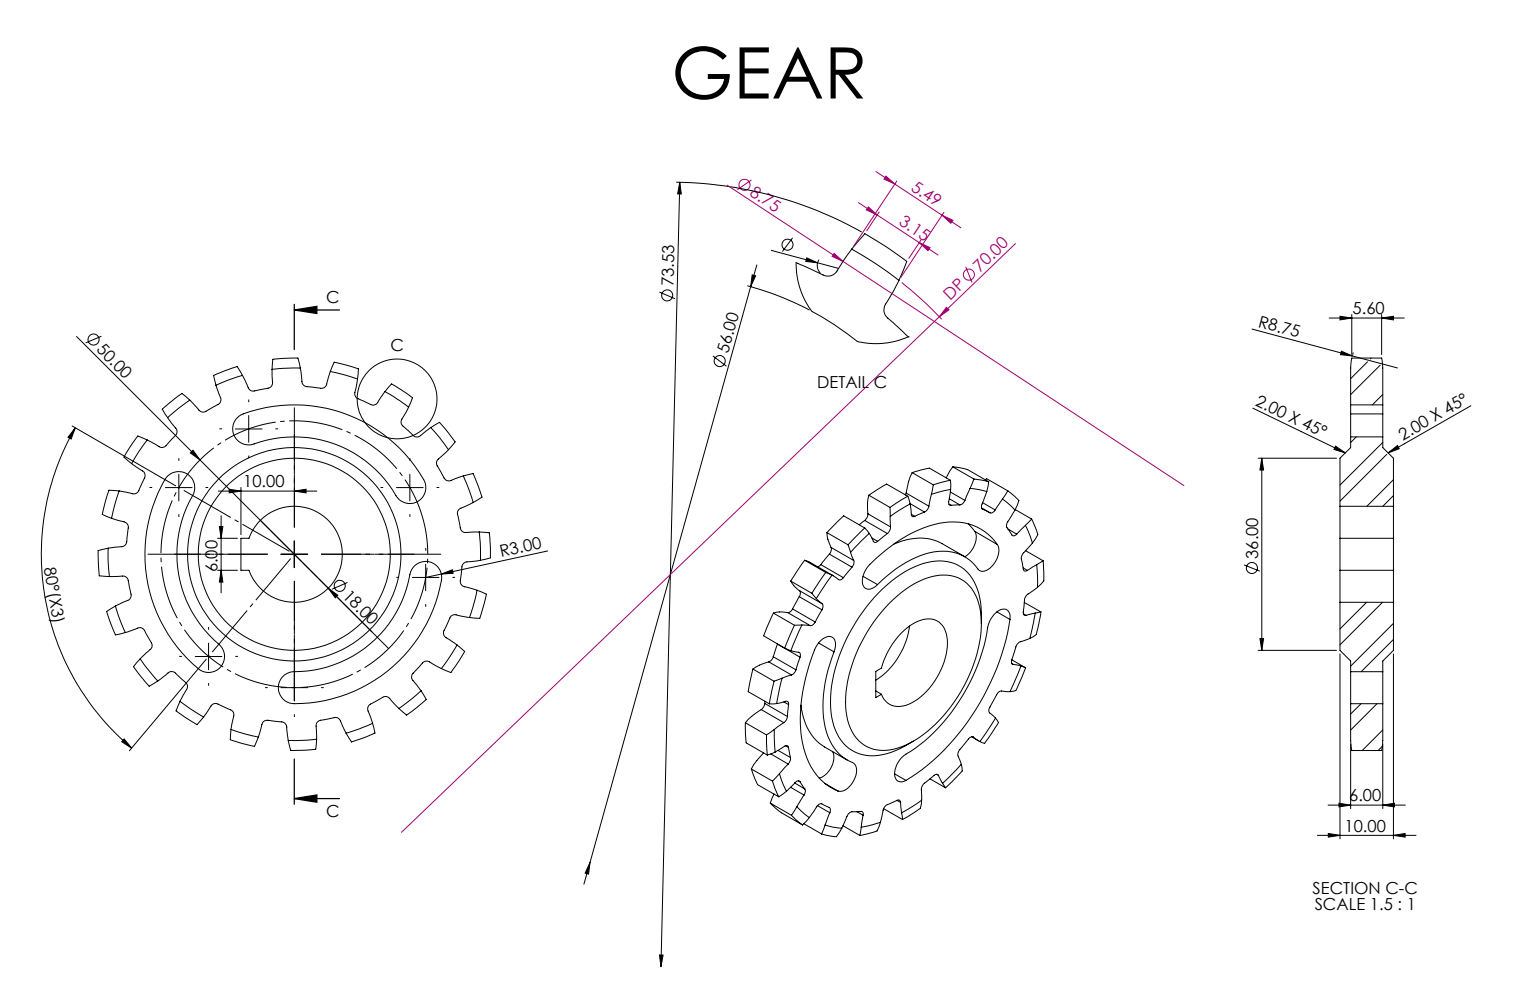
ISO-10303-21;
HEADER;
FILE_DESCRIPTION (('STEP AP214'),
    '1' );
FILE_NAME ('GEAR.step',
    '2026-10-24T00:51:42',
    ( '' ),
    ( '' ),
    'SwSTEP 2.0',
    'SolidWorks 2025',
    '' );
FILE_SCHEMA (( 'AUTOMOTIVE_DESIGN' ));
ENDSEC;

DATA;
#2=DIRECTION ( 'NONE',  ( -1.000000000000000000, 0.000000000000000000, 0.000000000000000000 ) ) ;
#3=EDGE_CURVE ( 'NONE', #16867, #19408, #6040, .T. ) ;
#4=CIRCLE ( 'NONE', #2943, 3.000000000000002665 ) ;
#5=ORIENTED_EDGE ( 'NONE', *, *, #17834, .T. ) ;
#10=CYLINDRICAL_SURFACE ( 'NONE', #2581, 1.000000000000000888 ) ;
#12=DIRECTION ( 'NONE',  ( -6.505213034913038160E-19, -3.903127820947822896E-18, -1.000000000000000000 ) ) ;
#23=ORIENTED_EDGE ( 'NONE', *, *, #6487, .T. ) ;
#24=DIRECTION ( 'NONE',  ( -6.505213034913038160E-19, -3.903127820947822896E-18, -1.000000000000000000 ) ) ;
#29=CARTESIAN_POINT ( 'NONE',  ( -36.39375341857508062, -7.980461308160102796, -6.999999999999985789 ) ) ;
#31=VERTEX_POINT ( 'NONE', #2518 ) ;
#35=ORIENTED_EDGE ( 'NONE', *, *, #15224, .F. ) ;
#41=DIRECTION ( 'NONE',  ( 6.505213034913038160E-19, 3.903127820947822896E-18, 1.000000000000000000 ) ) ;
#43=VERTEX_POINT ( 'NONE', #2740 ) ;
#45=ORIENTED_EDGE ( 'NONE', *, *, #21489, .F. ) ;
#48=DIRECTION ( 'NONE',  ( -1.000000000000000000, -1.208970125616063644E-17, 0.000000000000000000 ) ) ;
#49=ADVANCED_FACE ( 'NONE', ( #14857 ), #21880, .F. ) ;
#61=CARTESIAN_POINT ( 'NONE',  ( -24.43377932785584505, 26.64693883069154623, -2.933296326616394278 ) ) ;
#66=VERTEX_POINT ( 'NONE', #2856 ) ;
#68=CARTESIAN_POINT ( 'NONE',  ( -6.742883674876493316, -34.24928931925791176, -2.999999999999975131 ) ) ;
#69=EDGE_CURVE ( 'NONE', #16039, #14303, #1275, .T. ) ;
#72=DIRECTION ( 'NONE',  ( -1.000000000000000000, 0.000000000000000000, 0.000000000000000000 ) ) ;
#73=EDGE_CURVE ( 'NONE', #8231, #15027, #14429, .T. ) ;
#75=CARTESIAN_POINT ( 'NONE',  ( -21.65063509461097269, 12.49999999999990052, -5.000000000000004441 ) ) ;
#79=ADVANCED_FACE ( 'NONE', ( #15536 ), #15524, .T. ) ;
#80=ORIENTED_EDGE ( 'NONE', *, *, #1374, .F. ) ;
#81=ORIENTED_EDGE ( 'NONE', *, *, #16043, .F. ) ;
#85=CIRCLE ( 'NONE', #13966, 31.50000000000000711 ) ;
#94=CARTESIAN_POINT ( 'NONE',  ( 2.775557561562891351E-14, -2.775557561562891351E-14, 2.999999999999999112 ) ) ;
#100=CARTESIAN_POINT ( 'NONE',  ( -22.28024240313497728, -22.26748298433262008, 3.000000000000023537 ) ) ;
#101=CARTESIAN_POINT ( 'NONE',  ( 27.01645732367885699, 17.86915608785655252, -2.999999999999971578 ) ) ;
#102=AXIS2_PLACEMENT_3D ( 'NONE', #16431, #14697, #2342 ) ;
#103=EDGE_CURVE ( 'NONE', #20053, #16550, #22141, .T. ) ;
#104=VERTEX_POINT ( 'NONE', #2968 ) ;
#109=AXIS2_PLACEMENT_3D ( 'NONE', #8322, #11535, #18749 ) ;
#111=B_SPLINE_CURVE_WITH_KNOTS ( 'NONE', 3,
 ( #17365, #18873, #3301, #3063 ),
 .UNSPECIFIED., .F., .F.,
 ( 4, 4 ),
 ( 0.001893031756885769868, 0.003808480026564024790 ),
 .UNSPECIFIED. ) ;
#115=ORIENTED_EDGE ( 'NONE', *, *, #21368, .T. ) ;
#116=DIRECTION ( 'NONE',  ( 6.505213034913038160E-19, 3.903127820947822896E-18, 1.000000000000000000 ) ) ;
#119=DIRECTION ( 'NONE',  ( -6.505213034913038160E-19, -3.903127820947822896E-18, -1.000000000000000000 ) ) ;
#127=CARTESIAN_POINT ( 'NONE',  ( 4.177897941877304788, -34.13396246814587442, -2.999999999999999112 ) ) ;
#128=CARTESIAN_POINT ( 'NONE',  ( -31.11077005834418685, 4.936596639065066405, 2.999999999999995559 ) ) ;
#129=AXIS2_PLACEMENT_3D ( 'NONE', #9904, #8084, #22058 ) ;
#132=ORIENTED_EDGE ( 'NONE', *, *, #8958, .T. ) ;
#143=ORIENTED_EDGE ( 'NONE', *, *, #2467, .F. ) ;
#144=DIRECTION ( 'NONE',  ( 6.505213034913038160E-19, 3.903127820947822896E-18, 1.000000000000000000 ) ) ;
#148=ORIENTED_EDGE ( 'NONE', *, *, #5497, .F. ) ;
#161=ORIENTED_EDGE ( 'NONE', *, *, #622, .T. ) ;
#162=ORIENTED_EDGE ( 'NONE', *, *, #20424, .T. ) ;
#163=EDGE_CURVE ( 'NONE', #12184, #10164, #18107, .T. ) ;
#165=CARTESIAN_POINT ( 'NONE',  ( -32.75570538720762670, 15.02862401740784293, -2.999999999999995559 ) ) ;
#167=CARTESIAN_POINT ( 'NONE',  ( 3.330669073875469621E-13, -1.110223024625156540E-13, -2.999999999999971578 ) ) ;
#173=AXIS2_PLACEMENT_3D ( 'NONE', #16930, #17152, #13241 ) ;
#175=CARTESIAN_POINT ( 'NONE',  ( 2.220446049250313081E-13, 2.775557561562891351E-14, -2.800654218530485018 ) ) ;
#182=EDGE_CURVE ( 'NONE', #4097, #21371, #18465, .T. ) ;
#188=ORIENTED_EDGE ( 'NONE', *, *, #1082, .F. ) ;
#192=EDGE_LOOP ( 'NONE', ( #22045, #625, #16460, #5308 ) ) ;
#195=DIRECTION ( 'NONE',  ( 6.505213034913038160E-19, 3.903127820947822896E-18, 1.000000000000000000 ) ) ;
#203=AXIS2_PLACEMENT_3D ( 'NONE', #6824, #20803, #5115 ) ;
#204=ORIENTED_EDGE ( 'NONE', *, *, #20103, .T. ) ;
#206=CARTESIAN_POINT ( 'NONE',  ( -11.35354668330701422, -30.33632613426187774, 2.999999999999999112 ) ) ;
#209=CARTESIAN_POINT ( 'NONE',  ( -26.64365646977275048, -17.09029715894938661, -6.999999999999950262 ) ) ;
#211=CIRCLE ( 'NONE', #1322, 34.90673715956759082 ) ;
#214=DIRECTION ( 'NONE',  ( 6.505213034913038160E-19, 3.903127820947822896E-18, 1.000000000000000000 ) ) ;
#217=AXIS2_PLACEMENT_3D ( 'NONE', #4678, #12107, #11654 ) ;
#218=EDGE_CURVE ( 'NONE', #13519, #1842, #5991, .T. ) ;
#228=CARTESIAN_POINT ( 'NONE',  ( 11.93772187171674126, 33.46652738560661788, -3.000000000000018208 ) ) ;
#230=DIRECTION ( 'NONE',  ( 1.000000000000000000, 0.000000000000000000, 0.000000000000000000 ) ) ;
#236=FACE_OUTER_BOUND ( 'NONE', #19875, .T. ) ;
#237=ORIENTED_EDGE ( 'NONE', *, *, #15109, .F. ) ;
#238=DIRECTION ( 'NONE',  ( -1.000000000000000000, 0.000000000000000000, 0.000000000000000000 ) ) ;
#247=ORIENTED_EDGE ( 'NONE', *, *, #15444, .T. ) ;
#251=EDGE_CURVE ( 'NONE', #17561, #8959, #16232, .T. ) ;
#258=DIRECTION ( 'NONE',  ( -1.000000000000000000, -1.208970125616081209E-17, 0.000000000000000000 ) ) ;
#260=VERTEX_POINT ( 'NONE', #22683 ) ;
#263=DIRECTION ( 'NONE',  ( 1.000000000000000000, 0.000000000000000000, 0.000000000000000000 ) ) ;
#271=CARTESIAN_POINT ( 'NONE',  ( -12.00937115242646591, -34.74700806321101254, 2.800654218530512551 ) ) ;
#275=CARTESIAN_POINT ( 'NONE',  ( 17.79229176513301525, 31.47226199422865278, -2.933296326616372074 ) ) ;
#278=CARTESIAN_POINT ( 'NONE',  ( -25.58633464742629471, -23.74488952252781715, -2.999999999999975131 ) ) ;
#281=ORIENTED_EDGE ( 'NONE', *, *, #17376, .F. ) ;
#290=DIRECTION ( 'NONE',  ( 1.000000000000000000, 0.000000000000000000, 0.000000000000000000 ) ) ;
#294=CIRCLE ( 'NONE', #3228, 34.90673715956759082 ) ;
#295=VERTEX_POINT ( 'NONE', #13926 ) ;
#299=FACE_OUTER_BOUND ( 'NONE', #1043, .T. ) ;
#302=FACE_OUTER_BOUND ( 'NONE', #6391, .T. ) ;
#303=EDGE_CURVE ( 'NONE', #11367, #19446, #9654, .T. ) ;
#304=VECTOR ( 'NONE', #3939, 1000.000000000000000 ) ;
#309=AXIS2_PLACEMENT_3D ( 'NONE', #21426, #5731, #12703 ) ;
#312=VERTEX_POINT ( 'NONE', #7642 ) ;
#315=AXIS2_PLACEMENT_3D ( 'NONE', #10190, #17183, #1262 ) ;
#318=CARTESIAN_POINT ( 'NONE',  ( -26.50842683089743446, 24.41514043009193458, -2.999999999999975131 ) ) ;
#320=EDGE_CURVE ( 'NONE', #13797, #13818, #18394, .T. ) ;
#326=EDGE_LOOP ( 'NONE', ( #11952, #8295, #15497, #872 ) ) ;
#327=CARTESIAN_POINT ( 'NONE',  ( 5.551115123125782702E-14, -1.387778780781445676E-13, -5.749999999999949374 ) ) ;
#331=EDGE_CURVE ( 'NONE', #8378, #6859, #4945, .T. ) ;
#332=DIRECTION ( 'NONE',  ( 6.505213034913038160E-19, 3.903127820947822896E-18, 1.000000000000000000 ) ) ;
#333=ORIENTED_EDGE ( 'NONE', *, *, #2752, .T. ) ;
#335=DIRECTION ( 'NONE',  ( 6.505213034913038160E-19, 3.903127820947822896E-18, 1.000000000000000000 ) ) ;
#338=ORIENTED_EDGE ( 'NONE', *, *, #3032, .F. ) ;
#344=ADVANCED_FACE ( 'NONE', ( #7407, #531 ), #16341, .T. ) ;
#345=DIRECTION ( 'NONE',  ( 6.505213034913038160E-19, 3.903127820947822896E-18, 1.000000000000000000 ) ) ;
#346=ORIENTED_EDGE ( 'NONE', *, *, #17247, .F. ) ;
#352=DIRECTION ( 'NONE',  ( 1.000000000000000000, 0.000000000000000000, 0.000000000000000000 ) ) ;
#361=DIRECTION ( 'NONE',  ( -1.000000000000000000, -1.208970125616060717E-17, 0.000000000000000000 ) ) ;
#363=CIRCLE ( 'NONE', #12085, 1.000000000000000888 ) ;
#365=ORIENTED_EDGE ( 'NONE', *, *, #6652, .F. ) ;
#366=B_SPLINE_CURVE_WITH_KNOTS ( 'NONE', 3,
 ( #12902, #16119, #9147, #665 ),
 .UNSPECIFIED., .F., .F.,
 ( 4, 4 ),
 ( 0.001893031756885595529, 0.003808480026563915502 ),
 .UNSPECIFIED. ) ;
#372=AXIS2_PLACEMENT_3D ( 'NONE', #19827, #18095, #3326 ) ;
#375=ORIENTED_EDGE ( 'NONE', *, *, #11869, .T. ) ;
#376=DIRECTION ( 'NONE',  ( 1.000000000000000000, 0.000000000000000000, 0.000000000000000000 ) ) ;
#377=DIRECTION ( 'NONE',  ( 6.505213034913038160E-19, 3.903127820947822896E-18, 1.000000000000000000 ) ) ;
#378=ORIENTED_EDGE ( 'NONE', *, *, #15742, .T. ) ;
#381=CARTESIAN_POINT ( 'NONE',  ( 21.69517388068236841, 28.13960001536964128, -3.000000000000001776 ) ) ;
#382=DIRECTION ( 'NONE',  ( -6.505213034913038160E-19, -3.903127820947822896E-18, -1.000000000000000000 ) ) ;
#384=VERTEX_POINT ( 'NONE', #9359 ) ;
#396=ORIENTED_EDGE ( 'NONE', *, *, #11487, .T. ) ;
#399=ORIENTED_EDGE ( 'NONE', *, *, #73, .F. ) ;
#402=CARTESIAN_POINT ( 'NONE',  ( -35.79662727779878395, 4.171001175319294596, 3.000000000000006217 ) ) ;
#406=VECTOR ( 'NONE', #10198, 1000.000000000000000 ) ;
#410=LINE ( 'NONE', #7295, #19704 ) ;
#411=CARTESIAN_POINT ( 'NONE',  ( 2.775557561562891351E-14, 2.775557561562891351E-14, 5.750000000000001776 ) ) ;
#415=DIRECTION ( 'NONE',  ( 1.000000000000000000, 0.000000000000000000, 0.000000000000000000 ) ) ;
#417=B_SPLINE_CURVE_WITH_KNOTS ( 'NONE', 3,
 ( #9345, #17934, #21264, #14708 ),
 .UNSPECIFIED., .F., .F.,
 ( 4, 4 ),
 ( 9.545285770746368752E-07, 0.001900595205834774504 ),
 .UNSPECIFIED. ) ;
#427=LINE ( 'NONE', #14393, #10875 ) ;
#429=FACE_OUTER_BOUND ( 'NONE', #19761, .T. ) ;
#430=ADVANCED_FACE ( 'NONE', ( #15166 ), #13332, .T. ) ;
#443=EDGE_CURVE ( 'NONE', #2350, #18209, #20357, .T. ) ;
#444=ORIENTED_EDGE ( 'NONE', *, *, #19808, .F. ) ;
#445=CARTESIAN_POINT ( 'NONE',  ( -15.12081897056664914, 33.51030287062364721, -2.800654218530457484 ) ) ;
#446=ADVANCED_FACE ( 'NONE', ( #9810 ), #21783, .T. ) ;
#447=ORIENTED_EDGE ( 'NONE', *, *, #13329, .T. ) ;
#448=CARTESIAN_POINT ( 'NONE',  ( -4.170748987303213084, 34.65667543218822999, 3.000000000000002665 ) ) ;
#450=FACE_OUTER_BOUND ( 'NONE', #22695, .T. ) ;
#456=CARTESIAN_POINT ( 'NONE',  ( 2.775557561562891351E-14, -2.775557561562891351E-14, 2.999999999999999112 ) ) ;
#458=AXIS2_PLACEMENT_3D ( 'NONE', #18438, #22003, #1140 ) ;
#461=CARTESIAN_POINT ( 'NONE',  ( 7.463862311151453710, 35.99819890246943999, -2.800654218530457484 ) ) ;
#463=B_SPLINE_CURVE_WITH_KNOTS ( 'NONE', 3,
 ( #3611, #20792, #8757, #8523 ),
 .UNSPECIFIED., .F., .F.,
 ( 4, 4 ),
 ( 9.715086409175039034E-07, 0.001929643240672277446 ),
 .UNSPECIFIED. ) ;
#467=CARTESIAN_POINT ( 'NONE',  ( 31.21605069118074738, 8.646032897228984382, 2.999999999999995559 ) ) ;
#473=EDGE_LOOP ( 'NONE', ( #18170, #2329, #19189, #6844 ) ) ;
#481=CARTESIAN_POINT ( 'NONE',  ( 2.775557561562891351E-14, -2.775557561562891351E-14, 2.999999999999999112 ) ) ;
#483=CARTESIAN_POINT ( 'NONE',  ( -31.92986134326225667, 18.22261011550274645, 2.800654218530509443 ) ) ;
#489=ORIENTED_EDGE ( 'NONE', *, *, #9326, .F. ) ;
#492=DIRECTION ( 'NONE',  ( -1.000000000000000000, -1.052817288873011806E-14, 0.000000000000000000 ) ) ;
#502=AXIS2_PLACEMENT_3D ( 'NONE', #8254, #6205, #22245 ) ;
#505=ORIENTED_EDGE ( 'NONE', *, *, #18677, .F. ) ;
#509=ORIENTED_EDGE ( 'NONE', *, *, #13212, .T. ) ;
#519=EDGE_CURVE ( 'NONE', #5408, #3873, #7462, .T. ) ;
#520=EDGE_CURVE ( 'NONE', #4189, #4363, #18750, .T. ) ;
#525=DIRECTION ( 'NONE',  ( -1.000000000000000000, 0.000000000000000000, 0.000000000000000000 ) ) ;
#527=EDGE_CURVE ( 'NONE', #21131, #15970, #924, .T. ) ;
#531=FACE_OUTER_BOUND ( 'NONE', #18877, .T. ) ;
#541=AXIS2_PLACEMENT_3D ( 'NONE', #5026, #15537, #8566 ) ;
#556=PLANE ( 'NONE',  #2500 ) ;
#557=CIRCLE ( 'NONE', #3135, 31.50000000000000711 ) ;
#559=DIRECTION ( 'NONE',  ( 1.000000000000000000, 0.000000000000000000, 0.000000000000000000 ) ) ;
#561=EDGE_CURVE ( 'NONE', #19756, #19564, #12445, .T. ) ;
#571=CYLINDRICAL_SURFACE ( 'NONE', #12438, 36.76383501243555685 ) ;
#573=VERTEX_POINT ( 'NONE', #3286 ) ;
#581=DIRECTION ( 'NONE',  ( -6.505213034913038160E-19, -3.903127820947822896E-18, -1.000000000000000000 ) ) ;
#583=DIRECTION ( 'NONE',  ( 6.505213034913038160E-19, 3.903127820947822896E-18, 1.000000000000000000 ) ) ;
#584=DIRECTION ( 'NONE',  ( 1.000000000000000000, 0.000000000000000000, 0.000000000000000000 ) ) ;
#586=VERTEX_POINT ( 'NONE', #3393 ) ;
#587=DIRECTION ( 'NONE',  ( 1.000000000000000000, 0.000000000000000000, 0.000000000000000000 ) ) ;
#589=AXIS2_PLACEMENT_3D ( 'NONE', #14454, #144, #14110 ) ;
#591=CIRCLE ( 'NONE', #19618, 34.90673715956759082 ) ;
#600=CARTESIAN_POINT ( 'NONE',  ( 32.09841355225995585, -5.093313992686393732, -2.999999999999971578 ) ) ;
#601=DIRECTION ( 'NONE',  ( -6.505213034913038160E-19, -3.903127820947822896E-18, -1.000000000000000000 ) ) ;
#603=ORIENTED_EDGE ( 'NONE', *, *, #21489, .T. ) ;
#611=ORIENTED_EDGE ( 'NONE', *, *, #4266, .F. ) ;
#612=EDGE_CURVE ( 'NONE', #4064, #19773, #10257, .T. ) ;
#618=ORIENTED_EDGE ( 'NONE', *, *, #4093, .F. ) ;
#622=EDGE_CURVE ( 'NONE', #14783, #19446, #2359, .T. ) ;
#625=ORIENTED_EDGE ( 'NONE', *, *, #14576, .T. ) ;
#632=ORIENTED_EDGE ( 'NONE', *, *, #6395, .T. ) ;
#633=CARTESIAN_POINT ( 'NONE',  ( 21.00948735876884044, 24.79619811426203668, -6.999999999999950262 ) ) ;
#638=EDGE_LOOP ( 'NONE', ( #7057, #3498, #13428, #19774 ) ) ;
#648=AXIS2_PLACEMENT_3D ( 'NONE', #22157, #18941, #22389 ) ;
#649=DIRECTION ( 'NONE',  ( 1.000000000000000000, 0.000000000000000000, 0.000000000000000000 ) ) ;
#650=EDGE_CURVE ( 'NONE', #2517, #14456, #15130, .T. ) ;
#655=ADVANCED_FACE ( 'NONE', ( #1789 ), #15745, .T. ) ;
#657=EDGE_LOOP ( 'NONE', ( #17524, #9089, #7383, #7095 ) ) ;
#660=AXIS2_PLACEMENT_3D ( 'NONE', #764, #11299, #10833 ) ;
#662=FACE_OUTER_BOUND ( 'NONE', #3144, .T. ) ;
#665=CARTESIAN_POINT ( 'NONE',  ( -10.70799354677358295, 35.16985127952384715, -2.800654218530457484 ) ) ;
#667=VECTOR ( 'NONE', #15836, 1000.000000000000000 ) ;
#673=DIRECTION ( 'NONE',  ( -6.505213034913038160E-19, -3.903127820947822896E-18, -1.000000000000000000 ) ) ;
#683=AXIS2_PLACEMENT_3D ( 'NONE', #20759, #3350, #19155 ) ;
#684=ORIENTED_EDGE ( 'NONE', *, *, #8709, .F. ) ;
#686=LINE ( 'NONE', #5725, #14759 ) ;
#687=CIRCLE ( 'NONE', #13469, 19.11328065563150957 ) ;
#688=EDGE_CURVE ( 'NONE', #6587, #2221, #21014, .T. ) ;
#689=CARTESIAN_POINT ( 'NONE',  ( -4.153395668489446635, 35.29097153256767427, -3.000000000000005773 ) ) ;
#691=VERTEX_POINT ( 'NONE', #19537 ) ;
#700=CARTESIAN_POINT ( 'NONE',  ( 2.220446049250313081E-13, -8.326672684688674053E-14, 2.800654218530498785 ) ) ;
#706=AXIS2_PLACEMENT_3D ( 'NONE', #726, #7708, #376 ) ;
#710=ADVANCED_FACE ( 'NONE', ( #9559 ), #16194, .F. ) ;
#719=ORIENTED_EDGE ( 'NONE', *, *, #14828, .T. ) ;
#721=DIRECTION ( 'NONE',  ( -1.000000000000000000, -1.208970125616046080E-17, 6.505213034913038160E-19 ) ) ;
#726=CARTESIAN_POINT ( 'NONE',  ( -36.39375341857506641, -7.980461308160019307, 2.999999999999995559 ) ) ;
#728=VERTEX_POINT ( 'NONE', #12980 ) ;
#735=CARTESIAN_POINT ( 'NONE',  ( 3.330669073875469621E-13, -1.110223024625156540E-13, -2.999999999999971578 ) ) ;
#739=DIRECTION ( 'NONE',  ( 6.505213034913038160E-19, 3.903127820947822896E-18, 1.000000000000000000 ) ) ;
#741=ORIENTED_EDGE ( 'NONE', *, *, #20768, .T. ) ;
#743=DIRECTION ( 'NONE',  ( -1.000000000000000000, 0.000000000000000000, 0.000000000000000000 ) ) ;
#744=LINE ( 'NONE', #7724, #8894 ) ;
#746=AXIS2_PLACEMENT_3D ( 'NONE', #2751, #20166, #1139 ) ;
#749=ORIENTED_EDGE ( 'NONE', *, *, #19224, .T. ) ;
#750=ORIENTED_EDGE ( 'NONE', *, *, #2861, .F. ) ;
#754=ORIENTED_EDGE ( 'NONE', *, *, #3, .T. ) ;
#755=CARTESIAN_POINT ( 'NONE',  ( -30.57187188083515750, -7.711478842616581453, -7.000000000000006217 ) ) ;
#756=DIRECTION ( 'NONE',  ( -1.000000000000000000, -1.208970125616060717E-17, 0.000000000000000000 ) ) ;
#758=ORIENTED_EDGE ( 'NONE', *, *, #14920, .T. ) ;
#763=LINE ( 'NONE', #21503, #19035 ) ;
#764=CARTESIAN_POINT ( 'NONE',  ( 2.775557561562891351E-14, -2.775557561562891351E-14, 2.999999999999999112 ) ) ;
#766=DIRECTION ( 'NONE',  ( 6.505213034913038160E-19, 3.903127820947822896E-18, 1.000000000000000000 ) ) ;
#767=VERTEX_POINT ( 'NONE', #11155 ) ;
#768=VERTEX_POINT ( 'NONE', #14807 ) ;
#781=CARTESIAN_POINT ( 'NONE',  ( 3.330669073875469621E-13, -1.110223024625156540E-13, -2.999999999999971578 ) ) ;
#784=DIRECTION ( 'NONE',  ( 6.505213034913038160E-19, 3.903127820947822896E-18, 1.000000000000000000 ) ) ;
#794=EDGE_CURVE ( 'NONE', #10901, #12610, #2063, .T. ) ;
#795=ORIENTED_EDGE ( 'NONE', *, *, #10962, .F. ) ;
#801=CARTESIAN_POINT ( 'NONE',  ( -31.41239365194187272, 2.347663744114131035, -2.999999999999999112 ) ) ;
#803=DIRECTION ( 'NONE',  ( 1.000000000000000000, 0.000000000000000000, 0.000000000000000000 ) ) ;
#804=DIRECTION ( 'NONE',  ( -6.505213034913038160E-19, -3.903127820947822896E-18, -1.000000000000000000 ) ) ;
#808=CARTESIAN_POINT ( 'NONE',  ( -32.09841355225989901, 5.093313992686310243, -2.999999999999971578 ) ) ;
#811=DIRECTION ( 'NONE',  ( 6.505213034913038160E-19, 3.903127820947822896E-18, 1.000000000000000000 ) ) ;
#817=VERTEX_POINT ( 'NONE', #7327 ) ;
#820=CARTESIAN_POINT ( 'NONE',  ( 10.70799354677390269, -35.16985127952376899, -1.999999999999977573 ) ) ;
#822=AXIS2_PLACEMENT_3D ( 'NONE', #1588, #15211, #10392 ) ;
#824=DIRECTION ( 'NONE',  ( -1.000000000000000000, -1.208970125616062874E-17, 0.000000000000000000 ) ) ;
#827=ORIENTED_EDGE ( 'NONE', *, *, #19139, .F. ) ;
#829=FACE_OUTER_BOUND ( 'NONE', #20164, .T. ) ;
#833=DIRECTION ( 'NONE',  ( 6.505213034913038160E-19, 3.903127820947822896E-18, 1.000000000000000000 ) ) ;
#835=ORIENTED_EDGE ( 'NONE', *, *, #6395, .F. ) ;
#836=CARTESIAN_POINT ( 'NONE',  ( 36.75746821813308429, -0.6841746959067585010, 2.800654218530485018 ) ) ;
#838=EDGE_LOOP ( 'NONE', ( #3738, #12394, #3480, #9059 ) ) ;
#842=EDGE_LOOP ( 'NONE', ( #12632, #21482, #12314, #5111 ) ) ;
#845=DIRECTION ( 'NONE',  ( -1.000000000000000000, 0.000000000000000000, 0.000000000000000000 ) ) ;
#849=ORIENTED_EDGE ( 'NONE', *, *, #20424, .F. ) ;
#852=ORIENTED_EDGE ( 'NONE', *, *, #561, .T. ) ;
#854=DIRECTION ( 'NONE',  ( 6.505213034913038160E-19, 3.903127820947822896E-18, 1.000000000000000000 ) ) ;
#858=LINE ( 'NONE', #977, #13833 ) ;
#859=DIRECTION ( 'NONE',  ( -1.000000000000000000, 0.000000000000000000, 0.000000000000000000 ) ) ;
#863=DIRECTION ( 'NONE',  ( -6.505213034913038160E-19, -3.903127820947822896E-18, -1.000000000000000000 ) ) ;
#870=CARTESIAN_POINT ( 'NONE',  ( 8.646032897229400049, -31.21605069118077580, -6.999999999999950262 ) ) ;
#872=ORIENTED_EDGE ( 'NONE', *, *, #16600, .F. ) ;
#873=AXIS2_PLACEMENT_3D ( 'NONE', #3321, #3426, #13829 ) ;
#875=AXIS2_PLACEMENT_3D ( 'NONE', #12799, #6284, #13239 ) ;
#877=VERTEX_POINT ( 'NONE', #17322 ) ;
#885=DIRECTION ( 'NONE',  ( -1.000000000000000000, -1.208970125616063644E-17, 0.000000000000000000 ) ) ;
#890=CYLINDRICAL_SURFACE ( 'NONE', #9031, 1.000000000000000888 ) ;
#892=AXIS2_PLACEMENT_3D ( 'NONE', #18524, #18401, #17021 ) ;
#896=DIRECTION ( 'NONE',  ( 6.505213034913038160E-19, 3.903127820947822896E-18, 1.000000000000000000 ) ) ;
#898=ORIENTED_EDGE ( 'NONE', *, *, #4527, .T. ) ;
#899=CARTESIAN_POINT ( 'NONE',  ( 31.88709182564711142, -6.070730550691017413, 3.000000000000023537 ) ) ;
#901=CARTESIAN_POINT ( 'NONE',  ( 13.83143812983114707, -29.36548507648029016, -7.000000000000006217 ) ) ;
#905=CLOSED_SHELL ( 'NONE', ( #8563, #7076, #7929, #5678, #4465, #19150, #22576, #21458, #17712, #22222, #14782, #18419, #10391, #18239, #21785, #15928, #20178, #20226, #22233, #17927, #1863, #20395, #11837, #3599, #19443, #4692, #22628, #3299, #8649, #15514, #16721, #17259, #9019, #446, #1883, #17878, #8627, #15174, #20934, #10317, #17011, #430, #21730, #10433, #7354, #6426, #8274, #6528, #19882, #14280, #5310, #16856, #1353, #21124, #21999, #3977, #3481, #22065, #21190, #19028, #20680, #7463, #4335, #7078, #19523, #6625, #13775, #6600, #79, #8690, #20388, #3896, #2793, #13872, #15714, #5580, #19400, #10512, #8045, #12162, #18996, #15644, #12391, #11699, #344, #4559, #19376, #6148, #16346, #5545, #20631, #5202, #6959, #710, #4050, #13479, #14669, #14161, #1133, #2663, #18798, #4994, #14152, #14115, #16630, #13032, #3733, #10277, #7161, #2695, #3578, #1578, #655, #3354, #22650, #16686, #10847, #4861, #2677, #4727, #8678, #2175, #1764, #21366, #8230, #21822, #11023, #12771, #6554, #3602, #17130, #2598, #18208, #1841, #49, #6063, #16890, #12466, #17199, #15996, #21331, #8768, #2547, #8457, #22021, #6723, #20844, #21569, #17421, #5170, #16899, #4305, #11695, #22112, #22530, #9787, #17969, #8510, #5336, #13785, #10560, #17620, #13789, #1192, #21912, #3155, #19476, #2571, #13649, #2542, #11689, #2092, #18154, #9700, #18616, #5920, #14977, #20262, #5253, #5136, #6203, #12695, #20029, #16570, #21394, #16155, #16800, #21167, #16955, #6364, #9507, #16744, #8591, #19098, #1749, #6842, #21050, #6972, #17155, #19451, #8556 ) ) ;
#907=CARTESIAN_POINT ( 'NONE',  ( 34.74700806321121149, -12.00937115242670039, 2.800654218530512551 ) ) ;
#908=EDGE_CURVE ( 'NONE', #19435, #14442, #4561, .T. ) ;
#909=CARTESIAN_POINT ( 'NONE',  ( -4.025500340002513333, 36.54278193890309012, -2.800654218530457484 ) ) ;
#910=ORIENTED_EDGE ( 'NONE', *, *, #12200, .F. ) ;
#912=DIRECTION ( 'NONE',  ( 6.505213034913038160E-19, 3.903127820947822896E-18, 1.000000000000000000 ) ) ;
#920=CARTESIAN_POINT ( 'NONE',  ( 17.38064605515585725, 30.98879172160187068, 3.000000000000048850 ) ) ;
#921=EDGE_CURVE ( 'NONE', #10690, #11353, #1254, .T. ) ;
#924=CIRCLE ( 'NONE', #17694, 19.11328065563150957 ) ;
#928=VERTEX_POINT ( 'NONE', #1173 ) ;
#934=CIRCLE ( 'NONE', #6414, 36.76383501243555685 ) ;
#936=ORIENTED_EDGE ( 'NONE', *, *, #12946, .T. ) ;
#943=VERTEX_POINT ( 'NONE', #14908 ) ;
#945=CARTESIAN_POINT ( 'NONE',  ( 33.52953626616073279, 9.708269511265299911, -2.999999999999999112 ) ) ;
#953=ORIENTED_EDGE ( 'NONE', *, *, #3177, .F. ) ;
#955=AXIS2_PLACEMENT_3D ( 'NONE', #2451, #833, #9435 ) ;
#956=CARTESIAN_POINT ( 'NONE',  ( -21.05198877411806890, 30.13956425491229396, 2.800654218530481465 ) ) ;
#961=CARTESIAN_POINT ( 'NONE',  ( 22.15900668633799597, 29.33526866242094755, 2.800654218530481465 ) ) ;
#962=CARTESIAN_POINT ( 'NONE',  ( 2.775557561562891351E-14, 2.775557561562891351E-14, 5.750000000000001776 ) ) ;
#969=CIRCLE ( 'NONE', #14843, 1.000000000000000888 ) ;
#975=EDGE_CURVE ( 'NONE', #10281, #6403, #8168, .T. ) ;
#977=CARTESIAN_POINT ( 'NONE',  ( -33.51030287062356194, -15.12081897056691204, -2.000000000000005329 ) ) ;
#980=DIRECTION ( 'NONE',  ( -6.505213034913038160E-19, -3.903127820947822896E-18, -1.000000000000000000 ) ) ;
#986=CARTESIAN_POINT ( 'NONE',  ( -35.91964150878168027, -4.104665049622911788, -2.933296326616361416 ) ) ;
#995=FACE_OUTER_BOUND ( 'NONE', #22560, .T. ) ;
#1002=DIRECTION ( 'NONE',  ( 1.000000000000000000, 1.208970125616053475E-17, 0.000000000000000000 ) ) ;
#1010=DIRECTION ( 'NONE',  ( 1.000000000000000000, 1.208970125616053321E-17, 0.000000000000000000 ) ) ;
#1019=CARTESIAN_POINT ( 'NONE',  ( 37.07861450834818129, -3.656418565264468512, -6.999999999999999112 ) ) ;
#1020=EDGE_CURVE ( 'NONE', #18887, #21019, #14081, .T. ) ;
#1022=DIRECTION ( 'NONE',  ( 6.505213034913038160E-19, 3.903127820947822896E-18, 1.000000000000000000 ) ) ;
#1025=CIRCLE ( 'NONE', #15655, 31.50000000000001421 ) ;
#1028=VECTOR ( 'NONE', #21615, 1000.000000000000000 ) ;
#1029=DIRECTION ( 'NONE',  ( -1.000000000000000000, -1.208970125616060717E-17, 0.000000000000000000 ) ) ;
#1034=DIRECTION ( 'NONE',  ( -1.000000000000000000, -1.208970125616077665E-17, 0.000000000000000000 ) ) ;
#1041=B_SPLINE_CURVE_WITH_KNOTS ( 'NONE', 3,
 ( #15282, #19394, #22410, #15505 ),
 .UNSPECIFIED., .F., .F.,
 ( 4, 4 ),
 ( 0.001893031756885169004, 0.003808480026563660498 ),
 .UNSPECIFIED. ) ;
#1043=EDGE_LOOP ( 'NONE', ( #3805, #13880, #14516, #5311 ) ) ;
#1044=AXIS2_PLACEMENT_3D ( 'NONE', #4036, #2841, #6275 ) ;
#1046=DIRECTION ( 'NONE',  ( 6.505213034913038160E-19, 3.903127820947822896E-18, 1.000000000000000000 ) ) ;
#1047=AXIS2_PLACEMENT_3D ( 'NONE', #633, #15979, #290 ) ;
#1048=AXIS2_PLACEMENT_3D ( 'NONE', #20032, #4338, #1002 ) ;
#1050=ORIENTED_EDGE ( 'NONE', *, *, #320, .T. ) ;
#1051=EDGE_CURVE ( 'NONE', #1297, #18279, #13311, .T. ) ;
#1052=ORIENTED_EDGE ( 'NONE', *, *, #13195, .T. ) ;
#1060=CARTESIAN_POINT ( 'NONE',  ( -5.074925817841801745, 32.10132595304121850, -6.999999999999950262 ) ) ;
#1064=CIRCLE ( 'NONE', #7639, 36.76383501243555685 ) ;
#1066=EDGE_CURVE ( 'NONE', #22056, #12221, #10745, .T. ) ;
#1068=DIRECTION ( 'NONE',  ( 1.000000000000000000, 0.000000000000000000, 0.000000000000000000 ) ) ;
#1072=CARTESIAN_POINT ( 'NONE',  ( 29.36548507648026174, 13.83143812983086995, 3.000000000000023537 ) ) ;
#1073=ORIENTED_EDGE ( 'NONE', *, *, #4590, .T. ) ;
#1076=ORIENTED_EDGE ( 'NONE', *, *, #6843, .F. ) ;
#1080=EDGE_LOOP ( 'NONE', ( #4988, #8993, #12256, #12165, #18775, #10133 ) ) ;
#1081=DIRECTION ( 'NONE',  ( -1.000000000000000000, -1.208970125616081209E-17, 0.000000000000000000 ) ) ;
#1082=EDGE_CURVE ( 'NONE', #8936, #13925, #9174, .T. ) ;
#1086=ORIENTED_EDGE ( 'NONE', *, *, #5522, .F. ) ;
#1087=ORIENTED_EDGE ( 'NONE', *, *, #13548, .F. ) ;
#1088=VERTEX_POINT ( 'NONE', #16387 ) ;
#1089=VERTEX_POINT ( 'NONE', #12592 ) ;
#1093=DIRECTION ( 'NONE',  ( 6.505213034913038160E-19, 3.903127820947822896E-18, 1.000000000000000000 ) ) ;
#1103=EDGE_CURVE ( 'NONE', #4270, #21371, #16147, .T. ) ;
#1109=EDGE_LOOP ( 'NONE', ( #375, #3783, #3352, #21228, #19143, #12835 ) ) ;
#1110=CIRCLE ( 'NONE', #20504, 1.000000000000000888 ) ;
#1114=DIRECTION ( 'NONE',  ( 6.505213034913038160E-19, 3.903127820947822896E-18, 1.000000000000000000 ) ) ;
#1116=AXIS2_PLACEMENT_3D ( 'NONE', #1709, #13712, #16941 ) ;
#1118=DIRECTION ( 'NONE',  ( -1.000000000000000000, 0.000000000000000000, 0.000000000000000000 ) ) ;
#1128=DIRECTION ( 'NONE',  ( -6.505213034913038160E-19, -3.903127820947822896E-18, -1.000000000000000000 ) ) ;
#1129=CARTESIAN_POINT ( 'NONE',  ( 31.41239365194228839, -2.347663744114464102, -2.999999999999999112 ) ) ;
#1130=CARTESIAN_POINT ( 'NONE',  ( 34.64233806479157352, 10.34893680499398272, 2.932969818539056472 ) ) ;
#1133=ADVANCED_FACE ( 'NONE', ( #15921 ), #5617, .F. ) ;
#1139=DIRECTION ( 'NONE',  ( 1.000000000000000000, 0.000000000000000000, 0.000000000000000000 ) ) ;
#1140=DIRECTION ( 'NONE',  ( 1.000000000000000000, 0.000000000000000000, 0.000000000000000000 ) ) ;
#1141=CARTESIAN_POINT ( 'NONE',  ( 5.551115123125782702E-14, -1.387778780781445676E-13, -5.749999999999949374 ) ) ;
#1144=FACE_OUTER_BOUND ( 'NONE', #11608, .T. ) ;
#1152=CARTESIAN_POINT ( 'NONE',  ( 2.775557561562891351E-14, 2.775557561562891351E-14, 5.750000000000001776 ) ) ;
#1154=CIRCLE ( 'NONE', #13936, 19.11328065563152023 ) ;
#1156=ORIENTED_EDGE ( 'NONE', *, *, #12333, .T. ) ;
#1158=EDGE_LOOP ( 'NONE', ( #1280, #14441, #11642, #13027 ) ) ;
#1165=ORIENTED_EDGE ( 'NONE', *, *, #11487, .F. ) ;
#1169=CARTESIAN_POINT ( 'NONE',  ( -31.11359284679382498, -4.918774254216079278, -2.999999999999971578 ) ) ;
#1170=DIRECTION ( 'NONE',  ( -1.000000000000000000, 0.000000000000000000, 0.000000000000000000 ) ) ;
#1172=ORIENTED_EDGE ( 'NONE', *, *, #2942, .F. ) ;
#1173=CARTESIAN_POINT ( 'NONE',  ( -34.24928931925748543, 6.742883674876520850, -2.999999999999957367 ) ) ;
#1178=DIRECTION ( 'NONE',  ( -6.505213034913038160E-19, -3.903127820947822896E-18, -1.000000000000000000 ) ) ;
#1179=EDGE_CURVE ( 'NONE', #14813, #15106, #21665, .T. ) ;
#1183=EDGE_CURVE ( 'NONE', #15016, #19404, #7569, .T. ) ;
#1189=ORIENTED_EDGE ( 'NONE', *, *, #16482, .F. ) ;
#1192=ADVANCED_FACE ( 'NONE', ( #236 ), #10760, .T. ) ;
#1194=CYLINDRICAL_SURFACE ( 'NONE', #10169, 19.11328065563151668 ) ;
#1196=ORIENTED_EDGE ( 'NONE', *, *, #19405, .T. ) ;
#1199=ORIENTED_EDGE ( 'NONE', *, *, #1318, .F. ) ;
#1206=EDGE_CURVE ( 'NONE', #14456, #5141, #2188, .T. ) ;
#1213=LINE ( 'NONE', #6269, #13676 ) ;
#1219=FACE_OUTER_BOUND ( 'NONE', #18138, .T. ) ;
#1220=EDGE_LOOP ( 'NONE', ( #16663, #20723, #12377, #11901, #7553, #4761 ) ) ;
#1224=CARTESIAN_POINT ( 'NONE',  ( 19.59430950039317665, -28.88846368933348074, -2.999999999999999112 ) ) ;
#1229=ORIENTED_EDGE ( 'NONE', *, *, #6730, .F. ) ;
#1230=VECTOR ( 'NONE', #854, 1000.000000000000000 ) ;
#1236=ORIENTED_EDGE ( 'NONE', *, *, #4757, .T. ) ;
#1237=EDGE_CURVE ( 'NONE', #21534, #5255, #14095, .T. ) ;
#1238=ORIENTED_EDGE ( 'NONE', *, *, #7866, .T. ) ;
#1243=CARTESIAN_POINT ( 'NONE',  ( -14.93538271375417814, -34.13396246814587442, -6.999999999999950262 ) ) ;
#1244=TOROIDAL_SURFACE ( 'NONE', #873, 34.90673715956759082, 8.750000000000000000 ) ;
#1251=DIRECTION ( 'NONE',  ( -6.505213034913038160E-19, -3.903127820947822896E-18, -1.000000000000000000 ) ) ;
#1254=B_SPLINE_CURVE_WITH_KNOTS ( 'NONE', 3,
 ( #836, #7825, #22270, #16763 ),
 .UNSPECIFIED., .F., .F.,
 ( 4, 4 ),
 ( 9.715086431488502079E-07, 0.001929643240674611517 ),
 .UNSPECIFIED. ) ;
#1255=DIRECTION ( 'NONE',  ( 1.000000000000000000, 1.208970125616062874E-17, 0.000000000000000000 ) ) ;
#1256=CARTESIAN_POINT ( 'NONE',  ( -7.474202570535965151, 30.60042966911705165, 3.000000000000023537 ) ) ;
#1261=CARTESIAN_POINT ( 'NONE',  ( 2.220446049250313081E-13, -8.326672684688674053E-14, 2.800654218530498785 ) ) ;
#1262=DIRECTION ( 'NONE',  ( -1.000000000000000000, 0.000000000000000000, 0.000000000000000000 ) ) ;
#1263=VECTOR ( 'NONE', #7771, 1000.000000000000000 ) ;
#1266=B_SPLINE_CURVE_WITH_KNOTS ( 'NONE', 3,
 ( #10601, #3981, #8893, #7520 ),
 .UNSPECIFIED., .F., .F.,
 ( 4, 4 ),
 ( 0.001893031756885373267, 0.003808480026563830501 ),
 .UNSPECIFIED. ) ;
#1267=ORIENTED_EDGE ( 'NONE', *, *, #13329, .F. ) ;
#1271=CYLINDRICAL_SURFACE ( 'NONE', #19822, 1.000000000000000888 ) ;
#1275=CIRCLE ( 'NONE', #14789, 36.76383501243555685 ) ;
#1280=ORIENTED_EDGE ( 'NONE', *, *, #921, .F. ) ;
#1281=DIRECTION ( 'NONE',  ( -1.000000000000000000, 0.000000000000000000, 0.000000000000000000 ) ) ;
#1284=CARTESIAN_POINT ( 'NONE',  ( -28.45046755804880689, 15.62726112422596714, -2.999999999999999112 ) ) ;
#1288=ORIENTED_EDGE ( 'NONE', *, *, #21257, .T. ) ;
#1291=ORIENTED_EDGE ( 'NONE', *, *, #4150, .T. ) ;
#1293=DIRECTION ( 'NONE',  ( -1.000000000000000000, -1.788446540656407938E-15, 0.000000000000000000 ) ) ;
#1297=VERTEX_POINT ( 'NONE', #14988 ) ;
#1302=ORIENTED_EDGE ( 'NONE', *, *, #10885, .T. ) ;
#1303=DIRECTION ( 'NONE',  ( 1.000000000000000000, 0.000000000000000000, 0.000000000000000000 ) ) ;
#1304=DIRECTION ( 'NONE',  ( 6.505213034913038160E-19, 3.903127820947822896E-18, 1.000000000000000000 ) ) ;
#1306=ORIENTED_EDGE ( 'NONE', *, *, #1183, .F. ) ;
#1307=CARTESIAN_POINT ( 'NONE',  ( -29.75120097320039392, -20.55056392469606408, -2.932164912090505116 ) ) ;
#1309=ORIENTED_EDGE ( 'NONE', *, *, #20125, .F. ) ;
#1310=VECTOR ( 'NONE', #7238, 1000.000000000000000 ) ;
#1311=LINE ( 'NONE', #8305, #19049 ) ;
#1318=EDGE_CURVE ( 'NONE', #4146, #3268, #16945, .T. ) ;
#1319=LINE ( 'NONE', #19080, #8620 ) ;
#1322=AXIS2_PLACEMENT_3D ( 'NONE', #7206, #7552, #15901 ) ;
#1325=ORIENTED_EDGE ( 'NONE', *, *, #20988, .T. ) ;
#1328=ORIENTED_EDGE ( 'NONE', *, *, #519, .T. ) ;
#1332=CYLINDRICAL_SURFACE ( 'NONE', #21333, 22.00000000000000000 ) ;
#1336=CARTESIAN_POINT ( 'NONE',  ( 2.220446049250313081E-13, -2.498001805406602216E-13, -6.859353255829918616 ) ) ;
#1338=DIRECTION ( 'NONE',  ( 6.505213034913038160E-19, 3.903127820947822896E-18, 1.000000000000000000 ) ) ;
#1343=LINE ( 'NONE', #15307, #2031 ) ;
#1344=CIRCLE ( 'NONE', #21481, 0.9999999999999974465 ) ;
#1349=CARTESIAN_POINT ( 'NONE',  ( -1.423424233832348840, -32.35999952201584762, 3.000000000000002665 ) ) ;
#1353=ADVANCED_FACE ( 'NONE', ( #1144 ), #2535, .T. ) ;
#1354=ORIENTED_EDGE ( 'NONE', *, *, #11440, .T. ) ;
#1356=VECTOR ( 'NONE', #9848, 1000.000000000000000 ) ;
#1365=DIRECTION ( 'NONE',  ( 6.505213034913038160E-19, 3.903127820947822896E-18, 1.000000000000000000 ) ) ;
#1366=AXIS2_PLACEMENT_3D ( 'NONE', #3464, #14075, #10640 ) ;
#1368=VERTEX_POINT ( 'NONE', #9520 ) ;
#1370=AXIS2_PLACEMENT_3D ( 'NONE', #22005, #13158, #11571 ) ;
#1374=EDGE_CURVE ( 'NONE', #21043, #20280, #14319, .T. ) ;
#1378=DIRECTION ( 'NONE',  ( 6.505213034913038160E-19, 3.903127820947822896E-18, 1.000000000000000000 ) ) ;
#1379=CARTESIAN_POINT ( 'NONE',  ( 24.03323817228492132, -20.36304159388363644, 2.999999999999995559 ) ) ;
#1380=DIRECTION ( 'NONE',  ( -1.000000000000000000, -1.208970125616060717E-17, 0.000000000000000000 ) ) ;
#1387=ORIENTED_EDGE ( 'NONE', *, *, #1673, .T. ) ;
#1388=CARTESIAN_POINT ( 'NONE',  ( 14.67611967928938910, -31.67162468656004037, 2.999999999999999112 ) ) ;
#1391=CARTESIAN_POINT ( 'NONE',  ( -28.88846368933341324, -19.59430950039328678, 2.999999999999995559 ) ) ;
#1394=DIRECTION ( 'NONE',  ( 6.505213034913038160E-19, 3.903127820947822896E-18, 1.000000000000000000 ) ) ;
#1400=EDGE_CURVE ( 'NONE', #5811, #2517, #8137, .T. ) ;
#1402=LINE ( 'NONE', #8610, #11556 ) ;
#1405=AXIS2_PLACEMENT_3D ( 'NONE', #1465, #5570, #5468 ) ;
#1407=CARTESIAN_POINT ( 'NONE',  ( 21.05198877411829272, -30.13956425491240410, -2.800654218530457484 ) ) ;
#1408=DIRECTION ( 'NONE',  ( 1.000000000000000000, 0.000000000000000000, 0.000000000000000000 ) ) ;
#1410=ORIENTED_EDGE ( 'NONE', *, *, #4917, .F. ) ;
#1414=DIRECTION ( 'NONE',  ( 6.505213034913038160E-19, 3.903127820947822896E-18, 1.000000000000000000 ) ) ;
#1415=CARTESIAN_POINT ( 'NONE',  ( 0.8626474017861728294, 36.14481870267503894, 2.932969818539059137 ) ) ;
#1420=AXIS2_PLACEMENT_3D ( 'NONE', #20372, #8111, #1118 ) ;
#1434=VERTEX_POINT ( 'NONE', #8542 ) ;
#1435=LINE ( 'NONE', #12088, #8258 ) ;
#1437=CARTESIAN_POINT ( 'NONE',  ( 29.75120097320059642, 20.55056392469582249, -2.932164912090509556 ) ) ;
#1439=TOROIDAL_SURFACE ( 'NONE', #14213, 34.90673715956759082, 8.750000000000000000 ) ;
#1440=LINE ( 'NONE', #14853, #8918 ) ;
#1441=CIRCLE ( 'NONE', #7651, 19.11328065563151668 ) ;
#1442=CARTESIAN_POINT ( 'NONE',  ( 18.83615802559807051, -32.14641817400198676, -2.999999999999950706 ) ) ;
#1448=EDGE_CURVE ( 'NONE', #16878, #5871, #5205, .T. ) ;
#1451=LINE ( 'NONE', #20249, #16625 ) ;
#1453=TOROIDAL_SURFACE ( 'NONE', #18647, 34.90673715956759082, 8.750000000000000000 ) ;
#1461=DIRECTION ( 'NONE',  ( 6.505213034913038160E-19, 3.903127820947822896E-18, 1.000000000000000000 ) ) ;
#1462=ORIENTED_EDGE ( 'NONE', *, *, #22203, .T. ) ;
#1463=CARTESIAN_POINT ( 'NONE',  ( 29.14949368109903816, -11.93972437435561496, -6.999999999999999112 ) ) ;
#1465=CARTESIAN_POINT ( 'NONE',  ( 2.775557561562891351E-14, 2.775557561562891351E-14, 5.750000000000001776 ) ) ;
#1467=EDGE_CURVE ( 'NONE', #8376, #13932, #14012, .T. ) ;
#1472=EDGE_CURVE ( 'NONE', #1729, #5874, #13588, .T. ) ;
#1475=TOROIDAL_SURFACE ( 'NONE', #2955, 34.90673715956759082, 8.750000000000000000 ) ;
#1477=ORIENTED_EDGE ( 'NONE', *, *, #17589, .F. ) ;
#1483=CARTESIAN_POINT ( 'NONE',  ( -31.09841355225970005, 5.093313992686310243, 2.999999999999995559 ) ) ;
#1487=CARTESIAN_POINT ( 'NONE',  ( -28.95348479018568355, 14.76298474240497782, -2.999999999999999112 ) ) ;
#1489=LINE ( 'NONE', #13265, #7925 ) ;
#1491=EDGE_LOOP ( 'NONE', ( #5886, #13429, #17032, #22013, #13605, #1325 ) ) ;
#1493=EDGE_CURVE ( 'NONE', #19154, #7411, #3753, .T. ) ;
#1496=CARTESIAN_POINT ( 'NONE',  ( -36.54278193890292670, -4.025500340002762911, -1.999999999999977573 ) ) ;
#1498=SHAPE_DEFINITION_REPRESENTATION ( #16442, #18960 ) ;
#1499=EDGE_CURVE ( 'NONE', #11018, #12118, #6669, .T. ) ;
#1507=DIRECTION ( 'NONE',  ( -1.000000000000000000, -1.208970125616081209E-17, 0.000000000000000000 ) ) ;
#1508=VERTEX_POINT ( 'NONE', #1900 ) ;
#1510=CARTESIAN_POINT ( 'NONE',  ( -31.41173278719225337, -17.66631876130930578, -2.999999999999981792 ) ) ;
#1512=CARTESIAN_POINT ( 'NONE',  ( 4.104166344909097042, -35.92356703407504881, 2.932460736555814407 ) ) ;
#1513=DIRECTION ( 'NONE',  ( -1.000000000000000000, -1.208970125616083212E-17, 0.000000000000000000 ) ) ;
#1518=EDGE_CURVE ( 'NONE', #8421, #11018, #19211, .T. ) ;
#1521=DIRECTION ( 'NONE',  ( 1.000000000000000000, 0.000000000000000000, 0.000000000000000000 ) ) ;
#1529=ORIENTED_EDGE ( 'NONE', *, *, #2995, .T. ) ;
#1531=ORIENTED_EDGE ( 'NONE', *, *, #14736, .T. ) ;
#1533=ORIENTED_EDGE ( 'NONE', *, *, #11163, .F. ) ;
#1534=DIRECTION ( 'NONE',  ( -6.505213034913038160E-19, -3.903127820947822896E-18, -1.000000000000000000 ) ) ;
#1536=VECTOR ( 'NONE', #1251, 1000.000000000000000 ) ;
#1540=FACE_OUTER_BOUND ( 'NONE', #15792, .T. ) ;
#1547=FACE_OUTER_BOUND ( 'NONE', #14907, .T. ) ;
#1551=CARTESIAN_POINT ( 'NONE',  ( 10.01331137436180008, -34.09180625983483992, -2.999999999999996891 ) ) ;
#1553=EDGE_CURVE ( 'NONE', #2190, #14890, #85, .T. ) ;
#1554=ORIENTED_EDGE ( 'NONE', *, *, #11138, .F. ) ;
#1555=VERTEX_POINT ( 'NONE', #3516 ) ;
#1557=CARTESIAN_POINT ( 'NONE',  ( 2.220446049250313081E-13, -8.326672684688674053E-14, 2.800654218530498785 ) ) ;
#1562=AXIS2_PLACEMENT_3D ( 'NONE', #2038, #14391, #17621 ) ;
#1569=CIRCLE ( 'NONE', #12525, 19.11328065563151668 ) ;
#1573=ORIENTED_EDGE ( 'NONE', *, *, #1493, .T. ) ;
#1577=ORIENTED_EDGE ( 'NONE', *, *, #20768, .F. ) ;
#1578=ADVANCED_FACE ( 'NONE', ( #21038 ), #21605, .F. ) ;
#1584=CARTESIAN_POINT ( 'NONE',  ( 32.09841355226000559, -5.093313992686670844, 2.999999999999995559 ) ) ;
#1588=CARTESIAN_POINT ( 'NONE',  ( 22.97438720605751783, -22.98755168577440600, -2.999999999999995559 ) ) ;
#1591=CARTESIAN_POINT ( 'NONE',  ( 18.22261011550299514, 31.92986134326217140, -2.800654218530460593 ) ) ;
#1602=ORIENTED_EDGE ( 'NONE', *, *, #8075, .T. ) ;
#1603=CARTESIAN_POINT ( 'NONE',  ( 2.220446049250313081E-13, 2.775557561562891351E-14, -2.800654218530485018 ) ) ;
#1612=AXIS2_PLACEMENT_3D ( 'NONE', #18108, #14771, #16730 ) ;
#1614=CARTESIAN_POINT ( 'NONE',  ( 4.170748987303491084, -34.65667543218836499, -2.999999999999988898 ) ) ;
#1615=CYLINDRICAL_SURFACE ( 'NONE', #8464, 8.999999999999998224 ) ;
#1619=LINE ( 'NONE', #3234, #6176 ) ;
#1625=DIRECTION ( 'NONE',  ( 6.505213034913038160E-19, 3.903127820947822896E-18, 1.000000000000000000 ) ) ;
#1643=ORIENTED_EDGE ( 'NONE', *, *, #4636, .T. ) ;
#1644=EDGE_CURVE ( 'NONE', #6092, #9113, #22053, .T. ) ;
#1648=CARTESIAN_POINT ( 'NONE',  ( 0.000000000000000000, 0.000000000000000000, 0.000000000000000000 ) ) ;
#1652=DIRECTION ( 'NONE',  ( -1.000000000000000000, -1.208970125616044077E-17, 0.000000000000000000 ) ) ;
#1656=CARTESIAN_POINT ( 'NONE',  ( 11.93972437435558653, 29.14949368109881433, 2.999999999999995559 ) ) ;
#1657=CARTESIAN_POINT ( 'NONE',  ( 1.110223024625156540E-13, -5.551115123125782702E-14, -6.999999999999950262 ) ) ;
#1659=ORIENTED_EDGE ( 'NONE', *, *, #20988, .F. ) ;
#1673=EDGE_CURVE ( 'NONE', #16039, #2202, #2606, .T. ) ;
#1678=CYLINDRICAL_SURFACE ( 'NONE', #14726, 0.9999999999999974465 ) ;
#1679=CIRCLE ( 'NONE', #19987, 2.999999999999999112 ) ;
#1681=CARTESIAN_POINT ( 'NONE',  ( 21.66577056626872633, -3.820259908672546167, -2.999999999999971578 ) ) ;
#1686=CARTESIAN_POINT ( 'NONE',  ( -34.09574698892485856, -10.01544929272315088, 3.000000000000056399 ) ) ;
#1688=CARTESIAN_POINT ( 'NONE',  ( 1.110223024625156540E-13, -5.551115123125782702E-14, -6.999999999999950262 ) ) ;
#1697=DIRECTION ( 'NONE',  ( 1.000000000000000000, 0.000000000000000000, 0.000000000000000000 ) ) ;
#1703=ORIENTED_EDGE ( 'NONE', *, *, #17438, .T. ) ;
#1708=EDGE_CURVE ( 'NONE', #19434, #18082, #21683, .T. ) ;
#1709=CARTESIAN_POINT ( 'NONE',  ( 1.110223024625156540E-13, -5.551115123125782702E-14, -6.999999999999950262 ) ) ;
#1714=EDGE_CURVE ( 'NONE', #12526, #19349, #10771, .T. ) ;
#1715=AXIS2_PLACEMENT_3D ( 'NONE', #7984, #21973, #12889 ) ;
#1720=CARTESIAN_POINT ( 'NONE',  ( -36.54278193890294091, -4.025500340002652777, 2.800654218530481465 ) ) ;
#1721=ORIENTED_EDGE ( 'NONE', *, *, #14368, .F. ) ;
#1725=EDGE_CURVE ( 'NONE', #2966, #11042, #17270, .T. ) ;
#1729=VERTEX_POINT ( 'NONE', #18275 ) ;
#1734=CARTESIAN_POINT ( 'NONE',  ( 4.936596639065371050, 31.11077005834392395, -2.999999999999975131 ) ) ;
#1737=VERTEX_POINT ( 'NONE', #20454 ) ;
#1738=FACE_OUTER_BOUND ( 'NONE', #22008, .T. ) ;
#1742=CIRCLE ( 'NONE', #2089, 3.000000000000002665 ) ;
#1748=CARTESIAN_POINT ( 'NONE',  ( 20.00000000000004974, -2.506448799221099482E-14, 2.999999999999995559 ) ) ;
#1749=ADVANCED_FACE ( 'NONE', ( #4646 ), #4530, .F. ) ;
#1754=AXIS2_PLACEMENT_3D ( 'NONE', #3712, #21577, #721 ) ;
#1759=AXIS2_PLACEMENT_3D ( 'NONE', #7535, #9704, #14727 ) ;
#1760=ORIENTED_EDGE ( 'NONE', *, *, #4883, .T. ) ;
#1762=ORIENTED_EDGE ( 'NONE', *, *, #19139, .T. ) ;
#1764=ADVANCED_FACE ( 'NONE', ( #11512 ), #16551, .T. ) ;
#1766=EDGE_CURVE ( 'NONE', #1817, #14184, #21715, .T. ) ;
#1769=CARTESIAN_POINT ( 'NONE',  ( 2.220446049250313081E-13, -2.498001805406602216E-13, -6.859353255829918616 ) ) ;
#1779=DIRECTION ( 'NONE',  ( 1.000000000000000000, 1.208970125616053321E-17, 0.000000000000000000 ) ) ;
#1783=EDGE_CURVE ( 'NONE', #10281, #4282, #12160, .T. ) ;
#1784=DIRECTION ( 'NONE',  ( -1.000000000000000000, -5.354846555474805578E-15, 0.000000000000000000 ) ) ;
#1789=FACE_OUTER_BOUND ( 'NONE', #2176, .T. ) ;
#1793=AXIS2_PLACEMENT_3D ( 'NONE', #5535, #12510, #17457 ) ;
#1795=VERTEX_POINT ( 'NONE', #4419 ) ;
#1798=DIRECTION ( 'NONE',  ( 6.505213034913038160E-19, 3.903127820947822896E-18, 1.000000000000000000 ) ) ;
#1800=DIRECTION ( 'NONE',  ( -1.000000000000000000, -1.208970125616046080E-17, 6.505213034913038160E-19 ) ) ;
#1805=ORIENTED_EDGE ( 'NONE', *, *, #12333, .F. ) ;
#1809=CARTESIAN_POINT ( 'NONE',  ( 27.01645732367857633, 17.86915608785674792, 3.000000000000023537 ) ) ;
#1812=DIRECTION ( 'NONE',  ( 1.000000000000000000, 0.000000000000000000, 0.000000000000000000 ) ) ;
#1817=VERTEX_POINT ( 'NONE', #12074 ) ;
#1819=CIRCLE ( 'NONE', #19020, 19.11328065563150957 ) ;
#1822=CARTESIAN_POINT ( 'NONE',  ( 2.775557561562891351E-14, -2.775557561562891351E-14, 2.999999999999995559 ) ) ;
#1823=VERTEX_POINT ( 'NONE', #15269 ) ;
#1826=CARTESIAN_POINT ( 'NONE',  ( 28.45046755804883531, -15.62726112422599378, -2.999999999999971578 ) ) ;
#1827=DIRECTION ( 'NONE',  ( 6.505213034913038160E-19, 3.903127820947822896E-18, 1.000000000000000000 ) ) ;
#1829=CYLINDRICAL_SURFACE ( 'NONE', #7148, 0.9999999999999974465 ) ;
#1830=CIRCLE ( 'NONE', #4408, 19.11328065563152379 ) ;
#1832=DIRECTION ( 'NONE',  ( -1.000000000000000000, -1.208970125616044077E-17, 0.000000000000000000 ) ) ;
#1835=CARTESIAN_POINT ( 'NONE',  ( 34.88850421923977763, -1.128083539116253586, 3.000000000000023537 ) ) ;
#1837=CARTESIAN_POINT ( 'NONE',  ( 36.54278193890314697, 4.025500340002402311, -2.800654218530457484 ) ) ;
#1841=ADVANCED_FACE ( 'NONE', ( #10229 ), #21011, .T. ) ;
#1842=VERTEX_POINT ( 'NONE', #17221 ) ;
#1846=CARTESIAN_POINT ( 'NONE',  ( 2.775557561562891351E-14, 2.775557561562891351E-14, 5.750000000000001776 ) ) ;
#1854=FACE_OUTER_BOUND ( 'NONE', #17768, .T. ) ;
#1857=ORIENTED_EDGE ( 'NONE', *, *, #4842, .T. ) ;
#1863=ADVANCED_FACE ( 'NONE', ( #6926 ), #16193, .T. ) ;
#1866=EDGE_CURVE ( 'NONE', #18033, #8806, #17562, .T. ) ;
#1871=CARTESIAN_POINT ( 'NONE',  ( -8.646032897229122938, 31.21605069118058040, -6.999999999999950262 ) ) ;
#1875=VERTEX_POINT ( 'NONE', #3145 ) ;
#1878=ORIENTED_EDGE ( 'NONE', *, *, #9036, .T. ) ;
#1880=CIRCLE ( 'NONE', #5533, 1.000000000000001776 ) ;
#1883=ADVANCED_FACE ( 'NONE', ( #3605 ), #9242, .T. ) ;
#1885=ORIENTED_EDGE ( 'NONE', *, *, #3594, .F. ) ;
#1886=CARTESIAN_POINT ( 'NONE',  ( 35.43002037646326841, -7.196011215416819873, -2.933296326616337435 ) ) ;
#1900=CARTESIAN_POINT ( 'NONE',  ( -31.67162468655987340, -14.67611967928944594, -2.999999999999971578 ) ) ;
#1905=EDGE_CURVE ( 'NONE', #3795, #8449, #2994, .T. ) ;
#1907=DIRECTION ( 'NONE',  ( 1.000000000000000000, 1.208970125616067650E-17, 0.000000000000000000 ) ) ;
#1908=DIRECTION ( 'NONE',  ( -1.000000000000000000, -1.208970125616060717E-17, 0.000000000000000000 ) ) ;
#1912=AXIS2_PLACEMENT_3D ( 'NONE', #1557, #15854, #22421 ) ;
#1914=DIRECTION ( 'NONE',  ( 1.000000000000000000, 0.000000000000000000, 0.000000000000000000 ) ) ;
#1915=CARTESIAN_POINT ( 'NONE',  ( -30.98879172160200213, 17.38064605515573291, 3.000000000000043077 ) ) ;
#1916=CARTESIAN_POINT ( 'NONE',  ( -24.10117729468380077, 26.10603996529630777, 3.000000000000042188 ) ) ;
#1917=EDGE_CURVE ( 'NONE', #4478, #16652, #11956, .T. ) ;
#1919=ORIENTED_EDGE ( 'NONE', *, *, #19990, .F. ) ;
#1923=AXIS2_PLACEMENT_3D ( 'NONE', #18496, #11280, #15037 ) ;
#1926=CARTESIAN_POINT ( 'NONE',  ( 28.07080038625117524, 14.29266125237876928, 2.999999999999995559 ) ) ;
#1931=VERTEX_POINT ( 'NONE', #22513 ) ;
#1938=LINE ( 'NONE', #13847, #10442 ) ;
#1942=EDGE_LOOP ( 'NONE', ( #18055, #2733, #2323, #16683 ) ) ;
#1944=ORIENTED_EDGE ( 'NONE', *, *, #1708, .F. ) ;
#1947=TOROIDAL_SURFACE ( 'NONE', #3788, 34.90673715956759082, 8.750000000000000000 ) ;
#1957=EDGE_CURVE ( 'NONE', #12666, #15098, #19511, .T. ) ;
#1958=CARTESIAN_POINT ( 'NONE',  ( 2.775557561562891351E-14, 2.775557561562891351E-14, 5.750000000000001776 ) ) ;
#1959=DIRECTION ( 'NONE',  ( 1.000000000000000000, 0.000000000000000000, 0.000000000000000000 ) ) ;
#1968=CARTESIAN_POINT ( 'NONE',  ( 3.330669073875469621E-13, -1.110223024625156540E-13, -2.999999999999971578 ) ) ;
#1971=AXIS2_PLACEMENT_3D ( 'NONE', #21641, #673, #21759 ) ;
#1972=AXIS2_PLACEMENT_3D ( 'NONE', #8588, #18795, #6882 ) ;
#1974=EDGE_LOOP ( 'NONE', ( #17985, #19237, #10620, #7582 ) ) ;
#1976=SHAPE_REPRESENTATION_RELATIONSHIP ( 'NONE' , 'NONE' ,  #18960, #19467 ) ;
#1978=FACE_OUTER_BOUND ( 'NONE', #2696, .T. ) ;
#1983=DIRECTION ( 'NONE',  ( -6.505213034913038160E-19, -3.903127820947822896E-18, -1.000000000000000000 ) ) ;
#1993=ORIENTED_EDGE ( 'NONE', *, *, #14587, .T. ) ;
#1997=CIRCLE ( 'NONE', #4923, 3.000000000000002665 ) ;
#1999=CARTESIAN_POINT ( 'NONE',  ( -11.98978967046166666, -34.10919265018085866, 2.932969818539081786 ) ) ;
#2003=EDGE_LOOP ( 'NONE', ( #10767, #8699, #15633, #17642 ) ) ;
#2005=EDGE_CURVE ( 'NONE', #4617, #5340, #5421, .T. ) ;
#2007=EDGE_LOOP ( 'NONE', ( #10156, #21285, #13146, #10033 ) ) ;
#2009=CARTESIAN_POINT ( 'NONE',  ( -24.10368028608786162, 26.10969099697611995, -3.000000000000011546 ) ) ;
#2013=CIRCLE ( 'NONE', #5327, 19.11328065563151668 ) ;
#2014=EDGE_CURVE ( 'NONE', #15016, #3715, #20184, .T. ) ;
#2017=CYLINDRICAL_SURFACE ( 'NONE', #10457, 19.11328065563152379 ) ;
#2021=VECTOR ( 'NONE', #8797, 1000.000000000000000 ) ;
#2022=CARTESIAN_POINT ( 'NONE',  ( -23.65408649739100966, -22.22891329980539155, -2.999999999999995559 ) ) ;
#2023=DIRECTION ( 'NONE',  ( -1.000000000000000000, -1.208970125616063644E-17, 0.000000000000000000 ) ) ;
#2028=EDGE_CURVE ( 'NONE', #17302, #16867, #2252, .T. ) ;
#2031=VECTOR ( 'NONE', #22330, 1000.000000000000000 ) ;
#2032=FACE_OUTER_BOUND ( 'NONE', #17813, .T. ) ;
#2034=EDGE_CURVE ( 'NONE', #14303, #14783, #12839, .T. ) ;
#2038=CARTESIAN_POINT ( 'NONE',  ( -28.95348479018558407, 14.76298474240494940, 3.000000000000023537 ) ) ;
#2039=CARTESIAN_POINT ( 'NONE',  ( 3.330669073875469621E-13, -1.110223024625156540E-13, -2.999999999999971578 ) ) ;
#2043=AXIS2_PLACEMENT_3D ( 'NONE', #16183, #14231, #1784 ) ;
#2046=DIRECTION ( 'NONE',  ( 6.505213034913038160E-19, 3.903127820947822896E-18, 1.000000000000000000 ) ) ;
#2051=ORIENTED_EDGE ( 'NONE', *, *, #6256, .T. ) ;
#2052=LINE ( 'NONE', #19474, #7529 ) ;
#2054=TOROIDAL_SURFACE ( 'NONE', #5721, 34.90673715956759082, 8.750000000000000000 ) ;
#2055=VECTOR ( 'NONE', #12216, 1000.000000000000000 ) ;
#2059=ORIENTED_EDGE ( 'NONE', *, *, #6843, .T. ) ;
#2063=B_SPLINE_CURVE_WITH_KNOTS ( 'NONE', 3,
 ( #16023, #3899, #12464, #2173 ),
 .UNSPECIFIED., .F., .F.,
 ( 4, 4 ),
 ( 9.715086407478086874E-07, 0.001929643240672472169 ),
 .UNSPECIFIED. ) ;
#2065=ORIENTED_EDGE ( 'NONE', *, *, #19552, .T. ) ;
#2068=ORIENTED_EDGE ( 'NONE', *, *, #6955, .T. ) ;
#2075=CARTESIAN_POINT ( 'NONE',  ( 30.07487443287998374, -12.31876324338282380, -7.000000000000006217 ) ) ;
#2078=AXIS2_PLACEMENT_3D ( 'NONE', #2075, #9069, #5619 ) ;
#2079=VERTEX_POINT ( 'NONE', #21454 ) ;
#2082=DIRECTION ( 'NONE',  ( -1.000000000000000000, 9.802091999852181989E-15, 0.000000000000000000 ) ) ;
#2083=LINE ( 'NONE', #2429, #18051 ) ;
#2086=ORIENTED_EDGE ( 'NONE', *, *, #4485, .F. ) ;
#2087=CIRCLE ( 'NONE', #17827, 31.50000000000000711 ) ;
#2088=ORIENTED_EDGE ( 'NONE', *, *, #16733, .T. ) ;
#2089=AXIS2_PLACEMENT_3D ( 'NONE', #13590, #15322, #16836 ) ;
#2092=ADVANCED_FACE ( 'NONE', ( #1978 ), #8960, .F. ) ;
#2093=CARTESIAN_POINT ( 'NONE',  ( -29.33203831401591444, -20.06142356895425038, 3.000000000000049738 ) ) ;
#2096=DIRECTION ( 'NONE',  ( -6.505213034913038160E-19, -3.903127820947822896E-18, -1.000000000000000000 ) ) ;
#2099=CARTESIAN_POINT ( 'NONE',  ( -29.33526866242094755, 22.15900668633769044, -2.800654218530477912 ) ) ;
#2101=CARTESIAN_POINT ( 'NONE',  ( 31.11359284679418735, 4.918774254215718678, -6.999999999999999112 ) ) ;
#2104=ORIENTED_EDGE ( 'NONE', *, *, #1673, .F. ) ;
#2109=DIRECTION ( 'NONE',  ( 6.505213034913038160E-19, 3.903127820947822896E-18, 1.000000000000000000 ) ) ;
#2110=ORIENTED_EDGE ( 'NONE', *, *, #14828, .F. ) ;
#2111=DIRECTION ( 'NONE',  ( 1.000000000000000000, 0.000000000000000000, 0.000000000000000000 ) ) ;
#2127=DIRECTION ( 'NONE',  ( 1.000000000000000000, 0.000000000000000000, 0.000000000000000000 ) ) ;
#2133=DIRECTION ( 'NONE',  ( 1.000000000000000000, 0.000000000000000000, 0.000000000000000000 ) ) ;
#2136=CARTESIAN_POINT ( 'NONE',  ( 19.05255888325771352, 10.99999999999989875, 2.999999999999995559 ) ) ;
#2140=EDGE_CURVE ( 'NONE', #19773, #877, #2555, .T. ) ;
#2143=CIRCLE ( 'NONE', #12004, 31.50000000000000711 ) ;
#2145=CARTESIAN_POINT ( 'NONE',  ( 14.93538271375446946, 34.13396246814556889, 3.000000000000023537 ) ) ;
#2146=B_SPLINE_CURVE_WITH_KNOTS ( 'NONE', 3,
 ( #945, #20198, #18703, #14900 ),
 .UNSPECIFIED., .F., .F.,
 ( 4, 4 ),
 ( 0.001893031756885906478, 0.003808480026564050377 ),
 .UNSPECIFIED. ) ;
#2154=CYLINDRICAL_SURFACE ( 'NONE', #13661, 31.50000000000000711 ) ;
#2155=AXIS2_PLACEMENT_3D ( 'NONE', #4219, #14847, #12678 ) ;
#2162=CARTESIAN_POINT ( 'NONE',  ( 5.551115123125782702E-14, -1.387778780781445676E-13, -5.749999999999949374 ) ) ;
#2163=EDGE_CURVE ( 'NONE', #17952, #22537, #11802, .T. ) ;
#2164=ORIENTED_EDGE ( 'NONE', *, *, #16598, .T. ) ;
#2166=DIRECTION ( 'NONE',  ( 6.505213034913038160E-19, 3.903127820947822896E-18, 1.000000000000000000 ) ) ;
#2168=VERTEX_POINT ( 'NONE', #13514 ) ;
#2170=DIRECTION ( 'NONE',  ( 6.505213034913038160E-19, 3.903127820947822896E-18, 1.000000000000000000 ) ) ;
#2173=CARTESIAN_POINT ( 'NONE',  ( -19.59430950039299546, 28.88846368933323205, 2.999999999999995559 ) ) ;
#2175=ADVANCED_FACE ( 'NONE', ( #8716 ), #1271, .F. ) ;
#2176=EDGE_LOOP ( 'NONE', ( #8644, #3320, #15371, #20064, #8776, #7471 ) ) ;
#2177=CARTESIAN_POINT ( 'NONE',  ( -4.153516728483839238, 35.28654656445758064, 3.000000000000046629 ) ) ;
#2181=ORIENTED_EDGE ( 'NONE', *, *, #8709, .T. ) ;
#2182=FACE_OUTER_BOUND ( 'NONE', #17675, .T. ) ;
#2185=CARTESIAN_POINT ( 'NONE',  ( 29.33526866242106124, -22.15900668633785742, 2.800654218530492123 ) ) ;
#2187=DIRECTION ( 'NONE',  ( -1.000000000000000000, -9.076011110974242363E-16, 0.000000000000000000 ) ) ;
#2188=LINE ( 'NONE', #12713, #13951 ) ;
#2190=VERTEX_POINT ( 'NONE', #16963 ) ;
#2192=FACE_OUTER_BOUND ( 'NONE', #12078, .T. ) ;
#2194=ORIENTED_EDGE ( 'NONE', *, *, #14920, .F. ) ;
#2200=EDGE_CURVE ( 'NONE', #20280, #8421, #7747, .T. ) ;
#2202=VERTEX_POINT ( 'NONE', #1614 ) ;
#2207=CYLINDRICAL_SURFACE ( 'NONE', #18576, 1.000000000000000888 ) ;
#2213=DIRECTION ( 'NONE',  ( -6.505213034913038160E-19, -3.903127820947822896E-18, -1.000000000000000000 ) ) ;
#2215=ORIENTED_EDGE ( 'NONE', *, *, #3324, .T. ) ;
#2221=VERTEX_POINT ( 'NONE', #3002 ) ;
#2222=CARTESIAN_POINT ( 'NONE',  ( -4.171001175319544174, -35.79662727779886211, -2.999999999999995559 ) ) ;
#2226=CARTESIAN_POINT ( 'NONE',  ( -11.85401191286875111, -32.83234229683740324, 3.000000000000023537 ) ) ;
#2228=CARTESIAN_POINT ( 'NONE',  ( 26.10969099697632956, 24.10368028608786517, -3.000000000000007105 ) ) ;
#2239=EDGE_CURVE ( 'NONE', #5417, #22152, #1154, .T. ) ;
#2241=CARTESIAN_POINT ( 'NONE',  ( -13.83143812983110621, 29.36548507648009831, -2.999999999999995559 ) ) ;
#2244=CARTESIAN_POINT ( 'NONE',  ( -28.96193690644918561, -14.74639653023249153, -2.999999999999988898 ) ) ;
#2246=CARTESIAN_POINT ( 'NONE',  ( 28.45046755804905914, -15.62726112422602220, -7.000000000000006217 ) ) ;
#2252=CIRCLE ( 'NONE', #19087, 28.00000000000001066 ) ;
#2253=AXIS2_PLACEMENT_3D ( 'NONE', #8380, #11803, #11922 ) ;
#2254=CARTESIAN_POINT ( 'NONE',  ( -18.83615802559791774, 32.14641817400182333, 2.999999999999995559 ) ) ;
#2256=ORIENTED_EDGE ( 'NONE', *, *, #13298, .F. ) ;
#2263=DIRECTION ( 'NONE',  ( 1.000000000000000000, 1.208970125616053321E-17, 0.000000000000000000 ) ) ;
#2266=EDGE_CURVE ( 'NONE', #8449, #4746, #10218, .T. ) ;
#2270=CARTESIAN_POINT ( 'NONE',  ( 1.110223024625156540E-13, -5.551115123125782702E-14, -6.999999999999950262 ) ) ;
#2273=LINE ( 'NONE', #16242, #18852 ) ;
#2275=ORIENTED_EDGE ( 'NONE', *, *, #13053, .T. ) ;
#2276=CARTESIAN_POINT ( 'NONE',  ( -19.99999999999979394, -2.775557561562891351E-14, -2.999999999999971578 ) ) ;
#2277=VERTEX_POINT ( 'NONE', #11920 ) ;
#2278=DIRECTION ( 'NONE',  ( 6.505213034913038160E-19, 3.903127820947822896E-18, 1.000000000000000000 ) ) ;
#2282=ORIENTED_EDGE ( 'NONE', *, *, #17720, .F. ) ;
#2283=CARTESIAN_POINT ( 'NONE',  ( -30.13956425491233659, -21.05198877411806890, -2.000000000000001776 ) ) ;
#2286=CARTESIAN_POINT ( 'NONE',  ( -4.025500340002485800, 36.54278193890309012, 2.800654218530485018 ) ) ;
#2288=CYLINDRICAL_SURFACE ( 'NONE', #7270, 0.9999999999999974465 ) ;
#2289=ORIENTED_EDGE ( 'NONE', *, *, #14020, .T. ) ;
#2291=CARTESIAN_POINT ( 'NONE',  ( -27.19760187735847978, -24.73600648735121865, -1.999999999999977573 ) ) ;
#2292=VERTEX_POINT ( 'NONE', #15574 ) ;
#2293=CARTESIAN_POINT ( 'NONE',  ( -17.99999999999980460, -8.348434146949763185E-14, 4.999999999999993783 ) ) ;
#2294=EDGE_CURVE ( 'NONE', #2966, #18701, #22597, .T. ) ;
#2298=CARTESIAN_POINT ( 'NONE',  ( 35.99819890246955367, -7.463862311151231665, -2.000000000000001776 ) ) ;
#2300=LINE ( 'NONE', #12827, #21107 ) ;
#2308=VERTEX_POINT ( 'NONE', #5284 ) ;
#2315=ORIENTED_EDGE ( 'NONE', *, *, #18484, .T. ) ;
#2318=DIRECTION ( 'NONE',  ( -6.505213034913038160E-19, -3.903127820947822896E-18, -1.000000000000000000 ) ) ;
#2321=CARTESIAN_POINT ( 'NONE',  ( -18.83615802559775076, 32.14641817400176649, -2.999999999999971578 ) ) ;
#2322=CARTESIAN_POINT ( 'NONE',  ( -30.48934413892756368, 16.99647590252650886, -2.999999999999995559 ) ) ;
#2323=ORIENTED_EDGE ( 'NONE', *, *, #21288, .T. ) ;
#2326=DIRECTION ( 'NONE',  ( -1.000000000000000000, -1.208970125616077665E-17, 0.000000000000000000 ) ) ;
#2327=CARTESIAN_POINT ( 'NONE',  ( -33.51030287062352642, -15.12081897056683033, 2.800654218530502337 ) ) ;
#2328=CARTESIAN_POINT ( 'NONE',  ( -21.65063509461097269, 12.49999999999990052, -5.000000000000004441 ) ) ;
#2329=ORIENTED_EDGE ( 'NONE', *, *, #1957, .T. ) ;
#2330=CIRCLE ( 'NONE', #15851, 19.11328065563152023 ) ;
#2335=EDGE_CURVE ( 'NONE', #1842, #1434, #12463, .T. ) ;
#2342=DIRECTION ( 'NONE',  ( 1.000000000000000000, 0.000000000000000000, 0.000000000000000000 ) ) ;
#2343=VECTOR ( 'NONE', #13022, 1000.000000000000000 ) ;
#2344=VECTOR ( 'NONE', #3447, 1000.000000000000000 ) ;
#2345=DIRECTION ( 'NONE',  ( -6.505213034913038160E-19, -3.903127820947822896E-18, -1.000000000000000000 ) ) ;
#2349=ORIENTED_EDGE ( 'NONE', *, *, #14496, .T. ) ;
#2350=VERTEX_POINT ( 'NONE', #7215 ) ;
#2354=DIRECTION ( 'NONE',  ( -6.505213034913038160E-19, -3.903127820947822896E-18, -1.000000000000000000 ) ) ;
#2356=DIRECTION ( 'NONE',  ( 6.505213034913038160E-19, 3.903127820947822896E-18, 1.000000000000000000 ) ) ;
#2358=AXIS2_PLACEMENT_3D ( 'NONE', #94, #10399, #19249 ) ;
#2359=B_SPLINE_CURVE_WITH_KNOTS ( 'NONE', 3,
 ( #20809, #5120, #6828, #13792 ),
 .UNSPECIFIED., .F., .F.,
 ( 4, 4 ),
 ( 9.715086431275246711E-07, 0.001929643240674561860 ),
 .UNSPECIFIED. ) ;
#2370=DIRECTION ( 'NONE',  ( 1.000000000000000000, 1.208970125616062874E-17, 0.000000000000000000 ) ) ;
#2373=ORIENTED_EDGE ( 'NONE', *, *, #16600, .T. ) ;
#2387=DIRECTION ( 'NONE',  ( 6.505213034913038160E-19, 3.903127820947822896E-18, 1.000000000000000000 ) ) ;
#2388=VERTEX_POINT ( 'NONE', #10481 ) ;
#2389=CARTESIAN_POINT ( 'NONE',  ( 37.07861450834834471, -3.656418565264496490, -2.999999999999971578 ) ) ;
#2394=ORIENTED_EDGE ( 'NONE', *, *, #1237, .T. ) ;
#2395=DIRECTION ( 'NONE',  ( -6.505213034913038160E-19, -3.903127820947822896E-18, -1.000000000000000000 ) ) ;
#2401=ORIENTED_EDGE ( 'NONE', *, *, #2034, .T. ) ;
#2407=VERTEX_POINT ( 'NONE', #12428 ) ;
#2416=AXIS2_PLACEMENT_3D ( 'NONE', #1603, #15788, #10406 ) ;
#2420=CARTESIAN_POINT ( 'NONE',  ( 3.608224830031758756E-13, -2.775557561562891351E-14, -4.999999999999997335 ) ) ;
#2429=CARTESIAN_POINT ( 'NONE',  ( -9.999999999999758415, -3.000000000000169198, -4.999999999999984013 ) ) ;
#2430=CIRCLE ( 'NONE', #4262, 1.000000000000000888 ) ;
#2432=AXIS2_PLACEMENT_3D ( 'NONE', #10888, #7346, #15812 ) ;
#2434=EDGE_LOOP ( 'NONE', ( #8528, #1302, #8110, #3876 ) ) ;
#2435=AXIS2_PLACEMENT_3D ( 'NONE', #3194, #11770, #3075 ) ;
#2440=DIRECTION ( 'NONE',  ( 6.505213034913038160E-19, 3.903127820947822896E-18, 1.000000000000000000 ) ) ;
#2441=DIRECTION ( 'NONE',  ( 1.000000000000000000, 0.000000000000000000, 0.000000000000000000 ) ) ;
#2443=FACE_OUTER_BOUND ( 'NONE', #20008, .T. ) ;
#2446=ORIENTED_EDGE ( 'NONE', *, *, #3743, .F. ) ;
#2447=LINE ( 'NONE', #19860, #304 ) ;
#2448=CARTESIAN_POINT ( 'NONE',  ( 28.95348479018572263, -14.76298474240511638, -6.999999999999999112 ) ) ;
#2450=CARTESIAN_POINT ( 'NONE',  ( 21.05198877411804048, -30.13956425491232238, 2.800654218530485018 ) ) ;
#2451=CARTESIAN_POINT ( 'NONE',  ( 1.110223024625156540E-13, -5.551115123125782702E-14, -6.999999999999950262 ) ) ;
#2452=DIRECTION ( 'NONE',  ( -6.505213034913038160E-19, -3.903127820947822896E-18, -1.000000000000000000 ) ) ;
#2453=EDGE_LOOP ( 'NONE', ( #11507, #15045, #19659, #10420 ) ) ;
#2454=LINE ( 'NONE', #11259, #17473 ) ;
#2459=CARTESIAN_POINT ( 'NONE',  ( -17.09029715894932977, 27.64365646977273627, -6.999999999999999112 ) ) ;
#2463=CARTESIAN_POINT ( 'NONE',  ( 18.22261011550299514, 31.92986134326217140, -2.800654218530460593 ) ) ;
#2467=EDGE_CURVE ( 'NONE', #2631, #2388, #19331, .T. ) ;
#2489=AXIS2_PLACEMENT_3D ( 'NONE', #175, #18139, #1908 ) ;
#2492=VECTOR ( 'NONE', #4133, 1000.000000000000000 ) ;
#2494=AXIS2_PLACEMENT_3D ( 'NONE', #6744, #17162, #8461 ) ;
#2498=EDGE_CURVE ( 'NONE', #312, #5560, #12650, .T. ) ;
#2499=CYLINDRICAL_SURFACE ( 'NONE', #3959, 31.50000000000001421 ) ;
#2500=AXIS2_PLACEMENT_3D ( 'NONE', #5716, #14639, #10983 ) ;
#2501=EDGE_CURVE ( 'NONE', #15970, #12342, #4312, .T. ) ;
#2509=CIRCLE ( 'NONE', #8007, 31.50000000000000711 ) ;
#2510=ORIENTED_EDGE ( 'NONE', *, *, #3448, .F. ) ;
#2515=DIRECTION ( 'NONE',  ( 1.000000000000000000, 0.000000000000000000, 0.000000000000000000 ) ) ;
#2517=VERTEX_POINT ( 'NONE', #21610 ) ;
#2518=CARTESIAN_POINT ( 'NONE',  ( 4.025500340002624355, -36.54278193890314697, 2.800654218530485018 ) ) ;
#2519=CARTESIAN_POINT ( 'NONE',  ( -17.66631876130915657, 31.41173278719225337, -6.999999999999950262 ) ) ;
#2521=AXIS2_PLACEMENT_3D ( 'NONE', #13809, #20827, #22206 ) ;
#2522=VECTOR ( 'NONE', #1394, 1000.000000000000000 ) ;
#2526=TOROIDAL_SURFACE ( 'NONE', #309, 34.90673715956759082, 8.750000000000000000 ) ;
#2531=CARTESIAN_POINT ( 'NONE',  ( 2.220446049250313081E-13, 2.775557561562891351E-14, -2.800654218530485018 ) ) ;
#2534=DIRECTION ( 'NONE',  ( -1.000000000000000000, -1.208970125616077665E-17, 0.000000000000000000 ) ) ;
#2535=CYLINDRICAL_SURFACE ( 'NONE', #2656, 36.76383501243555685 ) ;
#2536=AXIS2_PLACEMENT_3D ( 'NONE', #10267, #6850, #10490 ) ;
#2540=AXIS2_PLACEMENT_3D ( 'NONE', #3716, #1983, #258 ) ;
#2542=ADVANCED_FACE ( 'NONE', ( #14365 ), #14252, .F. ) ;
#2543=ORIENTED_EDGE ( 'NONE', *, *, #8775, .F. ) ;
#2547=ADVANCED_FACE ( 'NONE', ( #8998 ), #10944, .T. ) ;
#2551=VECTOR ( 'NONE', #2850, 1000.000000000000000 ) ;
#2554=ORIENTED_EDGE ( 'NONE', *, *, #9741, .F. ) ;
#2555=LINE ( 'NONE', #820, #5193 ) ;
#2558=CARTESIAN_POINT ( 'NONE',  ( 24.79619811426236708, -21.00948735876897899, 3.000000000000016431 ) ) ;
#2559=DIRECTION ( 'NONE',  ( -1.000000000000000000, 0.000000000000000000, 0.000000000000000000 ) ) ;
#2560=VERTEX_POINT ( 'NONE', #5909 ) ;
#2563=VERTEX_POINT ( 'NONE', #2241 ) ;
#2568=LINE ( 'NONE', #18257, #2055 ) ;
#2569=CARTESIAN_POINT ( 'NONE',  ( 22.15900668633785742, 29.33526866242092268, -1.999999999999991340 ) ) ;
#2570=VERTEX_POINT ( 'NONE', #21719 ) ;
#2571=ADVANCED_FACE ( 'NONE', ( #12989 ), #9225, .T. ) ;
#2574=ORIENTED_EDGE ( 'NONE', *, *, #9619, .T. ) ;
#2576=CARTESIAN_POINT ( 'NONE',  ( 21.69710536060296135, 28.14364593009908688, 3.000000000000044853 ) ) ;
#2580=VERTEX_POINT ( 'NONE', #9347 ) ;
#2581=AXIS2_PLACEMENT_3D ( 'NONE', #3232, #5500, #15908 ) ;
#2583=ORIENTED_EDGE ( 'NONE', *, *, #2335, .F. ) ;
#2584=ORIENTED_EDGE ( 'NONE', *, *, #9100, .F. ) ;
#2589=ORIENTED_EDGE ( 'NONE', *, *, #4315, .F. ) ;
#2593=VERTEX_POINT ( 'NONE', #19782 ) ;
#2598=ADVANCED_FACE ( 'NONE', ( #16330 ), #20004, .F. ) ;
#2600=AXIS2_PLACEMENT_3D ( 'NONE', #4769, #11738, #9684 ) ;
#2601=CARTESIAN_POINT ( 'NONE',  ( -8.999999999999841904, -5.551115123125782702E-14, 5.000000000000022204 ) ) ;
#2602=LINE ( 'NONE', #870, #15961 ) ;
#2605=ORIENTED_EDGE ( 'NONE', *, *, #14981, .F. ) ;
#2606=B_SPLINE_CURVE_WITH_KNOTS ( 'NONE', 3,
 ( #12871, #19880, #5454, #8994 ),
 .UNSPECIFIED., .F., .F.,
 ( 4, 4 ),
 ( 9.545285769294494988E-07, 0.001900595205834635293 ),
 .UNSPECIFIED. ) ;
#2608=ORIENTED_EDGE ( 'NONE', *, *, #10655, .F. ) ;
#2611=VECTOR ( 'NONE', #4531, 1000.000000000000000 ) ;
#2612=EDGE_CURVE ( 'NONE', #10824, #5940, #858, .T. ) ;
#2613=B_SPLINE_CURVE_WITH_KNOTS ( 'NONE', 3,
 ( #12709, #19730, #11001, #9286 ),
 .UNSPECIFIED., .F., .F.,
 ( 4, 4 ),
 ( 9.715086411615364248E-07, 0.001929643240672571482 ),
 .UNSPECIFIED. ) ;
#2614=CARTESIAN_POINT ( 'NONE',  ( 17.09029715894957846, -27.64365646977279312, -2.999999999999992450 ) ) ;
#2615=CARTESIAN_POINT ( 'NONE',  ( -8.646032897229122938, 31.21605069118058040, -2.999999999999957367 ) ) ;
#2616=B_SPLINE_CURVE_WITH_KNOTS ( 'NONE', 3,
 ( #15225, #20300, #7800, #16510 ),
 .UNSPECIFIED., .F., .F.,
 ( 4, 4 ),
 ( 9.715086408138421055E-07, 0.001929643240672349221 ),
 .UNSPECIFIED. ) ;
#2621=EDGE_CURVE ( 'NONE', #11042, #7992, #9766, .T. ) ;
#2622=DIRECTION ( 'NONE',  ( -6.505213034913038160E-19, -3.903127820947822896E-18, -1.000000000000000000 ) ) ;
#2627=DIRECTION ( 'NONE',  ( 6.505213034913038160E-19, 3.903127820947822896E-18, 1.000000000000000000 ) ) ;
#2628=LINE ( 'NONE', #7428, #17740 ) ;
#2631=VERTEX_POINT ( 'NONE', #6136 ) ;
#2632=FACE_BOUND ( 'NONE', #15399, .T. ) ;
#2634=DIRECTION ( 'NONE',  ( -1.000000000000000000, 1.070969311094961116E-14, 0.000000000000000000 ) ) ;
#2639=DIRECTION ( 'NONE',  ( 1.000000000000000000, 0.000000000000000000, 0.000000000000000000 ) ) ;
#2641=ORIENTED_EDGE ( 'NONE', *, *, #12470, .F. ) ;
#2644=CARTESIAN_POINT ( 'NONE',  ( -9.708269511265104512, 33.52953626616034200, -2.999999999999978240 ) ) ;
#2645=DIRECTION ( 'NONE',  ( -1.000000000000000000, 0.000000000000000000, 0.000000000000000000 ) ) ;
#2647=DIRECTION ( 'NONE',  ( -6.505213034913038160E-19, -3.903127820947822896E-18, -1.000000000000000000 ) ) ;
#2650=CARTESIAN_POINT ( 'NONE',  ( 6.742883674876798850, 34.24928931925757780, -2.999999999999971578 ) ) ;
#2656=AXIS2_PLACEMENT_3D ( 'NONE', #13260, #18445, #2759 ) ;
#2663=ADVANCED_FACE ( 'NONE', ( #20119 ), #6588, .F. ) ;
#2664=ORIENTED_EDGE ( 'NONE', *, *, #14038, .T. ) ;
#2666=DIRECTION ( 'NONE',  ( 6.505213034913038160E-19, 3.903127820947822896E-18, 1.000000000000000000 ) ) ;
#2669=DIRECTION ( 'NONE',  ( 4.718764931986839378E-35, -3.903127820947822896E-18, -1.000000000000000000 ) ) ;
#2675=AXIS2_PLACEMENT_3D ( 'NONE', #5443, #19768, #19533 ) ;
#2677=ADVANCED_FACE ( 'NONE', ( #13104 ), #1194, .T. ) ;
#2687=CARTESIAN_POINT ( 'NONE',  ( 24.62019382530528233, -4.341204441673129466, 3.000000000000023537 ) ) ;
#2689=VECTOR ( 'NONE', #2724, 1000.000000000000000 ) ;
#2691=CIRCLE ( 'NONE', #502, 0.9999999999999974465 ) ;
#2692=VERTEX_POINT ( 'NONE', #15043 ) ;
#2694=VERTEX_POINT ( 'NONE', #13550 ) ;
#2695=ADVANCED_FACE ( 'NONE', ( #13208 ), #4422, .F. ) ;
#2696=EDGE_LOOP ( 'NONE', ( #10369, #9322, #10556, #3613 ) ) ;
#2697=CARTESIAN_POINT ( 'NONE',  ( 30.13956425491251423, 21.05198877411795877, -1.999999999999953149 ) ) ;
#2700=ORIENTED_EDGE ( 'NONE', *, *, #9245, .T. ) ;
#2701=CARTESIAN_POINT ( 'NONE',  ( -30.13956425491234725, -21.05198877411829272, -2.800654218530471251 ) ) ;
#2705=EDGE_CURVE ( 'NONE', #12156, #5124, #17853, .T. ) ;
#2707=ORIENTED_EDGE ( 'NONE', *, *, #21736, .F. ) ;
#2708=CARTESIAN_POINT ( 'NONE',  ( -13.74639653023205277, 28.96193690644924246, -7.000000000000006217 ) ) ;
#2714=AXIS2_PLACEMENT_3D ( 'NONE', #1442, #8428, #15056 ) ;
#2715=CARTESIAN_POINT ( 'NONE',  ( 14.30873905802343415, 28.06260833510304664, -6.999999999999950262 ) ) ;
#2716=EDGE_CURVE ( 'NONE', #20782, #12370, #2143, .T. ) ;
#2717=CARTESIAN_POINT ( 'NONE',  ( 3.330669073875469621E-13, -1.110223024625156540E-13, -2.999999999999971578 ) ) ;
#2718=VERTEX_POINT ( 'NONE', #16895 ) ;
#2719=EDGE_LOOP ( 'NONE', ( #4492, #6449, #8085, #81 ) ) ;
#2722=VERTEX_POINT ( 'NONE', #9569 ) ;
#2724=DIRECTION ( 'NONE',  ( -6.505213034913038160E-19, -3.903127820947822896E-18, -1.000000000000000000 ) ) ;
#2730=FACE_OUTER_BOUND ( 'NONE', #8226, .T. ) ;
#2733=ORIENTED_EDGE ( 'NONE', *, *, #21057, .T. ) ;
#2735=DIRECTION ( 'NONE',  ( 1.000000000000000000, 0.000000000000000000, 0.000000000000000000 ) ) ;
#2740=CARTESIAN_POINT ( 'NONE',  ( 34.65667543218833657, 4.170748987303380062, 2.999999999999999112 ) ) ;
#2741=EDGE_CURVE ( 'NONE', #10740, #2718, #7858, .T. ) ;
#2751=CARTESIAN_POINT ( 'NONE',  ( 27.84804035626045504, -24.75236754129161909, -7.000000000000006217 ) ) ;
#2752=EDGE_CURVE ( 'NONE', #9113, #8849, #1025, .T. ) ;
#2753=CARTESIAN_POINT ( 'NONE',  ( 2.775557561562891351E-14, 2.775557561562891351E-14, 5.750000000000001776 ) ) ;
#2755=CIRCLE ( 'NONE', #14437, 19.11328065563152379 ) ;
#2758=CIRCLE ( 'NONE', #14439, 36.76383501243555685 ) ;
#2759=DIRECTION ( 'NONE',  ( -1.000000000000000000, -1.208970125616044077E-17, 0.000000000000000000 ) ) ;
#2760=ORIENTED_EDGE ( 'NONE', *, *, #20514, .T. ) ;
#2761=CARTESIAN_POINT ( 'NONE',  ( -21.65063509461084834, 12.49999999999967848, -2.999999999999988898 ) ) ;
#2762=DIRECTION ( 'NONE',  ( 6.505213034913038160E-19, 3.903127820947822896E-18, 1.000000000000000000 ) ) ;
#2764=CARTESIAN_POINT ( 'NONE',  ( 3.608224830031758756E-13, -25.00000000000021672, -2.999999999999999112 ) ) ;
#2766=CIRCLE ( 'NONE', #21789, 19.11328065563152379 ) ;
#2769=CARTESIAN_POINT ( 'NONE',  ( -21.94460005644892675, -28.73837443790567647, -2.932164912090524655 ) ) ;
#2772=VERTEX_POINT ( 'NONE', #6931 ) ;
#2776=VECTOR ( 'NONE', #1461, 1000.000000000000000 ) ;
#2778=DIRECTION ( 'NONE',  ( -6.505213034913038160E-19, -3.903127820947822896E-18, -1.000000000000000000 ) ) ;
#2781=CARTESIAN_POINT ( 'NONE',  ( 2.775557561562891351E-14, 2.775557561562891351E-14, 5.750000000000001776 ) ) ;
#2784=CARTESIAN_POINT ( 'NONE',  ( 2.220446049250313081E-13, -2.498001805406602216E-13, -6.859353255829918616 ) ) ;
#2785=VERTEX_POINT ( 'NONE', #20907 ) ;
#2787=CARTESIAN_POINT ( 'NONE',  ( -32.89708536800386440, -15.00428685838208587, 2.932460736555834835 ) ) ;
#2791=DIRECTION ( 'NONE',  ( 6.505213034913038160E-19, 3.903127820947822896E-18, 1.000000000000000000 ) ) ;
#2793=ADVANCED_FACE ( 'NONE', ( #8416 ), #15289, .T. ) ;
#2799=ORIENTED_EDGE ( 'NONE', *, *, #14942, .F. ) ;
#2801=DIRECTION ( 'NONE',  ( -6.505213034913038160E-19, -3.903127820947822896E-18, -1.000000000000000000 ) ) ;
#2806=ORIENTED_EDGE ( 'NONE', *, *, #7077, .F. ) ;
#2809=AXIS2_PLACEMENT_3D ( 'NONE', #2915, #5082, #18823 ) ;
#2811=CARTESIAN_POINT ( 'NONE',  ( 24.41514043009218682, 26.50842683089740959, -6.999999999999999112 ) ) ;
#2813=CARTESIAN_POINT ( 'NONE',  ( -29.33526866242079478, 22.15900668633771886, 2.800654218530485018 ) ) ;
#2820=CARTESIAN_POINT ( 'NONE',  ( 2.775557561562891351E-14, -2.775557561562891351E-14, 2.999999999999999112 ) ) ;
#2823=CARTESIAN_POINT ( 'NONE',  ( -34.65667543218827262, -4.170748987303407596, -2.999999999999971578 ) ) ;
#2824=AXIS2_PLACEMENT_3D ( 'NONE', #2761, #6303, #9743 ) ;
#2834=B_SPLINE_CURVE_WITH_KNOTS ( 'NONE', 3,
 ( #909, #4362, #689, #7673 ),
 .UNSPECIFIED., .F., .F.,
 ( 4, 4 ),
 ( 9.545285769850769053E-07, 0.001900595205834759759 ),
 .UNSPECIFIED. ) ;
#2835=AXIS2_PLACEMENT_3D ( 'NONE', #12849, #13071, #3011 ) ;
#2838=DIRECTION ( 'NONE',  ( -6.505213034913038160E-19, -3.903127820947822896E-18, -1.000000000000000000 ) ) ;
#2841=DIRECTION ( 'NONE',  ( 6.505213034913038160E-19, 3.903127820947822896E-18, 1.000000000000000000 ) ) ;
#2843=CARTESIAN_POINT ( 'NONE',  ( -27.64365646977254443, -17.09029715894946833, 3.000000000000012879 ) ) ;
#2848=TOROIDAL_SURFACE ( 'NONE', #1754, 34.90673715956759082, 8.750000000000000000 ) ;
#2850=DIRECTION ( 'NONE',  ( 6.505213034913038160E-19, 3.903127820947822896E-18, 1.000000000000000000 ) ) ;
#2855=AXIS2_PLACEMENT_3D ( 'NONE', #4502, #20089, #13181 ) ;
#2856=CARTESIAN_POINT ( 'NONE',  ( 31.11077005834453502, -4.936596639065232495, 2.999999999999995559 ) ) ;
#2859=CARTESIAN_POINT ( 'NONE',  ( 27.56232195404084706, -21.41958700883264655, -2.999999999999954259 ) ) ;
#2861=EDGE_CURVE ( 'NONE', #14184, #1555, #463, .T. ) ;
#2865=ORIENTED_EDGE ( 'NONE', *, *, #3, .F. ) ;
#2877=CARTESIAN_POINT ( 'NONE',  ( 1.110223024625156540E-13, -5.551115123125782702E-14, -6.999999999999950262 ) ) ;
#2882=VERTEX_POINT ( 'NONE', #1656 ) ;
#2884=VECTOR ( 'NONE', #11383, 1000.000000000000000 ) ;
#2886=CARTESIAN_POINT ( 'NONE',  ( 34.65667543218853552, 4.170748987303296573, -2.999999999999975131 ) ) ;
#2889=EDGE_CURVE ( 'NONE', #5874, #11652, #16575, .T. ) ;
#2894=ORIENTED_EDGE ( 'NONE', *, *, #15318, .T. ) ;
#2897=PLANE ( 'NONE',  #16863 ) ;
#2912=CARTESIAN_POINT ( 'NONE',  ( -15.12081897056648216, 33.51030287062351221, -1.999999999999977573 ) ) ;
#2914=ORIENTED_EDGE ( 'NONE', *, *, #20129, .F. ) ;
#2915=CARTESIAN_POINT ( 'NONE',  ( -7.094908322883064500, 35.33352588067081967, 3.000000000000023537 ) ) ;
#2919=CARTESIAN_POINT ( 'NONE',  ( -4.171001175319322130, -35.79662727779903264, 3.000000000000023537 ) ) ;
#2920=CARTESIAN_POINT ( 'NONE',  ( 2.775557561562891351E-13, 3.000000000000002665, -5.000000000000004441 ) ) ;
#2925=ORIENTED_EDGE ( 'NONE', *, *, #20473, .F. ) ;
#2927=EDGE_CURVE ( 'NONE', #2593, #18617, #2447, .T. ) ;
#2928=ORIENTED_EDGE ( 'NONE', *, *, #5415, .T. ) ;
#2932=DIRECTION ( 'NONE',  ( 6.505213034913038160E-19, 3.903127820947822896E-18, 1.000000000000000000 ) ) ;
#2936=LINE ( 'NONE', #22150, #15177 ) ;
#2940=CARTESIAN_POINT ( 'NONE',  ( -34.88850421923980605, 1.128083539116031542, 2.999999999999995559 ) ) ;
#2942=EDGE_CURVE ( 'NONE', #11842, #14574, #9813, .T. ) ;
#2943=AXIS2_PLACEMENT_3D ( 'NONE', #8132, #16377, #4128 ) ;
#2944=CARTESIAN_POINT ( 'NONE',  ( 2.775557561562891351E-14, 2.775557561562891351E-14, 5.750000000000001776 ) ) ;
#2948=EDGE_CURVE ( 'NONE', #4189, #2718, #12723, .T. ) ;
#2949=VERTEX_POINT ( 'NONE', #18132 ) ;
#2951=DIRECTION ( 'NONE',  ( 1.000000000000000000, 1.208970125616067650E-17, 0.000000000000000000 ) ) ;
#2954=EDGE_CURVE ( 'NONE', #17558, #7013, #4701, .T. ) ;
#2955=AXIS2_PLACEMENT_3D ( 'NONE', #8908, #19572, #19462 ) ;
#2960=CARTESIAN_POINT ( 'NONE',  ( 36.54278193890331039, 4.025500340002458266, 2.800654218530485018 ) ) ;
#2962=EDGE_CURVE ( 'NONE', #7988, #14674, #7621, .T. ) ;
#2963=ORIENTED_EDGE ( 'NONE', *, *, #3662, .T. ) ;
#2964=CARTESIAN_POINT ( 'NONE',  ( 28.07080038625092655, 14.29266125237893448, -2.999999999999999112 ) ) ;
#2966=VERTEX_POINT ( 'NONE', #483 ) ;
#2968=CARTESIAN_POINT ( 'NONE',  ( -34.65667543218827262, -4.170748987303407596, -2.999999999999971578 ) ) ;
#2971=CIRCLE ( 'NONE', #15753, 36.76383501243555685 ) ;
#2973=CIRCLE ( 'NONE', #7343, 1.000000000000000888 ) ;
#2986=ORIENTED_EDGE ( 'NONE', *, *, #20605, .F. ) ;
#2988=DIRECTION ( 'NONE',  ( -1.000000000000000000, -1.208970125616014957E-17, 0.000000000000000000 ) ) ;
#2992=CARTESIAN_POINT ( 'NONE',  ( -28.96193690644939522, -14.74639653023249153, 2.999999999999995559 ) ) ;
#2993=CARTESIAN_POINT ( 'NONE',  ( -22.15900668633755188, -29.33526866242114295, -2.800654218530433059 ) ) ;
#2994=CIRCLE ( 'NONE', #8481, 19.11328065563151668 ) ;
#2995=EDGE_CURVE ( 'NONE', #12838, #21713, #1441, .T. ) ;
#3000=EDGE_CURVE ( 'NONE', #13430, #14951, #3285, .T. ) ;
#3002=CARTESIAN_POINT ( 'NONE',  ( 14.29266125237896290, -28.07080038625095497, 3.000000000000002665 ) ) ;
#3005=CARTESIAN_POINT ( 'NONE',  ( -10.01544929272295192, 34.09574698892465250, 3.000000000000057732 ) ) ;
#3011=DIRECTION ( 'NONE',  ( -1.000000000000000000, -1.208970125616077665E-17, 0.000000000000000000 ) ) ;
#3012=FACE_OUTER_BOUND ( 'NONE', #8975, .T. ) ;
#3016=ORIENTED_EDGE ( 'NONE', *, *, #22148, .T. ) ;
#3022=CARTESIAN_POINT ( 'NONE',  ( 30.48934413892778750, -16.99647590252659057, 3.000000000000027089 ) ) ;
#3029=ORIENTED_EDGE ( 'NONE', *, *, #2200, .T. ) ;
#3032=EDGE_CURVE ( 'NONE', #22365, #18209, #4740, .T. ) ;
#3051=ORIENTED_EDGE ( 'NONE', *, *, #3059, .F. ) ;
#3056=CARTESIAN_POINT ( 'NONE',  ( -7.711478842616553919, 31.57187188083510065, 3.000000000000023537 ) ) ;
#3059=EDGE_CURVE ( 'NONE', #10976, #4064, #5463, .T. ) ;
#3061=DIRECTION ( 'NONE',  ( 6.505213034913038160E-19, 3.903127820947822896E-18, 1.000000000000000000 ) ) ;
#3063=CARTESIAN_POINT ( 'NONE',  ( -35.16985127952374057, -10.70799354677395776, -2.800654218530457484 ) ) ;
#3066=AXIS2_PLACEMENT_3D ( 'NONE', #2254, #18053, #415 ) ;
#3070=ORIENTED_EDGE ( 'NONE', *, *, #3966, .F. ) ;
#3071=CARTESIAN_POINT ( 'NONE',  ( 34.13396246814584600, -14.93538271375421900, -2.999999999999971578 ) ) ;
#3075=DIRECTION ( 'NONE',  ( 1.000000000000000000, 0.000000000000000000, 0.000000000000000000 ) ) ;
#3078=ORIENTED_EDGE ( 'NONE', *, *, #21368, .F. ) ;
#3084=DIRECTION ( 'NONE',  ( -6.505213034913038160E-19, -3.903127820947822896E-18, -1.000000000000000000 ) ) ;
#3086=FACE_OUTER_BOUND ( 'NONE', #6443, .T. ) ;
#3089=CIRCLE ( 'NONE', #18441, 0.9999999999999995559 ) ;
#3099=DIRECTION ( 'NONE',  ( -1.000000000000000000, 0.000000000000000000, 0.000000000000000000 ) ) ;
#3100=CARTESIAN_POINT ( 'NONE',  ( -17.86915608785656673, 27.01645732367835606, -6.999999999999992006 ) ) ;
#3105=EDGE_CURVE ( 'NONE', #22237, #10740, #7294, .T. ) ;
#3108=ORIENTED_EDGE ( 'NONE', *, *, #11411, .F. ) ;
#3110=CARTESIAN_POINT ( 'NONE',  ( 34.88850421923997658, -1.128083539116281342, -2.999999999999971578 ) ) ;
#3113=CARTESIAN_POINT ( 'NONE',  ( 20.00000000000041211, -2.750597533486379899E-14, -2.999999999999971578 ) ) ;
#3116=CARTESIAN_POINT ( 'NONE',  ( -32.20238537491798780, -4.080045426412992171, 2.999999999999995559 ) ) ;
#3118=LINE ( 'NONE', #13625, #20025 ) ;
#3119=DIRECTION ( 'NONE',  ( 1.000000000000000000, 0.000000000000000000, 0.000000000000000000 ) ) ;
#3120=AXIS2_PLACEMENT_3D ( 'NONE', #7065, #14032, #14149 ) ;
#3123=ORIENTED_EDGE ( 'NONE', *, *, #6032, .F. ) ;
#3126=ORIENTED_EDGE ( 'NONE', *, *, #6887, .T. ) ;
#3127=CARTESIAN_POINT ( 'NONE',  ( 14.74639653023263008, -28.96193690644938101, -2.999999999999971578 ) ) ;
#3133=AXIS2_PLACEMENT_3D ( 'NONE', #1968, #13974, #10551 ) ;
#3135=AXIS2_PLACEMENT_3D ( 'NONE', #4136, #2647, #9289 ) ;
#3137=AXIS2_PLACEMENT_3D ( 'NONE', #6785, #13748, #11817 ) ;
#3141=EDGE_LOOP ( 'NONE', ( #611, #18493, #8514, #2194 ) ) ;
#3144=EDGE_LOOP ( 'NONE', ( #333, #17242, #15002, #10659 ) ) ;
#3145=CARTESIAN_POINT ( 'NONE',  ( -8.485281374238290653, -3.000000000000308198, -4.999999999999997335 ) ) ;
#3153=AXIS2_PLACEMENT_3D ( 'NONE', #8765, #7038, #48 ) ;
#3155=ADVANCED_FACE ( 'NONE', ( #9765 ), #13404, .T. ) ;
#3156=EDGE_LOOP ( 'NONE', ( #15749, #1531, #16740, #19176 ) ) ;
#3172=ORIENTED_EDGE ( 'NONE', *, *, #17176, .F. ) ;
#3175=DIRECTION ( 'NONE',  ( 6.505213034913038160E-19, 3.903127820947822896E-18, 1.000000000000000000 ) ) ;
#3177=EDGE_CURVE ( 'NONE', #9803, #10281, #19587, .T. ) ;
#3179=FACE_OUTER_BOUND ( 'NONE', #192, .T. ) ;
#3182=FACE_OUTER_BOUND ( 'NONE', #18847, .T. ) ;
#3184=CARTESIAN_POINT ( 'NONE',  ( 5.074925817841996256, -32.10132595304126824, -2.999999999999995559 ) ) ;
#3191=FACE_OUTER_BOUND ( 'NONE', #838, .T. ) ;
#3194=CARTESIAN_POINT ( 'NONE',  ( 5.093313992686365310, 32.09841355225992743, -6.999999999999999112 ) ) ;
#3197=EDGE_CURVE ( 'NONE', #22134, #768, #14573, .T. ) ;
#3199=AXIS2_PLACEMENT_3D ( 'NONE', #2389, #7885, #20037 ) ;
#3201=DIRECTION ( 'NONE',  ( 6.505213034913038160E-19, 3.903127820947822896E-18, 1.000000000000000000 ) ) ;
#3203=DIRECTION ( 'NONE',  ( 1.000000000000000000, 0.000000000000000000, 0.000000000000000000 ) ) ;
#3211=AXIS2_PLACEMENT_3D ( 'NONE', #2448, #19517, #21237 ) ;
#3222=CARTESIAN_POINT ( 'NONE',  ( 23.74488952252792728, -25.58633464742643326, 2.999999999999999112 ) ) ;
#3223=DIRECTION ( 'NONE',  ( -6.505213034913038160E-19, -3.903127820947822896E-18, -1.000000000000000000 ) ) ;
#3226=ORIENTED_EDGE ( 'NONE', *, *, #14377, .F. ) ;
#3228=AXIS2_PLACEMENT_3D ( 'NONE', #167, #15857, #7165 ) ;
#3231=CARTESIAN_POINT ( 'NONE',  ( 2.220446049250313081E-13, -2.498001805406602216E-13, -6.859353255829918616 ) ) ;
#3232=CARTESIAN_POINT ( 'NONE',  ( 32.10132595304135350, 5.074925817841719144, -7.000000000000006217 ) ) ;
#3234=CARTESIAN_POINT ( 'NONE',  ( -32.35999952201571972, 1.423424233832654151, -7.000000000000006217 ) ) ;
#3235=ORIENTED_EDGE ( 'NONE', *, *, #6400, .T. ) ;
#3236=DIRECTION ( 'NONE',  ( -1.000000000000000000, -1.208970125616077665E-17, 0.000000000000000000 ) ) ;
#3237=CARTESIAN_POINT ( 'NONE',  ( -27.19760187735852242, -24.73600648735135721, 2.800654218530492123 ) ) ;
#3241=DIRECTION ( 'NONE',  ( 1.000000000000000000, 0.000000000000000000, 0.000000000000000000 ) ) ;
#3245=CARTESIAN_POINT ( 'NONE',  ( -36.75746821813305587, 0.6841746959065087008, -1.999999999999977573 ) ) ;
#3246=AXIS2_PLACEMENT_3D ( 'NONE', #3071, #10042, #18882 ) ;
#3247=ORIENTED_EDGE ( 'NONE', *, *, #19252, .F. ) ;
#3249=LINE ( 'NONE', #17207, #18456 ) ;
#3250=ORIENTED_EDGE ( 'NONE', *, *, #5660, .T. ) ;
#3251=CARTESIAN_POINT ( 'NONE',  ( 31.47514467962671247, -17.79500259159635078, 2.932460736555848602 ) ) ;
#3255=CARTESIAN_POINT ( 'NONE',  ( -31.57187188083505802, -7.711478842616608986, -2.999999999999971578 ) ) ;
#3256=AXIS2_PLACEMENT_3D ( 'NONE', #9401, #16378, #14650 ) ;
#3263=DIRECTION ( 'NONE',  ( -6.505213034913038160E-19, -3.903127820947822896E-18, -1.000000000000000000 ) ) ;
#3268=VERTEX_POINT ( 'NONE', #6900 ) ;
#3271=ORIENTED_EDGE ( 'NONE', *, *, #14496, .F. ) ;
#3276=CARTESIAN_POINT ( 'NONE',  ( -32.20238537491819386, -4.080045426413020593, -2.999999999999975131 ) ) ;
#3277=EDGE_LOOP ( 'NONE', ( #1288, #13989, #378, #15264, #15144, #18553 ) ) ;
#3278=DIRECTION ( 'NONE',  ( -1.000000000000000000, 0.000000000000000000, 0.000000000000000000 ) ) ;
#3285=CIRCLE ( 'NONE', #2540, 34.90673715956759082 ) ;
#3286=CARTESIAN_POINT ( 'NONE',  ( -20.17230487860815913, -25.34312177887351680, -2.999999999999995559 ) ) ;
#3288=ORIENTED_EDGE ( 'NONE', *, *, #19075, .F. ) ;
#3290=ORIENTED_EDGE ( 'NONE', *, *, #2954, .F. ) ;
#3293=DIRECTION ( 'NONE',  ( -1.000000000000000000, -1.208970125616063644E-17, 0.000000000000000000 ) ) ;
#3299=ADVANCED_FACE ( 'NONE', ( #22261 ), #20829, .T. ) ;
#3301=CARTESIAN_POINT ( 'NONE',  ( -34.64554704988852052, -10.35112103033883812, -2.932164912090537534 ) ) ;
#3304=DIRECTION ( 'NONE',  ( 1.000000000000000000, 0.000000000000000000, 0.000000000000000000 ) ) ;
#3306=AXIS2_PLACEMENT_3D ( 'NONE', #14186, #21200, #12471 ) ;
#3312=FACE_OUTER_BOUND ( 'NONE', #20333, .T. ) ;
#3315=CARTESIAN_POINT ( 'NONE',  ( -31.92986134326225667, 18.22261011550274645, 2.800654218530509443 ) ) ;
#3319=EDGE_CURVE ( 'NONE', #14813, #6131, #1064, .T. ) ;
#3320=ORIENTED_EDGE ( 'NONE', *, *, #9372, .T. ) ;
#3321=CARTESIAN_POINT ( 'NONE',  ( 5.551115123125782702E-14, -1.387778780781445676E-13, -5.749999999999949374 ) ) ;
#3322=TOROIDAL_SURFACE ( 'NONE', #16104, 34.90673715956759082, 8.750000000000000000 ) ;
#3323=CARTESIAN_POINT ( 'NONE',  ( 2.775557561562891351E-14, -2.775557561562891351E-14, 2.999999999999999112 ) ) ;
#3324=EDGE_CURVE ( 'NONE', #19833, #16523, #17891, .T. ) ;
#3326=DIRECTION ( 'NONE',  ( 1.000000000000000000, 0.000000000000000000, 0.000000000000000000 ) ) ;
#3337=CARTESIAN_POINT ( 'NONE',  ( -35.28654656445755933, -4.153516728484126119, 3.000000000000047962 ) ) ;
#3341=CARTESIAN_POINT ( 'NONE',  ( 16.56444186175090749, -26.79308242454919764, -2.999999999999999112 ) ) ;
#3344=ORIENTED_EDGE ( 'NONE', *, *, #4142, .F. ) ;
#3345=DIRECTION ( 'NONE',  ( 6.505213034913038160E-19, 3.903127820947822896E-18, 1.000000000000000000 ) ) ;
#3349=ORIENTED_EDGE ( 'NONE', *, *, #2294, .T. ) ;
#3350=DIRECTION ( 'NONE',  ( 6.505213034913038160E-19, 3.903127820947822896E-18, 1.000000000000000000 ) ) ;
#3352=ORIENTED_EDGE ( 'NONE', *, *, #18266, .T. ) ;
#3354=ADVANCED_FACE ( 'NONE', ( #1738 ), #13520, .T. ) ;
#3359=EDGE_LOOP ( 'NONE', ( #5325, #9602, #14619, #14769 ) ) ;
#3371=VERTEX_POINT ( 'NONE', #13961 ) ;
#3376=EDGE_CURVE ( 'NONE', #3870, #9197, #12264, .T. ) ;
#3377=VECTOR ( 'NONE', #581, 1000.000000000000000 ) ;
#3379=VERTEX_POINT ( 'NONE', #22376 ) ;
#3389=B_SPLINE_CURVE_WITH_KNOTS ( 'NONE', 3,
 ( #11603, #16418, #21695, #6448 ),
 .UNSPECIFIED., .F., .F.,
 ( 4, 4 ),
 ( 0.001893031756885525489, 0.003808480026563626671 ),
 .UNSPECIFIED. ) ;
#3391=DIRECTION ( 'NONE',  ( 6.505213034913038160E-19, 3.903127820947822896E-18, 1.000000000000000000 ) ) ;
#3393=CARTESIAN_POINT ( 'NONE',  ( 22.22891329980544839, -23.65408649739131164, 3.000000000000023537 ) ) ;
#3394=EDGE_CURVE ( 'NONE', #10477, #4282, #13621, .T. ) ;
#3417=DIRECTION ( 'NONE',  ( -6.505213034913038160E-19, -3.903127820947822896E-18, -1.000000000000000000 ) ) ;
#3421=AXIS2_PLACEMENT_3D ( 'NONE', #7622, #19663, #2127 ) ;
#3422=ORIENTED_EDGE ( 'NONE', *, *, #2861, .T. ) ;
#3424=AXIS2_PLACEMENT_3D ( 'NONE', #2687, #8176, #22160 ) ;
#3426=DIRECTION ( 'NONE',  ( -6.505213034913038160E-19, -3.903127820947822896E-18, -1.000000000000000000 ) ) ;
#3427=DIRECTION ( 'NONE',  ( -1.000000000000000000, 0.000000000000000000, 0.000000000000000000 ) ) ;
#3428=ORIENTED_EDGE ( 'NONE', *, *, #1467, .T. ) ;
#3434=CARTESIAN_POINT ( 'NONE',  ( -33.52953626616041305, -9.708269511265326557, -2.999999999999971578 ) ) ;
#3438=DIRECTION ( 'NONE',  ( 1.000000000000000000, 0.000000000000000000, 0.000000000000000000 ) ) ;
#3440=CARTESIAN_POINT ( 'NONE',  ( -27.01645732367838448, -17.86915608785691489, 2.999999999999995559 ) ) ;
#3445=ORIENTED_EDGE ( 'NONE', *, *, #21208, .F. ) ;
#3447=DIRECTION ( 'NONE',  ( 6.505213034913038160E-19, 3.903127820947822896E-18, 1.000000000000000000 ) ) ;
#3448=EDGE_CURVE ( 'NONE', #12800, #13841, #11298, .T. ) ;
#3449=EDGE_CURVE ( 'NONE', #17215, #17302, #14201, .T. ) ;
#3451=ORIENTED_EDGE ( 'NONE', *, *, #8194, .F. ) ;
#3453=EDGE_CURVE ( 'NONE', #19820, #11397, #21540, .T. ) ;
#3458=DIRECTION ( 'NONE',  ( -6.505213034913038160E-19, -3.903127820947822896E-18, -1.000000000000000000 ) ) ;
#3464=CARTESIAN_POINT ( 'NONE',  ( 22.98755168577423902, 22.97438720605746099, -2.999999999999971578 ) ) ;
#3469=CARTESIAN_POINT ( 'NONE',  ( 4.171001175319766219, 35.79662727779869869, -2.999999999999992450 ) ) ;
#3470=DIRECTION ( 'NONE',  ( 6.505213034913038160E-19, 3.903127820947822896E-18, 1.000000000000000000 ) ) ;
#3472=FACE_OUTER_BOUND ( 'NONE', #13417, .T. ) ;
#3476=DIRECTION ( 'NONE',  ( 6.505213034913038160E-19, 3.903127820947822896E-18, 1.000000000000000000 ) ) ;
#3477=FACE_OUTER_BOUND ( 'NONE', #6339, .T. ) ;
#3478=DIRECTION ( 'NONE',  ( -1.000000000000000000, 0.000000000000000000, 0.000000000000000000 ) ) ;
#3479=B_SPLINE_CURVE_WITH_KNOTS ( 'NONE', 3,
 ( #8703, #8475, #22242, #12140 ),
 .UNSPECIFIED., .F., .F.,
 ( 4, 4 ),
 ( 9.545285770338856966E-07, 0.001900595205834574144 ),
 .UNSPECIFIED. ) ;
#3480=ORIENTED_EDGE ( 'NONE', *, *, #19931, .F. ) ;
#3481=ADVANCED_FACE ( 'NONE', ( #2182 ), #12706, .T. ) ;
#3493=ORIENTED_EDGE ( 'NONE', *, *, #14239, .T. ) ;
#3498=ORIENTED_EDGE ( 'NONE', *, *, #5104, .F. ) ;
#3502=CIRCLE ( 'NONE', #16280, 31.50000000000000711 ) ;
#3505=AXIS2_PLACEMENT_3D ( 'NONE', #19466, #7315, #8913 ) ;
#3506=CARTESIAN_POINT ( 'NONE',  ( 0.6841746959068417677, 36.75746821813288534, -1.999999999999977573 ) ) ;
#3510=EDGE_LOOP ( 'NONE', ( #719, #13213, #13948, #8055 ) ) ;
#3512=ORIENTED_EDGE ( 'NONE', *, *, #1374, .T. ) ;
#3514=VECTOR ( 'NONE', #14344, 1000.000000000000000 ) ;
#3516=CARTESIAN_POINT ( 'NONE',  ( 28.88846368933348074, 19.59430950039314823, 2.999999999999995559 ) ) ;
#3533=DIRECTION ( 'NONE',  ( -1.000000000000000000, 0.000000000000000000, 0.000000000000000000 ) ) ;
#3537=EDGE_CURVE ( 'NONE', #7411, #10689, #12893, .T. ) ;
#3538=CARTESIAN_POINT ( 'NONE',  ( -27.84804035626028806, 24.75236754129139882, 2.999999999999995559 ) ) ;
#3543=ORIENTED_EDGE ( 'NONE', *, *, #22437, .F. ) ;
#3549=DIRECTION ( 'NONE',  ( -6.505213034913038160E-19, -3.903127820947822896E-18, -1.000000000000000000 ) ) ;
#3557=DIRECTION ( 'NONE',  ( -6.505213034913038160E-19, -3.903127820947822896E-18, -1.000000000000000000 ) ) ;
#3566=ORIENTED_EDGE ( 'NONE', *, *, #15790, .F. ) ;
#3569=CIRCLE ( 'NONE', #16363, 19.11328065563152379 ) ;
#3576=CARTESIAN_POINT ( 'NONE',  ( -26.10603996529605553, -24.10117729468409209, 3.000000000000057732 ) ) ;
#3578=ADVANCED_FACE ( 'NONE', ( #7679 ), #21660, .T. ) ;
#3580=AXIS2_PLACEMENT_3D ( 'NONE', #16373, #5950, #19932 ) ;
#3582=CARTESIAN_POINT ( 'NONE',  ( 24.62019382530525391, -4.341204441673101933, -2.999999999999999112 ) ) ;
#3587=DIRECTION ( 'NONE',  ( -6.505213034913038160E-19, -3.903127820947822896E-18, -1.000000000000000000 ) ) ;
#3591=CIRCLE ( 'NONE', #9793, 19.11328065563152379 ) ;
#3593=FACE_OUTER_BOUND ( 'NONE', #1491, .T. ) ;
#3594=EDGE_CURVE ( 'NONE', #2221, #3795, #10326, .T. ) ;
#3597=AXIS2_PLACEMENT_3D ( 'NONE', #1510, #21098, #5291 ) ;
#3599=ADVANCED_FACE ( 'NONE', ( #4366 ), #13245, .T. ) ;
#3602=ADVANCED_FACE ( 'NONE', ( #16841 ), #20167, .F. ) ;
#3604=VERTEX_POINT ( 'NONE', #13376 ) ;
#3605=FACE_OUTER_BOUND ( 'NONE', #3141, .T. ) ;
#3607=CARTESIAN_POINT ( 'NONE',  ( 27.62019382530527878, -4.341204441673157888, 3.000000000000023537 ) ) ;
#3608=CARTESIAN_POINT ( 'NONE',  ( 7.474202570536298218, -30.60042966911724704, 2.999999999999995559 ) ) ;
#3609=VECTOR ( 'NONE', #18766, 1000.000000000000000 ) ;
#3611=CARTESIAN_POINT ( 'NONE',  ( 30.13956425491254265, 21.05198877411773495, 2.800654218530485018 ) ) ;
#3613=ORIENTED_EDGE ( 'NONE', *, *, #19693, .T. ) ;
#3627=CIRCLE ( 'NONE', #7999, 1.000000000000000888 ) ;
#3628=AXIS2_PLACEMENT_3D ( 'NONE', #20536, #22486, #17081 ) ;
#3629=ORIENTED_EDGE ( 'NONE', *, *, #13058, .F. ) ;
#3630=AXIS2_PLACEMENT_3D ( 'NONE', #10820, #12875, #6021 ) ;
#3636=DIRECTION ( 'NONE',  ( 1.000000000000000000, 1.208970125616063490E-17, 0.000000000000000000 ) ) ;
#3638=CARTESIAN_POINT ( 'NONE',  ( -9.999999999999980460, -3.000000000000002665, 4.999999999999997335 ) ) ;
#3639=FACE_OUTER_BOUND ( 'NONE', #22407, .T. ) ;
#3643=CARTESIAN_POINT ( 'NONE',  ( 2.775557561562891351E-14, -2.775557561562891351E-14, 2.999999999999995559 ) ) ;
#3647=CARTESIAN_POINT ( 'NONE',  ( 35.99819890246980236, -7.463862311151397755, -2.800654218530467698 ) ) ;
#3649=EDGE_CURVE ( 'NONE', #22210, #15922, #4122, .T. ) ;
#3660=DIRECTION ( 'NONE',  ( -1.000000000000000000, -1.208970125616046080E-17, 6.505213034913038160E-19 ) ) ;
#3662=EDGE_CURVE ( 'NONE', #2563, #10262, #11070, .T. ) ;
#3665=CARTESIAN_POINT ( 'NONE',  ( 35.16985127952396084, 10.70799354677376414, 2.800654218530485018 ) ) ;
#3672=( LENGTH_UNIT ( ) NAMED_UNIT ( * ) SI_UNIT ( .MILLI., .METRE. ) );
#3679=VERTEX_POINT ( 'NONE', #18675 ) ;
#3680=EDGE_CURVE ( 'NONE', #3268, #11125, #9240, .T. ) ;
#3682=ORIENTED_EDGE ( 'NONE', *, *, #15109, .T. ) ;
#3685=FACE_OUTER_BOUND ( 'NONE', #22154, .T. ) ;
#3687=CARTESIAN_POINT ( 'NONE',  ( -14.74639653023226948, 28.96193690644935259, 2.999999999999995559 ) ) ;
#3689=DIRECTION ( 'NONE',  ( 6.505213034913038160E-19, 3.903127820947822896E-18, 1.000000000000000000 ) ) ;
#3690=DIRECTION ( 'NONE',  ( -1.000000000000000000, -5.863186540146433761E-14, 0.000000000000000000 ) ) ;
#3693=CARTESIAN_POINT ( 'NONE',  ( -24.24871130596435620, 13.99999999999990052, 2.999999999999995559 ) ) ;
#3695=TOROIDAL_SURFACE ( 'NONE', #7328, 34.90673715956759082, 8.750000000000000000 ) ;
#3703=DIRECTION ( 'NONE',  ( 6.505213034913038160E-19, 3.903127820947822896E-18, 1.000000000000000000 ) ) ;
#3707=AXIS2_PLACEMENT_3D ( 'NONE', #7589, #19856, #6215 ) ;
#3709=ORIENTED_EDGE ( 'NONE', *, *, #14294, .F. ) ;
#3710=ORIENTED_EDGE ( 'NONE', *, *, #20129, .T. ) ;
#3712=CARTESIAN_POINT ( 'NONE',  ( 5.551115123125782702E-14, -1.387778780781445676E-13, -5.749999999999949374 ) ) ;
#3715=VERTEX_POINT ( 'NONE', #18327 ) ;
#3716=CARTESIAN_POINT ( 'NONE',  ( 3.330669073875469621E-13, -1.110223024625156540E-13, -2.999999999999971578 ) ) ;
#3719=CARTESIAN_POINT ( 'NONE',  ( -31.11359284679371484, -4.918774254216190300, -7.000000000000006217 ) ) ;
#3721=DIRECTION ( 'NONE',  ( -6.505213034913038160E-19, -3.903127820947822896E-18, -1.000000000000000000 ) ) ;
#3722=VERTEX_POINT ( 'NONE', #2644 ) ;
#3725=FACE_OUTER_BOUND ( 'NONE', #8858, .T. ) ;
#3727=CARTESIAN_POINT ( 'NONE',  ( 15.00354810072215095, -32.89319786336249507, -2.933296326616342764 ) ) ;
#3733=ADVANCED_FACE ( 'NONE', ( #3086 ), #20959, .F. ) ;
#3736=VECTOR ( 'NONE', #15493, 1000.000000000000000 ) ;
#3738=ORIENTED_EDGE ( 'NONE', *, *, #21735, .F. ) ;
#3743=EDGE_CURVE ( 'NONE', #14737, #4123, #16934, .T. ) ;
#3746=ORIENTED_EDGE ( 'NONE', *, *, #11418, .T. ) ;
#3748=CARTESIAN_POINT ( 'NONE',  ( 32.28023859650885186, 14.85562396683469544, -2.999999999999997780 ) ) ;
#3753=CIRCLE ( 'NONE', #16546, 34.90673715956759082 ) ;
#3755=DIRECTION ( 'NONE',  ( -6.505213034913038160E-19, -3.903127820947822896E-18, -1.000000000000000000 ) ) ;
#3757=EDGE_LOOP ( 'NONE', ( #17591, #3051, #11838, #12422 ) ) ;
#3766=DIRECTION ( 'NONE',  ( -6.505213034913038160E-19, -3.903127820947822896E-18, -1.000000000000000000 ) ) ;
#3768=FACE_OUTER_BOUND ( 'NONE', #9363, .T. ) ;
#3776=AXIS2_PLACEMENT_3D ( 'NONE', #15912, #7336, #230 ) ;
#3777=ORIENTED_EDGE ( 'NONE', *, *, #7700, .F. ) ;
#3779=DIRECTION ( 'NONE',  ( -1.000000000000000000, -7.986889777657331544E-15, 0.000000000000000000 ) ) ;
#3783=ORIENTED_EDGE ( 'NONE', *, *, #22592, .T. ) ;
#3785=EDGE_LOOP ( 'NONE', ( #20669, #19567, #10195, #9967 ) ) ;
#3787=DIRECTION ( 'NONE',  ( -6.505213034913038160E-19, -3.903127820947822896E-18, -1.000000000000000000 ) ) ;
#3788=AXIS2_PLACEMENT_3D ( 'NONE', #4224, #7886, #20151 ) ;
#3792=DIRECTION ( 'NONE',  ( -1.000000000000000000, -1.208970125616044077E-17, 0.000000000000000000 ) ) ;
#3795=VERTEX_POINT ( 'NONE', #20853 ) ;
#3796=DIRECTION ( 'NONE',  ( 6.505213034913038160E-19, 3.903127820947822896E-18, 1.000000000000000000 ) ) ;
#3805=ORIENTED_EDGE ( 'NONE', *, *, #7613, .F. ) ;
#3806=CARTESIAN_POINT ( 'NONE',  ( 2.220446049250313081E-13, 2.775557561562891351E-14, -2.800654218530485018 ) ) ;
#3807=CARTESIAN_POINT ( 'NONE',  ( 34.24928931925771991, -6.742883674876576805, -2.999999999999971578 ) ) ;
#3814=ORIENTED_EDGE ( 'NONE', *, *, #14239, .F. ) ;
#3816=ORIENTED_EDGE ( 'NONE', *, *, #21685, .T. ) ;
#3819=CARTESIAN_POINT ( 'NONE',  ( -30.13956425491219449, -21.05198877411826430, 2.800654218530505890 ) ) ;
#3830=VERTEX_POINT ( 'NONE', #11894 ) ;
#3843=ORIENTED_EDGE ( 'NONE', *, *, #8108, .F. ) ;
#3848=DIRECTION ( 'NONE',  ( 1.000000000000000000, 0.000000000000000000, 0.000000000000000000 ) ) ;
#3852=CARTESIAN_POINT ( 'NONE',  ( -32.09841355225981374, 5.093313992686310243, -7.000000000000006217 ) ) ;
#3857=DIRECTION ( 'NONE',  ( -1.000000000000000000, 0.000000000000000000, 0.000000000000000000 ) ) ;
#3861=CARTESIAN_POINT ( 'NONE',  ( 2.220446049250313081E-13, 2.775557561562891351E-14, -2.800654218530485018 ) ) ;
#3865=DIRECTION ( 'NONE',  ( 6.505213034913038160E-19, 3.903127820947822896E-18, 1.000000000000000000 ) ) ;
#3866=DIRECTION ( 'NONE',  ( -6.505213034913038160E-19, -3.903127820947822896E-18, -1.000000000000000000 ) ) ;
#3869=CIRCLE ( 'NONE', #8977, 34.90673715956759082 ) ;
#3870=VERTEX_POINT ( 'NONE', #17513 ) ;
#3873=VERTEX_POINT ( 'NONE', #1826 ) ;
#3874=EDGE_CURVE ( 'NONE', #10976, #13471, #18753, .T. ) ;
#3876=ORIENTED_EDGE ( 'NONE', *, *, #15734, .F. ) ;
#3879=EDGE_CURVE ( 'NONE', #15473, #8378, #15446, .T. ) ;
#3886=VECTOR ( 'NONE', #22409, 1000.000000000000000 ) ;
#3887=FACE_OUTER_BOUND ( 'NONE', #18134, .T. ) ;
#3888=AXIS2_PLACEMENT_3D ( 'NONE', #9576, #4321, #7743 ) ;
#3895=EDGE_LOOP ( 'NONE', ( #5883, #8008, #16558, #2914 ) ) ;
#3896=ADVANCED_FACE ( 'NONE', ( #5370 ), #7177, .T. ) ;
#3899=CARTESIAN_POINT ( 'NONE',  ( -20.54749497201914465, 29.74882400976386521, 2.932969818539061801 ) ) ;
#3914=CARTESIAN_POINT ( 'NONE',  ( 2.775557561562891351E-14, -2.775557561562891351E-14, 2.999999999999999112 ) ) ;
#3917=EDGE_LOOP ( 'NONE', ( #5908, #632, #4245, #5770 ) ) ;
#3918=CARTESIAN_POINT ( 'NONE',  ( -6.070730550690822902, -31.88709182564697286, -2.999999999999971578 ) ) ;
#3924=LINE ( 'NONE', #21329, #1310 ) ;
#3925=CARTESIAN_POINT ( 'NONE',  ( 18.83615802559796037, -32.14641817400193702, 2.999999999999995559 ) ) ;
#3929=B_SPLINE_CURVE_WITH_KNOTS ( 'NONE', 3,
 ( #19236, #9022, #10503, #17508 ),
 .UNSPECIFIED., .F., .F.,
 ( 4, 4 ),
 ( 9.545285768588289738E-07, 0.001900595205834635509 ),
 .UNSPECIFIED. ) ;
#3933=ORIENTED_EDGE ( 'NONE', *, *, #14294, .T. ) ;
#3939=DIRECTION ( 'NONE',  ( 6.505213034913038160E-19, 3.903127820947822896E-18, 1.000000000000000000 ) ) ;
#3940=DIRECTION ( 'NONE',  ( 1.000000000000000000, 0.000000000000000000, 0.000000000000000000 ) ) ;
#3947=CARTESIAN_POINT ( 'NONE',  ( -18.22261011550271803, -31.92986134326270076, 2.800654218530509443 ) ) ;
#3950=CARTESIAN_POINT ( 'NONE',  ( 34.24928931925771991, -6.742883674876576805, -2.999999999999971578 ) ) ;
#3952=CARTESIAN_POINT ( 'NONE',  ( 14.67611967928950101, -31.67162468656004037, -2.999999999999995559 ) ) ;
#3953=VERTEX_POINT ( 'NONE', #8910 ) ;
#3954=CARTESIAN_POINT ( 'NONE',  ( 32.35999952201606789, -1.423424233832765173, 2.999999999999999112 ) ) ;
#3956=CIRCLE ( 'NONE', #5048, 34.90673715956759082 ) ;
#3958=CARTESIAN_POINT ( 'NONE',  ( -1.423424233832348840, -32.35999952201618157, -6.999999999999992006 ) ) ;
#3959=AXIS2_PLACEMENT_3D ( 'NONE', #16692, #16228, #11072 ) ;
#3966=EDGE_CURVE ( 'NONE', #11046, #17302, #21180, .T. ) ;
#3970=VECTOR ( 'NONE', #19241, 1000.000000000000000 ) ;
#3974=DIRECTION ( 'NONE',  ( 6.505213034913038160E-19, 3.903127820947822896E-18, 1.000000000000000000 ) ) ;
#3977=ADVANCED_FACE ( 'NONE', ( #3768 ), #16007, .T. ) ;
#3978=ORIENTED_EDGE ( 'NONE', *, *, #19823, .T. ) ;
#3979=CARTESIAN_POINT ( 'NONE',  ( 24.41514043009201984, 26.50842683089762986, -2.999999999999947153 ) ) ;
#3981=CARTESIAN_POINT ( 'NONE',  ( -33.46652738560673868, 11.93772187171645172, -3.000000000000015099 ) ) ;
#3983=DIRECTION ( 'NONE',  ( 6.505213034913038160E-19, 3.903127820947822896E-18, 1.000000000000000000 ) ) ;
#3988=CARTESIAN_POINT ( 'NONE',  ( 28.88846368933370456, 19.59430950039303809, -2.999999999999975131 ) ) ;
#3997=CARTESIAN_POINT ( 'NONE',  ( -28.95348479018550236, 14.76298474240492276, -6.999999999999950262 ) ) ;
#4007=DIRECTION ( 'NONE',  ( 1.000000000000000000, 0.000000000000000000, 0.000000000000000000 ) ) ;
#4015=ORIENTED_EDGE ( 'NONE', *, *, #12837, .F. ) ;
#4018=CYLINDRICAL_SURFACE ( 'NONE', #14043, 2.999999999999999112 ) ;
#4019=FACE_OUTER_BOUND ( 'NONE', #22566, .T. ) ;
#4022=EDGE_CURVE ( 'NONE', #2292, #11397, #17795, .T. ) ;
#4030=VECTOR ( 'NONE', #11661, 1000.000000000000000 ) ;
#4036=CARTESIAN_POINT ( 'NONE',  ( 3.330669073875469621E-13, -1.110223024625156540E-13, -2.999999999999971578 ) ) ;
#4037=DIRECTION ( 'NONE',  ( 1.000000000000000000, 1.208970125616063028E-17, 0.000000000000000000 ) ) ;
#4041=LINE ( 'NONE', #9625, #22591 ) ;
#4045=AXIS2_PLACEMENT_3D ( 'NONE', #4585, #14758, #20282 ) ;
#4050=ADVANCED_FACE ( 'NONE', ( #11541 ), #20031, .F. ) ;
#4052=DIRECTION ( 'NONE',  ( 6.505213034913038160E-19, 3.903127820947822896E-18, 1.000000000000000000 ) ) ;
#4060=CARTESIAN_POINT ( 'NONE',  ( -34.74700806321090596, 12.00937115242645170, 2.800654218530481465 ) ) ;
#4062=DIRECTION ( 'NONE',  ( 6.505213034913038160E-19, 3.903127820947822896E-18, 1.000000000000000000 ) ) ;
#4064=VERTEX_POINT ( 'NONE', #18874 ) ;
#4069=DIRECTION ( 'NONE',  ( 1.000000000000000000, 0.000000000000000000, 0.000000000000000000 ) ) ;
#4070=CARTESIAN_POINT ( 'NONE',  ( 14.85562396683509689, -32.28023859650878080, -2.999999999999985789 ) ) ;
#4071=ORIENTED_EDGE ( 'NONE', *, *, #688, .F. ) ;
#4073=DIRECTION ( 'NONE',  ( -1.000000000000000000, -1.208970125616063644E-17, 0.000000000000000000 ) ) ;
#4093=EDGE_CURVE ( 'NONE', #12118, #17505, #9376, .T. ) ;
#4096=DIRECTION ( 'NONE',  ( -1.000000000000000000, -1.788446540656407938E-15, 0.000000000000000000 ) ) ;
#4097=VERTEX_POINT ( 'NONE', #6384 ) ;
#4109=CARTESIAN_POINT ( 'NONE',  ( -25.58633464742622721, -23.74488952252778873, 3.000000000000002665 ) ) ;
#4110=CARTESIAN_POINT ( 'NONE',  ( -35.33352588067073441, -7.094908322883425100, -7.000000000000006217 ) ) ;
#4118=CARTESIAN_POINT ( 'NONE',  ( 27.19760187735889545, 24.73600648735091312, 2.800654218530485018 ) ) ;
#4120=FACE_OUTER_BOUND ( 'NONE', #3156, .T. ) ;
#4122=CIRCLE ( 'NONE', #5234, 28.00000000000000355 ) ;
#4123=VERTEX_POINT ( 'NONE', #19336 ) ;
#4128=DIRECTION ( 'NONE',  ( 1.000000000000000000, 0.000000000000000000, 0.000000000000000000 ) ) ;
#4133=DIRECTION ( 'NONE',  ( -6.505213034913038160E-19, -3.903127820947822896E-18, -1.000000000000000000 ) ) ;
#4135=DIRECTION ( 'NONE',  ( -6.505213034913038160E-19, -3.903127820947822896E-18, -1.000000000000000000 ) ) ;
#4136=CARTESIAN_POINT ( 'NONE',  ( 2.775557561562891351E-14, -2.775557561562891351E-14, 2.999999999999999112 ) ) ;
#4139=CARTESIAN_POINT ( 'NONE',  ( -20.00948735876882623, -24.79619811426206510, -6.999999999999950262 ) ) ;
#4142=EDGE_CURVE ( 'NONE', #4270, #11307, #15950, .T. ) ;
#4144=CIRCLE ( 'NONE', #16935, 31.50000000000000711 ) ;
#4146=VERTEX_POINT ( 'NONE', #14257 ) ;
#4150=EDGE_CURVE ( 'NONE', #5303, #817, #2568, .T. ) ;
#4151=VERTEX_POINT ( 'NONE', #19448 ) ;
#4154=ORIENTED_EDGE ( 'NONE', *, *, #10758, .F. ) ;
#4162=ORIENTED_EDGE ( 'NONE', *, *, #2005, .F. ) ;
#4165=ORIENTED_EDGE ( 'NONE', *, *, #2705, .F. ) ;
#4166=CARTESIAN_POINT ( 'NONE',  ( 2.220446049250313081E-13, -8.326672684688674053E-14, 2.800654218530498785 ) ) ;
#4168=DIRECTION ( 'NONE',  ( 1.000000000000000000, 0.000000000000000000, 0.000000000000000000 ) ) ;
#4169=ORIENTED_EDGE ( 'NONE', *, *, #21574, .F. ) ;
#4171=ORIENTED_EDGE ( 'NONE', *, *, #2028, .F. ) ;
#4174=CYLINDRICAL_SURFACE ( 'NONE', #20983, 1.000000000000000888 ) ;
#4175=ORIENTED_EDGE ( 'NONE', *, *, #13148, .F. ) ;
#4181=CIRCLE ( 'NONE', #6007, 36.76383501243555685 ) ;
#4185=EDGE_LOOP ( 'NONE', ( #15540, #1052, #9663, #13067 ) ) ;
#4186=ORIENTED_EDGE ( 'NONE', *, *, #10227, .T. ) ;
#4189=VERTEX_POINT ( 'NONE', #4288 ) ;
#4194=ORIENTED_EDGE ( 'NONE', *, *, #5415, .F. ) ;
#4200=CARTESIAN_POINT ( 'NONE',  ( 6.070730550691017413, 31.88709182564680589, -2.999999999999995559 ) ) ;
#4204=CARTESIAN_POINT ( 'NONE',  ( 28.73837443790554502, -21.94460005644937439, -2.932164912090501563 ) ) ;
#4205=AXIS2_PLACEMENT_3D ( 'NONE', #9504, #14745, #2634 ) ;
#4207=LINE ( 'NONE', #9480, #22214 ) ;
#4208=ORIENTED_EDGE ( 'NONE', *, *, #10152, .F. ) ;
#4210=VERTEX_POINT ( 'NONE', #68 ) ;
#4213=EDGE_CURVE ( 'NONE', #16878, #10013, #2454, .T. ) ;
#4216=DIRECTION ( 'NONE',  ( 6.505213034913038160E-19, 3.903127820947822896E-18, 1.000000000000000000 ) ) ;
#4219=CARTESIAN_POINT ( 'NONE',  ( -22.97438720605730822, 22.98755168577401520, -7.000000000000006217 ) ) ;
#4221=EDGE_CURVE ( 'NONE', #19293, #16318, #9444, .T. ) ;
#4222=ORIENTED_EDGE ( 'NONE', *, *, #10562, .T. ) ;
#4224=CARTESIAN_POINT ( 'NONE',  ( 5.551115123125782702E-14, -1.387778780781445676E-13, -5.749999999999949374 ) ) ;
#4226=CARTESIAN_POINT ( 'NONE',  ( 35.33352588067128863, 7.094908322883036966, -2.999999999999971578 ) ) ;
#4229=ORIENTED_EDGE ( 'NONE', *, *, #4315, .T. ) ;
#4232=ORIENTED_EDGE ( 'NONE', *, *, #21498, .T. ) ;
#4236=ORIENTED_EDGE ( 'NONE', *, *, #18376, .F. ) ;
#4245=ORIENTED_EDGE ( 'NONE', *, *, #22073, .T. ) ;
#4247=FACE_OUTER_BOUND ( 'NONE', #18799, .T. ) ;
#4249=AXIS2_PLACEMENT_3D ( 'NONE', #17632, #214, #19373 ) ;
#4259=EDGE_LOOP ( 'NONE', ( #21771, #20997, #17156, #9624 ) ) ;
#4262=AXIS2_PLACEMENT_3D ( 'NONE', #17067, #22359, #20622 ) ;
#4265=AXIS2_PLACEMENT_3D ( 'NONE', #16425, #3587, #14665 ) ;
#4266=EDGE_CURVE ( 'NONE', #10013, #6602, #12283, .T. ) ;
#4268=CIRCLE ( 'NONE', #17059, 31.50000000000001421 ) ;
#4270=VERTEX_POINT ( 'NONE', #21045 ) ;
#4274=ORIENTED_EDGE ( 'NONE', *, *, #1725, .T. ) ;
#4275=FACE_OUTER_BOUND ( 'NONE', #4304, .T. ) ;
#4281=DIRECTION ( 'NONE',  ( -1.000000000000000000, -1.208970125616060717E-17, 0.000000000000000000 ) ) ;
#4282=VERTEX_POINT ( 'NONE', #16405 ) ;
#4288=CARTESIAN_POINT ( 'NONE',  ( -27.19760187735867518, -24.73600648735113694, -2.800654218530429507 ) ) ;
#4296=CARTESIAN_POINT ( 'NONE',  ( 2.775557561562891351E-14, -2.775557561562891351E-14, 2.999999999999995559 ) ) ;
#4301=AXIS2_PLACEMENT_3D ( 'NONE', #17686, #19530, #2111 ) ;
#4302=ORIENTED_EDGE ( 'NONE', *, *, #15059, .T. ) ;
#4304=EDGE_LOOP ( 'NONE', ( #13986, #10646, #8167, #15663 ) ) ;
#4305=ADVANCED_FACE ( 'NONE', ( #21681 ), #2207, .F. ) ;
#4307=DIRECTION ( 'NONE',  ( 6.505213034913038160E-19, 3.903127820947822896E-18, 1.000000000000000000 ) ) ;
#4312=LINE ( 'NONE', #19549, #17870 ) ;
#4313=DIRECTION ( 'NONE',  ( -6.505213034913038160E-19, -3.903127820947822896E-18, -1.000000000000000000 ) ) ;
#4314=ORIENTED_EDGE ( 'NONE', *, *, #16557, .F. ) ;
#4315=EDGE_CURVE ( 'NONE', #19421, #728, #21506, .T. ) ;
#4317=ORIENTED_EDGE ( 'NONE', *, *, #22598, .F. ) ;
#4318=CARTESIAN_POINT ( 'NONE',  ( 2.220446049250313081E-13, -2.498001805406602216E-13, -6.859353255829918616 ) ) ;
#4321=DIRECTION ( 'NONE',  ( -6.505213034913038160E-19, -3.903127820947822896E-18, -1.000000000000000000 ) ) ;
#4328=CIRCLE ( 'NONE', #12724, 1.000000000000000888 ) ;
#4329=ORIENTED_EDGE ( 'NONE', *, *, #650, .F. ) ;
#4335=ADVANCED_FACE ( 'NONE', ( #12954 ), #2848, .T. ) ;
#4337=DIRECTION ( 'NONE',  ( 6.505213034913038160E-19, 3.903127820947822896E-18, 1.000000000000000000 ) ) ;
#4338=DIRECTION ( 'NONE',  ( 6.505213034913038160E-19, 3.903127820947822896E-18, 1.000000000000000000 ) ) ;
#4340=CARTESIAN_POINT ( 'NONE',  ( 1.423424233832709662, 32.35999952201570551, -2.999999999999975131 ) ) ;
#4343=CIRCLE ( 'NONE', #8739, 1.000000000000000888 ) ;
#4345=EDGE_CURVE ( 'NONE', #18209, #22365, #13434, .T. ) ;
#4348=CARTESIAN_POINT ( 'NONE',  ( -36.54278193890295512, -4.025500340002762911, -2.800654218530457484 ) ) ;
#4349=CARTESIAN_POINT ( 'NONE',  ( 11.85401191286899980, 32.83234229683715455, 2.999999999999995559 ) ) ;
#4352=CARTESIAN_POINT ( 'NONE',  ( -14.30873905802322632, -28.06260833510309993, -2.999999999999957367 ) ) ;
#4357=AXIS2_PLACEMENT_3D ( 'NONE', #15647, #1338, #20483 ) ;
#4362=CARTESIAN_POINT ( 'NONE',  ( -4.104665049622623130, 35.91964150878174422, -2.933296326616367189 ) ) ;
#4363=VERTEX_POINT ( 'NONE', #12498 ) ;
#4366=FACE_OUTER_BOUND ( 'NONE', #20936, .T. ) ;
#4368=DIRECTION ( 'NONE',  ( 1.000000000000000000, 8.005695478557271943E-15, 0.000000000000000000 ) ) ;
#4370=DIRECTION ( 'NONE',  ( -6.505213034913038160E-19, -3.903127820947822896E-18, -1.000000000000000000 ) ) ;
#4372=ORIENTED_EDGE ( 'NONE', *, *, #8821, .F. ) ;
#4373=DIRECTION ( 'NONE',  ( -6.505213034913038160E-19, -3.903127820947822896E-18, -1.000000000000000000 ) ) ;
#4374=CARTESIAN_POINT ( 'NONE',  ( -10.70799354677358295, 35.16985127952384715, -2.800654218530457484 ) ) ;
#4384=ORIENTED_EDGE ( 'NONE', *, *, #17438, .F. ) ;
#4385=ORIENTED_EDGE ( 'NONE', *, *, #11163, .T. ) ;
#4388=CARTESIAN_POINT ( 'NONE',  ( 24.73600648735135721, -27.19760187735878532, 2.800654218530481465 ) ) ;
#4391=ORIENTED_EDGE ( 'NONE', *, *, #9058, .F. ) ;
#4393=CARTESIAN_POINT ( 'NONE',  ( 30.33632613426201630, -11.35354668330712613, 2.999999999999995559 ) ) ;
#4397=AXIS2_PLACEMENT_3D ( 'NONE', #15235, #13516, #18698 ) ;
#4405=CARTESIAN_POINT ( 'NONE',  ( 27.62019382530525391, -4.341204441673157888, -5.000000000000004441 ) ) ;
#4408=AXIS2_PLACEMENT_3D ( 'NONE', #21234, #14219, #12501 ) ;
#4410=DIRECTION ( 'NONE',  ( -1.000000000000000000, -4.975008120446308529E-14, 0.000000000000000000 ) ) ;
#4415=AXIS2_PLACEMENT_3D ( 'NONE', #10171, #3084, #22115 ) ;
#4417=ORIENTED_EDGE ( 'NONE', *, *, #21829, .F. ) ;
#4419=CARTESIAN_POINT ( 'NONE',  ( -14.14132741310371344, -16.85297774861763287, 2.999999999999995559 ) ) ;
#4422=CYLINDRICAL_SURFACE ( 'NONE', #12020, 1.000000000000000888 ) ;
#4428=LINE ( 'NONE', #20124, #18146 ) ;
#4440=EDGE_CURVE ( 'NONE', #4746, #877, #19324, .T. ) ;
#4441=ORIENTED_EDGE ( 'NONE', *, *, #1644, .F. ) ;
#4443=DIRECTION ( 'NONE',  ( 1.000000000000000000, 0.000000000000000000, 0.000000000000000000 ) ) ;
#4448=CARTESIAN_POINT ( 'NONE',  ( 2.775557561562891351E-14, -2.775557561562891351E-14, 2.999999999999999112 ) ) ;
#4451=CARTESIAN_POINT ( 'NONE',  ( 35.99819890246974552, -7.463862311151231665, 2.800654218530509443 ) ) ;
#4459=EDGE_LOOP ( 'NONE', ( #11575, #5939, #8184, #6790, #21741, #20951 ) ) ;
#4460=FACE_OUTER_BOUND ( 'NONE', #17382, .T. ) ;
#4465=ADVANCED_FACE ( 'NONE', ( #4275 ), #14894, .F. ) ;
#4468=AXIS2_PLACEMENT_3D ( 'NONE', #808, #4370, #4477 ) ;
#4470=DIRECTION ( 'NONE',  ( -1.000000000000000000, 1.815202222194848473E-15, 0.000000000000000000 ) ) ;
#4472=CARTESIAN_POINT ( 'NONE',  ( 15.02862401740806497, 32.75570538720773328, -2.999999999999999112 ) ) ;
#4473=DIRECTION ( 'NONE',  ( -1.000000000000000000, 0.000000000000000000, 0.000000000000000000 ) ) ;
#4474=CYLINDRICAL_SURFACE ( 'NONE', #14916, 1.000000000000000888 ) ;
#4476=DIRECTION ( 'NONE',  ( 6.505213034913038160E-19, 3.903127820947822896E-18, 1.000000000000000000 ) ) ;
#4477=DIRECTION ( 'NONE',  ( -1.000000000000000000, 0.000000000000000000, 0.000000000000000000 ) ) ;
#4478=VERTEX_POINT ( 'NONE', #9643 ) ;
#4484=CARTESIAN_POINT ( 'NONE',  ( -4.025500340002513333, 36.54278193890309012, -2.800654218530457484 ) ) ;
#4485=EDGE_CURVE ( 'NONE', #12526, #1555, #22018, .T. ) ;
#4486=AXIS2_PLACEMENT_3D ( 'NONE', #14247, #21262, #5553 ) ;
#4487=DIRECTION ( 'NONE',  ( 1.000000000000000000, 1.208970125616053784E-17, 0.000000000000000000 ) ) ;
#4489=ORIENTED_EDGE ( 'NONE', *, *, #17376, .T. ) ;
#4492=ORIENTED_EDGE ( 'NONE', *, *, #9847, .T. ) ;
#4494=DIRECTION ( 'NONE',  ( -6.505213034913038160E-19, -3.903127820947822896E-18, -1.000000000000000000 ) ) ;
#4501=DIRECTION ( 'NONE',  ( 1.000000000000000000, 1.208970125616053475E-17, 0.000000000000000000 ) ) ;
#4502=CARTESIAN_POINT ( 'NONE',  ( 32.10132595304146719, 5.074925817841635656, 2.999999999999995559 ) ) ;
#4504=DIRECTION ( 'NONE',  ( 6.505213034913038160E-19, 3.903127820947822896E-18, 1.000000000000000000 ) ) ;
#4506=EDGE_CURVE ( 'NONE', #817, #4626, #1880, .T. ) ;
#4508=DIRECTION ( 'NONE',  ( -1.000000000000000000, 0.000000000000000000, 0.000000000000000000 ) ) ;
#4509=CARTESIAN_POINT ( 'NONE',  ( 11.35354668330723626, 30.33632613426176405, 2.999999999999999112 ) ) ;
#4513=ORIENTED_EDGE ( 'NONE', *, *, #2005, .T. ) ;
#4524=CONICAL_SURFACE ( 'NONE', #5254, 18.00000000000000000, 0.7853981633974540522 ) ;
#4527=EDGE_CURVE ( 'NONE', #11599, #11128, #5194, .T. ) ;
#4528=ORIENTED_EDGE ( 'NONE', *, *, #18625, .F. ) ;
#4530=CYLINDRICAL_SURFACE ( 'NONE', #7774, 1.000000000000001776 ) ;
#4531=DIRECTION ( 'NONE',  ( -6.505213034913038160E-19, -3.903127820947822896E-18, -1.000000000000000000 ) ) ;
#4535=DIRECTION ( 'NONE',  ( 6.505213034913038160E-19, 3.903127820947822896E-18, 1.000000000000000000 ) ) ;
#4541=DIRECTION ( 'NONE',  ( 6.505213034913038160E-19, 3.903127820947822896E-18, 1.000000000000000000 ) ) ;
#4544=DIRECTION ( 'NONE',  ( -1.000000000000000000, 0.000000000000000000, 0.000000000000000000 ) ) ;
#4549=CARTESIAN_POINT ( 'NONE',  ( 28.96193690644943786, 14.74639653023224284, -2.999999999999971578 ) ) ;
#4550=ORIENTED_EDGE ( 'NONE', *, *, #20384, .F. ) ;
#4556=CARTESIAN_POINT ( 'NONE',  ( -30.48934413892778750, 16.99647590252656570, 2.999999999999999112 ) ) ;
#4557=CARTESIAN_POINT ( 'NONE',  ( -31.57187188083528184, -7.711478842616553919, 3.000000000000023537 ) ) ;
#4559=ADVANCED_FACE ( 'NONE', ( #20529 ), #1615, .F. ) ;
#4561=CIRCLE ( 'NONE', #20298, 0.9999999999999995559 ) ;
#4563=B_SPLINE_CURVE_WITH_KNOTS ( 'NONE', 3,
 ( #3022, #13418, #3251, #16983 ),
 .UNSPECIFIED., .F., .F.,
 ( 4, 4 ),
 ( 0.001875451646902537165, 0.003761979286330901194 ),
 .UNSPECIFIED. ) ;
#4565=CARTESIAN_POINT ( 'NONE',  ( 3.330669073875469621E-13, -1.110223024625156540E-13, -2.999999999999971578 ) ) ;
#4570=EDGE_CURVE ( 'NONE', #10093, #17988, #8770, .T. ) ;
#4577=CARTESIAN_POINT ( 'NONE',  ( -35.16985127952396084, -10.70799354677381920, -1.999999999999977573 ) ) ;
#4578=CARTESIAN_POINT ( 'NONE',  ( 34.09574698892499356, 10.01544929272282580, 3.000000000000049294 ) ) ;
#4579=EDGE_CURVE ( 'NONE', #13430, #14737, #15040, .T. ) ;
#4585=CARTESIAN_POINT ( 'NONE',  ( 36.39375341857542878, 7.980461308159686240, 2.999999999999995559 ) ) ;
#4587=CARTESIAN_POINT ( 'NONE',  ( 31.57187188083529605, 7.711478842616553919, -2.999999999999999112 ) ) ;
#4588=AXIS2_PLACEMENT_3D ( 'NONE', #18485, #2801, #1081 ) ;
#4590=EDGE_CURVE ( 'NONE', #4760, #11286, #21636, .T. ) ;
#4593=CARTESIAN_POINT ( 'NONE',  ( 7.463862311151453710, 35.99819890246924814, -1.999999999999977573 ) ) ;
#4594=ORIENTED_EDGE ( 'NONE', *, *, #1472, .T. ) ;
#4595=CARTESIAN_POINT ( 'NONE',  ( -34.13396246814566837, 14.93538271375399695, 2.999999999999995559 ) ) ;
#4600=ORIENTED_EDGE ( 'NONE', *, *, #13929, .F. ) ;
#4603=CARTESIAN_POINT ( 'NONE',  ( 3.330669073875469621E-13, -1.110223024625156540E-13, -2.999999999999971578 ) ) ;
#4607=ORIENTED_EDGE ( 'NONE', *, *, #12288, .F. ) ;
#4617=VERTEX_POINT ( 'NONE', #2615 ) ;
#4623=CARTESIAN_POINT ( 'NONE',  ( -32.09841355225989901, 5.093313992686310243, -2.999999999999971578 ) ) ;
#4626=VERTEX_POINT ( 'NONE', #11420 ) ;
#4628=CYLINDRICAL_SURFACE ( 'NONE', #7641, 0.9999999999999974465 ) ;
#4636=EDGE_CURVE ( 'NONE', #8959, #5811, #14744, .T. ) ;
#4641=EDGE_LOOP ( 'NONE', ( #15439, #20247, #4886, #22099 ) ) ;
#4646=FACE_OUTER_BOUND ( 'NONE', #14126, .T. ) ;
#4669=LINE ( 'NONE', #6490, #12538 ) ;
#4670=AXIS2_PLACEMENT_3D ( 'NONE', #2784, #11811, #16970 ) ;
#4671=AXIS2_PLACEMENT_3D ( 'NONE', #20316, #4504, #1281 ) ;
#4672=CYLINDRICAL_SURFACE ( 'NONE', #13825, 36.76383501243555685 ) ;
#4674=AXIS2_PLACEMENT_3D ( 'NONE', #3323, #8236, #22343 ) ;
#4677=LINE ( 'NONE', #19834, #8370 ) ;
#4678=CARTESIAN_POINT ( 'NONE',  ( -32.09841355225970005, 5.093313992686226754, 2.999999999999995559 ) ) ;
#4679=CARTESIAN_POINT ( 'NONE',  ( 31.67162468656012209, 14.67611967928900185, 3.000000000000002665 ) ) ;
#4680=DIRECTION ( 'NONE',  ( -6.505213034913038160E-19, -3.903127820947822896E-18, -1.000000000000000000 ) ) ;
#4683=ORIENTED_EDGE ( 'NONE', *, *, #13505, .T. ) ;
#4684=LINE ( 'NONE', #4795, #4030 ) ;
#4691=CARTESIAN_POINT ( 'NONE',  ( 15.02862401740828702, 32.75570538720756986, -6.999999999999950262 ) ) ;
#4692=ADVANCED_FACE ( 'NONE', ( #14957 ), #17607, .T. ) ;
#4698=VECTOR ( 'NONE', #4823, 1000.000000000000000 ) ;
#4699=DIRECTION ( 'NONE',  ( 6.505213034913038160E-19, 3.903127820947822896E-18, 1.000000000000000000 ) ) ;
#4700=VERTEX_POINT ( 'NONE', #20369 ) ;
#4701=CIRCLE ( 'NONE', #17494, 19.11328065563152379 ) ;
#4703=CYLINDRICAL_SURFACE ( 'NONE', #8427, 19.11328065563150957 ) ;
#4705=DIRECTION ( 'NONE',  ( -6.505213034913038160E-19, -3.903127820947822896E-18, -1.000000000000000000 ) ) ;
#4713=FACE_OUTER_BOUND ( 'NONE', #20639, .T. ) ;
#4718=VECTOR ( 'NONE', #12540, 1000.000000000000000 ) ;
#4719=CARTESIAN_POINT ( 'NONE',  ( -6.955395936296827841, -34.84717828836198805, -2.999999999999982236 ) ) ;
#4727=ADVANCED_FACE ( 'NONE', ( #3179 ), #15176, .F. ) ;
#4735=CARTESIAN_POINT ( 'NONE',  ( -9.708269511265271490, 33.52953626616022831, 2.999999999999999112 ) ) ;
#4736=AXIS2_PLACEMENT_3D ( 'NONE', #14611, #21727, #525 ) ;
#4738=ORIENTED_EDGE ( 'NONE', *, *, #6654, .T. ) ;
#4740=CIRCLE ( 'NONE', #20468, 20.00000000000002132 ) ;
#4742=DIRECTION ( 'NONE',  ( -6.505213034913038160E-19, -3.903127820947822896E-18, -1.000000000000000000 ) ) ;
#4746=VERTEX_POINT ( 'NONE', #10945 ) ;
#4751=ORIENTED_EDGE ( 'NONE', *, *, #11528, .T. ) ;
#4757=EDGE_CURVE ( 'NONE', #3371, #18887, #17318, .T. ) ;
#4758=EDGE_CURVE ( 'NONE', #19446, #19435, #2330, .T. ) ;
#4760=VERTEX_POINT ( 'NONE', #9467 ) ;
#4761=ORIENTED_EDGE ( 'NONE', *, *, #18998, .F. ) ;
#4762=CARTESIAN_POINT ( 'NONE',  ( -5.093313992686115732, -32.09841355226039639, -7.000000000000006217 ) ) ;
#4765=VERTEX_POINT ( 'NONE', #17938 ) ;
#4768=VERTEX_POINT ( 'NONE', #7398 ) ;
#4769=CARTESIAN_POINT ( 'NONE',  ( 2.775557561562891351E-14, -2.775557561562891351E-14, 2.999999999999995559 ) ) ;
#4774=CARTESIAN_POINT ( 'NONE',  ( -27.95348479018558763, 14.76298474240492276, 3.000000000000023537 ) ) ;
#4777=AXIS2_PLACEMENT_3D ( 'NONE', #20057, #12923, #16606 ) ;
#4779=VERTEX_POINT ( 'NONE', #7849 ) ;
#4787=AXIS2_PLACEMENT_3D ( 'NONE', #16115, #9024, #2263 ) ;
#4795=CARTESIAN_POINT ( 'NONE',  ( 24.65063509461093361, 12.50000000000006750, -5.000000000000004441 ) ) ;
#4802=AXIS2_PLACEMENT_3D ( 'NONE', #11284, #11395, #18380 ) ;
#4806=DIRECTION ( 'NONE',  ( 6.505213034913038160E-19, 3.903127820947822896E-18, 1.000000000000000000 ) ) ;
#4807=B_SPLINE_CURVE_WITH_KNOTS ( 'NONE', 3,
 ( #15163, #22528, #1437, #15506 ),
 .UNSPECIFIED., .F., .F.,
 ( 4, 4 ),
 ( 0.001893031756885383459, 0.003808480026563708203 ),
 .UNSPECIFIED. ) ;
#4823=DIRECTION ( 'NONE',  ( 6.505213034913038160E-19, 3.903127820947822896E-18, 1.000000000000000000 ) ) ;
#4824=DIRECTION ( 'NONE',  ( 6.505213034913038160E-19, 3.903127820947822896E-18, 1.000000000000000000 ) ) ;
#4825=DIRECTION ( 'NONE',  ( -1.000000000000000000, 0.000000000000000000, 0.000000000000000000 ) ) ;
#4828=ORIENTED_EDGE ( 'NONE', *, *, #1766, .F. ) ;
#4832=DIRECTION ( 'NONE',  ( -6.505213034913038160E-19, -3.903127820947822896E-18, -1.000000000000000000 ) ) ;
#4833=CARTESIAN_POINT ( 'NONE',  ( 7.980461308160213818, -36.39375341857525825, -2.999999999999999112 ) ) ;
#4842=EDGE_CURVE ( 'NONE', #9799, #10690, #2971, .T. ) ;
#4845=AXIS2_PLACEMENT_3D ( 'NONE', #5739, #17767, #352 ) ;
#4847=CYLINDRICAL_SURFACE ( 'NONE', #3137, 19.11328065563151313 ) ;
#4849=DIRECTION ( 'NONE',  ( -6.505213034913038160E-19, -3.903127820947822896E-18, -1.000000000000000000 ) ) ;
#4850=ORIENTED_EDGE ( 'NONE', *, *, #18415, .T. ) ;
#4856=DIRECTION ( 'NONE',  ( -6.505213034913038160E-19, -3.903127820947822896E-18, -1.000000000000000000 ) ) ;
#4858=ORIENTED_EDGE ( 'NONE', *, *, #6484, .T. ) ;
#4859=AXIS2_PLACEMENT_3D ( 'NONE', #7419, #14275, #17961 ) ;
#4860=VERTEX_POINT ( 'NONE', #16555 ) ;
#4861=ADVANCED_FACE ( 'NONE', ( #20005 ), #17823, .T. ) ;
#4864=VECTOR ( 'NONE', #16190, 1000.000000000000000 ) ;
#4875=CARTESIAN_POINT ( 'NONE',  ( 4.080045426412937104, -32.20238537491820807, 2.999999999999995559 ) ) ;
#4879=AXIS2_PLACEMENT_3D ( 'NONE', #17880, #9167, #7447 ) ;
#4881=AXIS2_PLACEMENT_3D ( 'NONE', #18988, #17593, #22542 ) ;
#4883=EDGE_CURVE ( 'NONE', #14834, #22210, #22173, .T. ) ;
#4884=ORIENTED_EDGE ( 'NONE', *, *, #18355, .F. ) ;
#4886=ORIENTED_EDGE ( 'NONE', *, *, #908, .T. ) ;
#4893=FACE_OUTER_BOUND ( 'NONE', #14989, .T. ) ;
#4895=VECTOR ( 'NONE', #13052, 1000.000000000000000 ) ;
#4899=DIRECTION ( 'NONE',  ( -1.000000000000000000, -9.002681209562842834E-16, 0.000000000000000000 ) ) ;
#4902=ORIENTED_EDGE ( 'NONE', *, *, #21257, .F. ) ;
#4903=CARTESIAN_POINT ( 'NONE',  ( 28.95348479018586119, -14.76298474240533842, 3.000000000000023537 ) ) ;
#4909=AXIS2_PLACEMENT_3D ( 'NONE', #19921, #11086, #2515 ) ;
#4910=EDGE_LOOP ( 'NONE', ( #21437, #15265, #15159, #5765 ) ) ;
#4912=ORIENTED_EDGE ( 'NONE', *, *, #19091, .F. ) ;
#4915=DIRECTION ( 'NONE',  ( 6.505213034913038160E-19, 3.903127820947822896E-18, 1.000000000000000000 ) ) ;
#4917=EDGE_CURVE ( 'NONE', #5723, #4700, #5895, .T. ) ;
#4923=AXIS2_PLACEMENT_3D ( 'NONE', #8814, #2046, #7426 ) ;
#4930=ORIENTED_EDGE ( 'NONE', *, *, #12380, .T. ) ;
#4937=ORIENTED_EDGE ( 'NONE', *, *, #1020, .F. ) ;
#4939=AXIS2_PLACEMENT_3D ( 'NONE', #13473, #896, #1010 ) ;
#4941=CARTESIAN_POINT ( 'NONE',  ( 15.00428685838202725, -32.89708536800409178, 2.932460736555828618 ) ) ;
#4944=CARTESIAN_POINT ( 'NONE',  ( 3.608224830031758756E-13, -2.775557561562891351E-14, -4.999999999999997335 ) ) ;
#4945=CIRCLE ( 'NONE', #3066, 19.11328065563151313 ) ;
#4954=CARTESIAN_POINT ( 'NONE',  ( 24.65063509461118230, 12.50000000000006750, -2.999999999999988898 ) ) ;
#4957=ORIENTED_EDGE ( 'NONE', *, *, #19973, .T. ) ;
#4960=ORIENTED_EDGE ( 'NONE', *, *, #6883, .T. ) ;
#4965=CIRCLE ( 'NONE', #17753, 36.76383501243555685 ) ;
#4968=CIRCLE ( 'NONE', #8984, 19.11328065563152023 ) ;
#4971=VERTEX_POINT ( 'NONE', #15155 ) ;
#4979=ORIENTED_EDGE ( 'NONE', *, *, #9058, .T. ) ;
#4982=ORIENTED_EDGE ( 'NONE', *, *, #4221, .F. ) ;
#4985=AXIS2_PLACEMENT_3D ( 'NONE', #3643, #17601, #1907 ) ;
#4988=ORIENTED_EDGE ( 'NONE', *, *, #19505, .T. ) ;
#4991=DIRECTION ( 'NONE',  ( -6.505213034913038160E-19, -3.903127820947822896E-18, -1.000000000000000000 ) ) ;
#4993=FACE_OUTER_BOUND ( 'NONE', #20761, .T. ) ;
#4994=ADVANCED_FACE ( 'NONE', ( #1540 ), #15729, .T. ) ;
#4997=CIRCLE ( 'NONE', #19634, 19.11328065563151668 ) ;
#5000=AXIS2_PLACEMENT_3D ( 'NONE', #3127, #11609, #15369 ) ;
#5001=ORIENTED_EDGE ( 'NONE', *, *, #17328, .F. ) ;
#5003=VERTEX_POINT ( 'NONE', #13988 ) ;
#5006=ORIENTED_EDGE ( 'NONE', *, *, #6978, .F. ) ;
#5008=CIRCLE ( 'NONE', #22582, 1.000000000000000888 ) ;
#5016=FACE_OUTER_BOUND ( 'NONE', #21485, .T. ) ;
#5017=LINE ( 'NONE', #19103, #2776 ) ;
#5018=AXIS2_PLACEMENT_3D ( 'NONE', #8916, #3557, #1832 ) ;
#5021=CARTESIAN_POINT ( 'NONE',  ( -22.98755168577423902, -22.97438720605751783, -6.999999999999950262 ) ) ;
#5022=CARTESIAN_POINT ( 'NONE',  ( 32.35999952201609631, -1.423424233832876196, -6.999999999999999112 ) ) ;
#5025=DIRECTION ( 'NONE',  ( -6.505213034913038160E-19, -3.903127820947822896E-18, -1.000000000000000000 ) ) ;
#5026=CARTESIAN_POINT ( 'NONE',  ( 32.10132595304146719, 5.074925817841635656, -2.999999999999971578 ) ) ;
#5027=DIRECTION ( 'NONE',  ( -1.000000000000000000, 2.141938622189920653E-14, 0.000000000000000000 ) ) ;
#5028=ORIENTED_EDGE ( 'NONE', *, *, #16309, .T. ) ;
#5045=CIRCLE ( 'NONE', #6872, 0.9999999999999974465 ) ;
#5047=DIRECTION ( 'NONE',  ( -6.505213034913038160E-19, -3.903127820947822896E-18, -1.000000000000000000 ) ) ;
#5048=AXIS2_PLACEMENT_3D ( 'NONE', #3914, #17764, #21209 ) ;
#5051=CARTESIAN_POINT ( 'NONE',  ( 7.197698565811989191, 35.43359966464129229, 2.932460736555801972 ) ) ;
#5052=AXIS2_PLACEMENT_3D ( 'NONE', #18777, #13485, #9946 ) ;
#5053=VERTEX_POINT ( 'NONE', #5428 ) ;
#5054=CYLINDRICAL_SURFACE ( 'NONE', #6065, 0.9999999999999974465 ) ;
#5058=AXIS2_PLACEMENT_3D ( 'NONE', #10271, #15535, #22561 ) ;
#5059=ORIENTED_EDGE ( 'NONE', *, *, #17176, .T. ) ;
#5062=AXIS2_PLACEMENT_3D ( 'NONE', #15392, #5113, #20681 ) ;
#5070=DIRECTION ( 'NONE',  ( 6.505213034913038160E-19, 3.903127820947822896E-18, 1.000000000000000000 ) ) ;
#5071=VERTEX_POINT ( 'NONE', #11961 ) ;
#5074=ORIENTED_EDGE ( 'NONE', *, *, #20274, .F. ) ;
#5075=DIRECTION ( 'NONE',  ( 6.505213034913038160E-19, 3.903127820947822896E-18, 1.000000000000000000 ) ) ;
#5077=CARTESIAN_POINT ( 'NONE',  ( 22.22891329980564024, -23.65408649739134006, -2.999999999999971578 ) ) ;
#5081=ORIENTED_EDGE ( 'NONE', *, *, #14388, .F. ) ;
#5082=DIRECTION ( 'NONE',  ( -6.505213034913038160E-19, -3.903127820947822896E-18, -1.000000000000000000 ) ) ;
#5086=ORIENTED_EDGE ( 'NONE', *, *, #15228, .T. ) ;
#5090=CARTESIAN_POINT ( 'NONE',  ( 23.74488952252801255, -25.58633464742643326, -2.999999999999978240 ) ) ;
#5100=EDGE_LOOP ( 'NONE', ( #9016, #2700, #3271, #1805 ) ) ;
#5104=EDGE_CURVE ( 'NONE', #21718, #19773, #20400, .T. ) ;
#5111=ORIENTED_EDGE ( 'NONE', *, *, #4022, .T. ) ;
#5113=DIRECTION ( 'NONE',  ( 6.505213034913038160E-19, 3.903127820947822896E-18, 1.000000000000000000 ) ) ;
#5115=DIRECTION ( 'NONE',  ( -1.000000000000000000, -1.208970125616060101E-17, 6.505213034913038160E-19 ) ) ;
#5116=DIRECTION ( 'NONE',  ( -1.000000000000000000, -1.208970125616060717E-17, 0.000000000000000000 ) ) ;
#5118=CARTESIAN_POINT ( 'NONE',  ( 2.775557561562891351E-14, -2.775557561562891351E-14, 2.999999999999999112 ) ) ;
#5119=CARTESIAN_POINT ( 'NONE',  ( 3.330669073875469621E-13, -1.110223024625156540E-13, -2.999999999999971578 ) ) ;
#5120=CARTESIAN_POINT ( 'NONE',  ( -0.8626474017859412369, -36.14481870267513131, 2.932969818539080453 ) ) ;
#5123=ORIENTED_EDGE ( 'NONE', *, *, #9302, .F. ) ;
#5124=VERTEX_POINT ( 'NONE', #19970 ) ;
#5131=ORIENTED_EDGE ( 'NONE', *, *, #13212, .F. ) ;
#5135=DIRECTION ( 'NONE',  ( 1.000000000000000000, 1.208970125616053321E-17, 0.000000000000000000 ) ) ;
#5136=ADVANCED_FACE ( 'NONE', ( #829 ), #12962, .F. ) ;
#5137=CARTESIAN_POINT ( 'NONE',  ( -34.90673715956756240, 2.733356359154242119E-14, 5.750000000000001776 ) ) ;
#5138=DIRECTION ( 'NONE',  ( -6.505213034913038160E-19, -3.903127820947822896E-18, -1.000000000000000000 ) ) ;
#5139=EDGE_CURVE ( 'NONE', #18701, #11842, #13593, .T. ) ;
#5141=VERTEX_POINT ( 'NONE', #4060 ) ;
#5142=CARTESIAN_POINT ( 'NONE',  ( -11.93830856187180700, -33.47097213929440329, 3.000000000000063061 ) ) ;
#5151=ORIENTED_EDGE ( 'NONE', *, *, #303, .F. ) ;
#5152=DIRECTION ( 'NONE',  ( -6.505213034913038160E-19, -3.903127820947822896E-18, -1.000000000000000000 ) ) ;
#5167=EDGE_CURVE ( 'NONE', #8307, #5279, #5045, .T. ) ;
#5170=ADVANCED_FACE ( 'NONE', ( #5882 ), #14336, .F. ) ;
#5174=CARTESIAN_POINT ( 'NONE',  ( 15.12081897056688540, -33.51030287062373247, 2.800654218530485018 ) ) ;
#5180=DIRECTION ( 'NONE',  ( -6.505213034913038160E-19, -3.903127820947822896E-18, -1.000000000000000000 ) ) ;
#5181=CARTESIAN_POINT ( 'NONE',  ( -7.524443153164861897, 20.67323765728989926, -5.000000000000004441 ) ) ;
#5182=ORIENTED_EDGE ( 'NONE', *, *, #303, .T. ) ;
#5187=CARTESIAN_POINT ( 'NONE',  ( 2.220446049250313081E-13, 2.775557561562891351E-14, -2.800654218530485018 ) ) ;
#5192=CYLINDRICAL_SURFACE ( 'NONE', #648, 19.11328065563150957 ) ;
#5193=VECTOR ( 'NONE', #2440, 1000.000000000000000 ) ;
#5194=CIRCLE ( 'NONE', #2253, 19.11328065563150957 ) ;
#5195=DIRECTION ( 'NONE',  ( 1.000000000000000000, 0.000000000000000000, 0.000000000000000000 ) ) ;
#5202=ADVANCED_FACE ( 'NONE', ( #7594 ), #18013, .F. ) ;
#5205=CIRCLE ( 'NONE', #1912, 36.76383501243555685 ) ;
#5211=ORIENTED_EDGE ( 'NONE', *, *, #794, .F. ) ;
#5220=DIRECTION ( 'NONE',  ( -6.505213034913038160E-19, -3.903127820947822896E-18, -1.000000000000000000 ) ) ;
#5221=CARTESIAN_POINT ( 'NONE',  ( -13.06969024216325970, -19.15111107797470780, -4.999999999999969802 ) ) ;
#5222=DIRECTION ( 'NONE',  ( -1.000000000000000000, -1.208970125616060717E-17, 0.000000000000000000 ) ) ;
#5227=EDGE_CURVE ( 'NONE', #260, #19833, #19683, .T. ) ;
#5231=CARTESIAN_POINT ( 'NONE',  ( -30.60042966911705165, -7.474202570536076173, 3.000000000000023537 ) ) ;
#5234=AXIS2_PLACEMENT_3D ( 'NONE', #18219, #9734, #14760 ) ;
#5236=CARTESIAN_POINT ( 'NONE',  ( 12.00937115242647835, 34.74700806321096280, 2.800654218530512551 ) ) ;
#5241=AXIS2_PLACEMENT_3D ( 'NONE', #22282, #4856, #11826 ) ;
#5243=CARTESIAN_POINT ( 'NONE',  ( -27.64365646977265456, -17.09029715894952517, -2.999999999999981792 ) ) ;
#5249=ORIENTED_EDGE ( 'NONE', *, *, #18573, .F. ) ;
#5252=EDGE_CURVE ( 'NONE', #2560, #20709, #14450, .T. ) ;
#5253=ADVANCED_FACE ( 'NONE', ( #16869 ), #11369, .T. ) ;
#5254=AXIS2_PLACEMENT_3D ( 'NONE', #12489, #19616, #17896 ) ;
#5255=VERTEX_POINT ( 'NONE', #11708 ) ;
#5260=CARTESIAN_POINT ( 'NONE',  ( -7.711478842616581453, 31.57187188083529605, -7.000000000000006217 ) ) ;
#5261=CARTESIAN_POINT ( 'NONE',  ( -29.14949368109861894, 11.93972437435542133, 2.999999999999995559 ) ) ;
#5266=VERTEX_POINT ( 'NONE', #6105 ) ;
#5267=LINE ( 'NONE', #9033, #14509 ) ;
#5270=EDGE_CURVE ( 'NONE', #21037, #21090, #2146, .T. ) ;
#5273=AXIS2_PLACEMENT_3D ( 'NONE', #11909, #19141, #4825 ) ;
#5278=AXIS2_PLACEMENT_3D ( 'NONE', #14122, #6946, #5222 ) ;
#5279=VERTEX_POINT ( 'NONE', #3116 ) ;
#5283=ORIENTED_EDGE ( 'NONE', *, *, #10191, .T. ) ;
#5284=CARTESIAN_POINT ( 'NONE',  ( 21.41958700883258970, 27.56232195404059837, 3.000000000000002665 ) ) ;
#5286=CARTESIAN_POINT ( 'NONE',  ( -31.21605069118058040, -8.646032897229122938, -6.999999999999999112 ) ) ;
#5288=DIRECTION ( 'NONE',  ( 6.505213034913038160E-19, 3.903127820947822896E-18, 1.000000000000000000 ) ) ;
#5291=DIRECTION ( 'NONE',  ( -1.000000000000000000, -3.103995799953189701E-14, 0.000000000000000000 ) ) ;
#5293=CARTESIAN_POINT ( 'NONE',  ( 2.220446049250313081E-13, 2.775557561562891351E-14, -2.800654218530485018 ) ) ;
#5296=CARTESIAN_POINT ( 'NONE',  ( 22.97438720605771323, -22.98755168577421060, -7.000000000000006217 ) ) ;
#5300=VECTOR ( 'NONE', #5962, 1000.000000000000000 ) ;
#5303=VERTEX_POINT ( 'NONE', #20537 ) ;
#5308=ORIENTED_EDGE ( 'NONE', *, *, #14749, .T. ) ;
#5310=ADVANCED_FACE ( 'NONE', ( #18469 ), #21927, .T. ) ;
#5311=ORIENTED_EDGE ( 'NONE', *, *, #12688, .F. ) ;
#5316=CYLINDRICAL_SURFACE ( 'NONE', #5847, 0.9999999999999974465 ) ;
#5321=CARTESIAN_POINT ( 'NONE',  ( 35.43359966464143440, -7.197698565811765370, 2.932460736555821512 ) ) ;
#5322=ORIENTED_EDGE ( 'NONE', *, *, #10596, .T. ) ;
#5324=EDGE_CURVE ( 'NONE', #16900, #943, #9053, .T. ) ;
#5325=ORIENTED_EDGE ( 'NONE', *, *, #17045, .F. ) ;
#5326=LINE ( 'NONE', #17805, #3514 ) ;
#5327=AXIS2_PLACEMENT_3D ( 'NONE', #19082, #13903, #6393 ) ;
#5333=AXIS2_PLACEMENT_3D ( 'NONE', #8447, #6501, #3304 ) ;
#5335=ORIENTED_EDGE ( 'NONE', *, *, #12367, .T. ) ;
#5336=ADVANCED_FACE ( 'NONE', ( #20314 ), #18814, .T. ) ;
#5339=AXIS2_PLACEMENT_3D ( 'NONE', #13110, #863, #13214 ) ;
#5340=VERTEX_POINT ( 'NONE', #20429 ) ;
#5342=CARTESIAN_POINT ( 'NONE',  ( -11.98990878915331848, -34.11307262910443683, -2.932164912090521547 ) ) ;
#5343=VECTOR ( 'NONE', #18510, 1000.000000000000000 ) ;
#5345=DIRECTION ( 'NONE',  ( 1.000000000000000000, 0.000000000000000000, 0.000000000000000000 ) ) ;
#5350=DIRECTION ( 'NONE',  ( 6.505213034913038160E-19, 3.903127820947822896E-18, 1.000000000000000000 ) ) ;
#5355=AXIS2_PLACEMENT_3D ( 'NONE', #19864, #16297, #18136 ) ;
#5356=VECTOR ( 'NONE', #5378, 1000.000000000000000 ) ;
#5363=ORIENTED_EDGE ( 'NONE', *, *, #22321, .F. ) ;
#5364=ORIENTED_EDGE ( 'NONE', *, *, #21013, .F. ) ;
#5365=DIRECTION ( 'NONE',  ( 6.505213034913038160E-19, 3.903127820947822896E-18, 1.000000000000000000 ) ) ;
#5366=DIRECTION ( 'NONE',  ( -1.000000000000000000, -1.208970125616044077E-17, 0.000000000000000000 ) ) ;
#5370=FACE_OUTER_BOUND ( 'NONE', #10000, .T. ) ;
#5373=FACE_OUTER_BOUND ( 'NONE', #5880, .T. ) ;
#5375=VERTEX_POINT ( 'NONE', #4393 ) ;
#5376=CARTESIAN_POINT ( 'NONE',  ( 7.094908322883425100, -35.33352588067112521, -6.999999999999950262 ) ) ;
#5378=DIRECTION ( 'NONE',  ( 6.505213034913038160E-19, 3.903127820947822896E-18, 1.000000000000000000 ) ) ;
#5380=EDGE_CURVE ( 'NONE', #11353, #21378, #3569, .T. ) ;
#5382=ORIENTED_EDGE ( 'NONE', *, *, #1066, .F. ) ;
#5384=CIRCLE ( 'NONE', #18183, 36.76383501243555685 ) ;
#5387=ORIENTED_EDGE ( 'NONE', *, *, #22535, .F. ) ;
#5397=CARTESIAN_POINT ( 'NONE',  ( -26.65040777864139443, -24.43568323314263324, 2.932460736555830838 ) ) ;
#5404=LINE ( 'NONE', #17429, #15206 ) ;
#5408=VERTEX_POINT ( 'NONE', #6901 ) ;
#5411=CYLINDRICAL_SURFACE ( 'NONE', #20693, 19.11328065563150957 ) ;
#5415=EDGE_CURVE ( 'NONE', #13797, #12800, #22235, .T. ) ;
#5417=VERTEX_POINT ( 'NONE', #22487 ) ;
#5421=LINE ( 'NONE', #1871, #6279 ) ;
#5428=CARTESIAN_POINT ( 'NONE',  ( -21.97438720605751783, 22.98755168577401520, 3.000000000000023537 ) ) ;
#5432=CARTESIAN_POINT ( 'NONE',  ( -28.95348479018558407, 14.76298474240494940, 3.000000000000023537 ) ) ;
#5435=ORIENTED_EDGE ( 'NONE', *, *, #15059, .F. ) ;
#5443=CARTESIAN_POINT ( 'NONE',  ( 1.110223024625156540E-13, -5.551115123125782702E-14, -6.999999999999950262 ) ) ;
#5444=EDGE_CURVE ( 'NONE', #12921, #295, #22606, .T. ) ;
#5445=EDGE_CURVE ( 'NONE', #10809, #15365, #5751, .T. ) ;
#5446=CARTESIAN_POINT ( 'NONE',  ( -35.79662727779868447, 4.171001175319489107, -7.000000000000006217 ) ) ;
#5447=AXIS2_PLACEMENT_3D ( 'NONE', #15801, #7106, #14074 ) ;
#5453=VERTEX_POINT ( 'NONE', #15466 ) ;
#5454=CARTESIAN_POINT ( 'NONE',  ( 4.153395668489503478, -35.29097153256777375, -2.999999999999992006 ) ) ;
#5455=FACE_OUTER_BOUND ( 'NONE', #20970, .T. ) ;
#5459=AXIS2_PLACEMENT_3D ( 'NONE', #15651, #5138, #17369 ) ;
#5463=CIRCLE ( 'NONE', #18269, 34.90673715956759082 ) ;
#5467=EDGE_CURVE ( 'NONE', #11128, #17574, #11238, .T. ) ;
#5468=DIRECTION ( 'NONE',  ( -1.000000000000000000, -1.208970125616060101E-17, 6.505213034913038160E-19 ) ) ;
#5470=CARTESIAN_POINT ( 'NONE',  ( -30.48934413892778750, 16.99647590252656570, 2.999999999999999112 ) ) ;
#5477=FACE_OUTER_BOUND ( 'NONE', #11545, .T. ) ;
#5480=DIRECTION ( 'NONE',  ( 1.000000000000000000, 0.000000000000000000, 0.000000000000000000 ) ) ;
#5481=CARTESIAN_POINT ( 'NONE',  ( -24.24871130596430291, 13.99999999999962341, -4.999999999999984013 ) ) ;
#5497=EDGE_CURVE ( 'NONE', #4768, #6508, #13084, .T. ) ;
#5500=DIRECTION ( 'NONE',  ( 6.505213034913038160E-19, 3.903127820947822896E-18, 1.000000000000000000 ) ) ;
#5505=DIRECTION ( 'NONE',  ( 1.000000000000000000, 0.000000000000000000, 0.000000000000000000 ) ) ;
#5508=CIRCLE ( 'NONE', #2600, 20.00000000000002132 ) ;
#5510=ORIENTED_EDGE ( 'NONE', *, *, #8922, .F. ) ;
#5515=LINE ( 'NONE', #7350, #10525 ) ;
#5520=ORIENTED_EDGE ( 'NONE', *, *, #3105, .T. ) ;
#5521=ORIENTED_EDGE ( 'NONE', *, *, #11835, .F. ) ;
#5522=EDGE_CURVE ( 'NONE', #14674, #11380, #7909, .T. ) ;
#5524=CARTESIAN_POINT ( 'NONE',  ( 27.01645732367882857, 17.86915608785644238, -6.999999999999985789 ) ) ;
#5528=CARTESIAN_POINT ( 'NONE',  ( -21.05198877411783442, 30.13956425491229396, -2.800654218530457484 ) ) ;
#5530=ORIENTED_EDGE ( 'NONE', *, *, #520, .T. ) ;
#5531=LINE ( 'NONE', #19519, #21496 ) ;
#5533=AXIS2_PLACEMENT_3D ( 'NONE', #20308, #16862, #20192 ) ;
#5535=CARTESIAN_POINT ( 'NONE',  ( -10.00000000000000888, 2.999999999999836131, -4.999999999999948486 ) ) ;
#5540=CARTESIAN_POINT ( 'NONE',  ( 16.99647590252670426, 30.48934413892764894, -2.999999999999971578 ) ) ;
#5544=DIRECTION ( 'NONE',  ( -1.000000000000000000, -1.208970125616057944E-17, 0.000000000000000000 ) ) ;
#5545=ADVANCED_FACE ( 'NONE', ( #4247 ), #18099, .F. ) ;
#5546=CARTESIAN_POINT ( 'NONE',  ( -26.10969099697608797, -24.10368028608829505, -2.999999999999992006 ) ) ;
#5548=ORIENTED_EDGE ( 'NONE', *, *, #12286, .F. ) ;
#5550=EDGE_LOOP ( 'NONE', ( #19642, #18004, #2181, #19702 ) ) ;
#5553=DIRECTION ( 'NONE',  ( -1.000000000000000000, 0.000000000000000000, 0.000000000000000000 ) ) ;
#5558=EDGE_CURVE ( 'NONE', #11380, #4189, #19728, .T. ) ;
#5560=VERTEX_POINT ( 'NONE', #5734 ) ;
#5563=LINE ( 'NONE', #2246, #16398 ) ;
#5565=B_SPLINE_CURVE_WITH_KNOTS ( 'NONE', 3,
 ( #14730, #12561, #9142, #20030 ),
 .UNSPECIFIED., .F., .F.,
 ( 4, 4 ),
 ( 0.001893031756885345078, 0.003808480026563831368 ),
 .UNSPECIFIED. ) ;
#5569=DIRECTION ( 'NONE',  ( -1.000000000000000000, -1.208970125616060717E-17, 0.000000000000000000 ) ) ;
#5570=DIRECTION ( 'NONE',  ( -6.505213034913038160E-19, -3.903127820947822896E-18, -1.000000000000000000 ) ) ;
#5580=ADVANCED_FACE ( 'NONE', ( #6410 ), #10513, .T. ) ;
#5593=DIRECTION ( 'NONE',  ( 6.505213034913038160E-19, 3.903127820947822896E-18, 1.000000000000000000 ) ) ;
#5607=CYLINDRICAL_SURFACE ( 'NONE', #16426, 0.9999999999999974465 ) ;
#5615=AXIS2_PLACEMENT_3D ( 'NONE', #15789, #8820, #8477 ) ;
#5617=CYLINDRICAL_SURFACE ( 'NONE', #8129, 27.99999999999999645 ) ;
#5619=DIRECTION ( 'NONE',  ( 1.000000000000000000, 0.000000000000000000, 0.000000000000000000 ) ) ;
#5625=DIRECTION ( 'NONE',  ( 1.000000000000000000, 0.000000000000000000, 0.000000000000000000 ) ) ;
#5626=CARTESIAN_POINT ( 'NONE',  ( -16.56444186175087907, 26.79308242454872513, -2.999999999999992450 ) ) ;
#5635=DIRECTION ( 'NONE',  ( 1.000000000000000000, 1.208970125616063182E-17, 0.000000000000000000 ) ) ;
#5638=FACE_OUTER_BOUND ( 'NONE', #14565, .T. ) ;
#5640=AXIS2_PLACEMENT_3D ( 'NONE', #5187, #13631, #20648 ) ;
#5641=ORIENTED_EDGE ( 'NONE', *, *, #2995, .F. ) ;
#5642=CARTESIAN_POINT ( 'NONE',  ( 3.330669073875469621E-13, -1.110223024625156540E-13, -2.999999999999971578 ) ) ;
#5645=CARTESIAN_POINT ( 'NONE',  ( 20.54749497201924058, -29.74882400976400376, 2.932969818539067131 ) ) ;
#5647=CARTESIAN_POINT ( 'NONE',  ( 35.92356703407504170, 4.104166344908929176, 2.932460736555814407 ) ) ;
#5652=FACE_OUTER_BOUND ( 'NONE', #19669, .T. ) ;
#5654=VECTOR ( 'NONE', #13416, 1000.000000000000000 ) ;
#5659=DIRECTION ( 'NONE',  ( -6.505213034913038160E-19, -3.903127820947822896E-18, -1.000000000000000000 ) ) ;
#5660=EDGE_CURVE ( 'NONE', #2593, #22272, #7987, .T. ) ;
#5661=EDGE_CURVE ( 'NONE', #5124, #19660, #4328, .T. ) ;
#5663=AXIS2_PLACEMENT_3D ( 'NONE', #11881, #6286, #22441 ) ;
#5664=VERTEX_POINT ( 'NONE', #9617 ) ;
#5667=EDGE_CURVE ( 'NONE', #16668, #13519, #11627, .T. ) ;
#5668=ORIENTED_EDGE ( 'NONE', *, *, #11189, .T. ) ;
#5674=ORIENTED_EDGE ( 'NONE', *, *, #14947, .F. ) ;
#5675=CARTESIAN_POINT ( 'NONE',  ( 17.66631876130925249, -31.41173278719244877, 2.999999999999995559 ) ) ;
#5676=AXIS2_PLACEMENT_3D ( 'NONE', #21640, #21757, #21410 ) ;
#5677=VECTOR ( 'NONE', #1365, 1000.000000000000000 ) ;
#5678=ADVANCED_FACE ( 'NONE', ( #11220 ), #4474, .F. ) ;
#5690=AXIS2_PLACEMENT_3D ( 'NONE', #1152, #20410, #11908 ) ;
#5697=ORIENTED_EDGE ( 'NONE', *, *, #612, .T. ) ;
#5698=CIRCLE ( 'NONE', #19963, 34.90673715956759082 ) ;
#5705=AXIS2_PLACEMENT_3D ( 'NONE', #4318, #18507, #11170 ) ;
#5706=CARTESIAN_POINT ( 'NONE',  ( -14.67611967928926475, 31.67162468655990182, -2.999999999999971578 ) ) ;
#5709=FACE_OUTER_BOUND ( 'NONE', #12121, .T. ) ;
#5711=CARTESIAN_POINT ( 'NONE',  ( -34.84717828836173936, 6.955395936296730142, -3.000000000000011990 ) ) ;
#5714=AXIS2_PLACEMENT_3D ( 'NONE', #9156, #14178, #5718 ) ;
#5716=CARTESIAN_POINT ( 'NONE',  ( -9.999999999999758415, -3.000000000000169198, -4.999999999999984013 ) ) ;
#5717=FACE_OUTER_BOUND ( 'NONE', #6893, .T. ) ;
#5718=DIRECTION ( 'NONE',  ( 1.000000000000000000, 0.000000000000000000, 0.000000000000000000 ) ) ;
#5719=EDGE_CURVE ( 'NONE', #21713, #5723, #13440, .T. ) ;
#5721=AXIS2_PLACEMENT_3D ( 'NONE', #1958, #12381, #15917 ) ;
#5723=VERTEX_POINT ( 'NONE', #5261 ) ;
#5725=CARTESIAN_POINT ( 'NONE',  ( -18.65063509461096913, 12.49999999999990052, -5.000000000000004441 ) ) ;
#5726=EDGE_CURVE ( 'NONE', #877, #5417, #19643, .T. ) ;
#5727=ORIENTED_EDGE ( 'NONE', *, *, #14097, .F. ) ;
#5729=VECTOR ( 'NONE', #19562, 1000.000000000000000 ) ;
#5731=DIRECTION ( 'NONE',  ( -6.505213034913038160E-19, -3.903127820947822896E-18, -1.000000000000000000 ) ) ;
#5732=VERTEX_POINT ( 'NONE', #22456 ) ;
#5733=CARTESIAN_POINT ( 'NONE',  ( 11.98978967046198996, 34.10919265018070945, 2.932969818539058249 ) ) ;
#5734=CARTESIAN_POINT ( 'NONE',  ( -30.57187188083528540, -7.711478842616581453, 3.000000000000023537 ) ) ;
#5736=CARTESIAN_POINT ( 'NONE',  ( 6.070730550691044947, 31.88709182564705813, 2.999999999999995559 ) ) ;
#5737=CARTESIAN_POINT ( 'NONE',  ( 3.330669073875469621E-13, -1.110223024625156540E-13, -2.999999999999971578 ) ) ;
#5738=CARTESIAN_POINT ( 'NONE',  ( -27.84804035626035912, 24.75236754129145211, -2.999999999999995559 ) ) ;
#5739=CARTESIAN_POINT ( 'NONE',  ( -18.83615802559775076, 32.14641817400173807, -6.999999999999950262 ) ) ;
#5745=EDGE_LOOP ( 'NONE', ( #3226, #16056, #12963, #12339 ) ) ;
#5747=EDGE_CURVE ( 'NONE', #22237, #18105, #6636, .T. ) ;
#5751=CIRCLE ( 'NONE', #8682, 19.11328065563151668 ) ;
#5752=ORIENTED_EDGE ( 'NONE', *, *, #8040, .F. ) ;
#5754=ORIENTED_EDGE ( 'NONE', *, *, #8717, .T. ) ;
#5759=DIRECTION ( 'NONE',  ( -1.000000000000000000, 0.000000000000000000, 0.000000000000000000 ) ) ;
#5760=CARTESIAN_POINT ( 'NONE',  ( 15.12081897056669000, -33.51030287062373247, -2.000000000000005329 ) ) ;
#5761=DIRECTION ( 'NONE',  ( -1.000000000000000000, 0.000000000000000000, 0.000000000000000000 ) ) ;
#5765=ORIENTED_EDGE ( 'NONE', *, *, #7700, .T. ) ;
#5769=CARTESIAN_POINT ( 'NONE',  ( -4.080045426412465481, 32.20238537491798780, 2.999999999999995559 ) ) ;
#5770=ORIENTED_EDGE ( 'NONE', *, *, #11418, .F. ) ;
#5775=CARTESIAN_POINT ( 'NONE',  ( -33.51030287062352642, -15.12081897056683033, 2.800654218530502337 ) ) ;
#5778=AXIS2_PLACEMENT_3D ( 'NONE', #13039, #804, #4368 ) ;
#5785=EDGE_CURVE ( 'NONE', #5453, #20150, #18965, .T. ) ;
#5786=AXIS2_PLACEMENT_3D ( 'NONE', #9334, #13503, #1380 ) ;
#5788=ORIENTED_EDGE ( 'NONE', *, *, #6256, .F. ) ;
#5792=AXIS2_PLACEMENT_3D ( 'NONE', #1141, #8240, #6073 ) ;
#5799=TOROIDAL_SURFACE ( 'NONE', #20804, 34.90673715956759082, 8.750000000000000000 ) ;
#5800=ORIENTED_EDGE ( 'NONE', *, *, #14410, .F. ) ;
#5803=DIRECTION ( 'NONE',  ( -6.505213034913038160E-19, -3.903127820947822896E-18, -1.000000000000000000 ) ) ;
#5805=DIRECTION ( 'NONE',  ( 6.505213034913038160E-19, 3.903127820947822896E-18, 1.000000000000000000 ) ) ;
#5807=AXIS2_PLACEMENT_3D ( 'NONE', #4565, #21747, #13132 ) ;
#5811=VERTEX_POINT ( 'NONE', #15779 ) ;
#5812=EDGE_LOOP ( 'NONE', ( #6401, #8899, #9786, #4982 ) ) ;
#5814=ORIENTED_EDGE ( 'NONE', *, *, #8846, .F. ) ;
#5815=CARTESIAN_POINT ( 'NONE',  ( 32.75570538720803881, -15.02862401740803833, 2.999999999999995559 ) ) ;
#5822=DIRECTION ( 'NONE',  ( -1.000000000000000000, -1.208970125616046080E-17, 6.505213034913038160E-19 ) ) ;
#5823=CYLINDRICAL_SURFACE ( 'NONE', #18624, 31.50000000000001421 ) ;
#5825=FACE_OUTER_BOUND ( 'NONE', #16665, .T. ) ;
#5828=DIRECTION ( 'NONE',  ( 1.000000000000000000, 0.000000000000000000, 0.000000000000000000 ) ) ;
#5833=CARTESIAN_POINT ( 'NONE',  ( 21.65063509461093005, 12.50000000000006750, -5.000000000000004441 ) ) ;
#5837=DIRECTION ( 'NONE',  ( -1.000000000000000000, -1.208970125616063490E-17, 0.000000000000000000 ) ) ;
#5842=CARTESIAN_POINT ( 'NONE',  ( 32.83234229683740324, -11.85401191286897316, 2.999999999999995559 ) ) ;
#5847=AXIS2_PLACEMENT_3D ( 'NONE', #12613, #12294, #19299 ) ;
#5856=DIRECTION ( 'NONE',  ( 6.505213034913038160E-19, 3.903127820947822896E-18, 1.000000000000000000 ) ) ;
#5863=ORIENTED_EDGE ( 'NONE', *, *, #10962, .T. ) ;
#5865=CIRCLE ( 'NONE', #19772, 19.11328065563152379 ) ;
#5871=VERTEX_POINT ( 'NONE', #3665 ) ;
#5874=VERTEX_POINT ( 'NONE', #16008 ) ;
#5875=DIRECTION ( 'NONE',  ( 6.505213034913038160E-19, 3.903127820947822896E-18, 1.000000000000000000 ) ) ;
#5876=CARTESIAN_POINT ( 'NONE',  ( -5.074925817841774212, 32.10132595304123981, -2.999999999999999112 ) ) ;
#5880=EDGE_LOOP ( 'NONE', ( #11231, #9186, #7970, #2543 ) ) ;
#5882=FACE_OUTER_BOUND ( 'NONE', #2007, .T. ) ;
#5883=ORIENTED_EDGE ( 'NONE', *, *, #14368, .T. ) ;
#5884=FACE_OUTER_BOUND ( 'NONE', #19623, .T. ) ;
#5886=ORIENTED_EDGE ( 'NONE', *, *, #13929, .T. ) ;
#5894=LINE ( 'NONE', #3958, #4864 ) ;
#5895=CIRCLE ( 'NONE', #11742, 31.50000000000000711 ) ;
#5897=DIRECTION ( 'NONE',  ( 6.505213034913038160E-19, 3.903127820947822896E-18, 1.000000000000000000 ) ) ;
#5908=ORIENTED_EDGE ( 'NONE', *, *, #5661, .T. ) ;
#5909=CARTESIAN_POINT ( 'NONE',  ( 18.00000000000019185, -2.519513924556040635E-14, 4.999999999999993783 ) ) ;
#5916=DIRECTION ( 'NONE',  ( -6.505213034913038160E-19, -3.903127820947822896E-18, -1.000000000000000000 ) ) ;
#5917=VECTOR ( 'NONE', #19853, 1000.000000000000000 ) ;
#5920=ADVANCED_FACE ( 'NONE', ( #662 ), #5823, .T. ) ;
#5922=ORIENTED_EDGE ( 'NONE', *, *, #18266, .F. ) ;
#5931=CARTESIAN_POINT ( 'NONE',  ( -7.474202570535936729, 30.60042966911716178, -2.999999999999971578 ) ) ;
#5933=EDGE_CURVE ( 'NONE', #3830, #18499, #2509, .T. ) ;
#5935=DIRECTION ( 'NONE',  ( -6.505213034913038160E-19, -3.903127820947822896E-18, -1.000000000000000000 ) ) ;
#5938=CARTESIAN_POINT ( 'NONE',  ( 29.36548507648051398, 13.83143812983095344, -2.999999999999971578 ) ) ;
#5939=ORIENTED_EDGE ( 'NONE', *, *, #14145, .T. ) ;
#5940=VERTEX_POINT ( 'NONE', #15888 ) ;
#5948=CARTESIAN_POINT ( 'NONE',  ( -36.54278193890294091, -4.025500340002652777, 2.800654218530481465 ) ) ;
#5950=DIRECTION ( 'NONE',  ( -6.505213034913038160E-19, -3.903127820947822896E-18, -1.000000000000000000 ) ) ;
#5953=FACE_OUTER_BOUND ( 'NONE', #1080, .T. ) ;
#5956=DIRECTION ( 'NONE',  ( 1.000000000000000000, 1.208970125616053475E-17, 0.000000000000000000 ) ) ;
#5962=DIRECTION ( 'NONE',  ( 6.505213034913038160E-19, 3.903127820947822896E-18, 1.000000000000000000 ) ) ;
#5969=CYLINDRICAL_SURFACE ( 'NONE', #19242, 31.50000000000000000 ) ;
#5976=CIRCLE ( 'NONE', #16595, 18.00000000000000000 ) ;
#5979=CIRCLE ( 'NONE', #16577, 34.90673715956759082 ) ;
#5982=CARTESIAN_POINT ( 'NONE',  ( 17.09029715894955359, -27.64365646977279312, -7.000000000000006217 ) ) ;
#5985=CARTESIAN_POINT ( 'NONE',  ( -22.97438720605733664, 22.98755168577407204, -2.999999999999971578 ) ) ;
#5990=CARTESIAN_POINT ( 'NONE',  ( 1.011722470948207109, 35.51751788033340773, -3.000000000000015543 ) ) ;
#5991=CIRCLE ( 'NONE', #14753, 19.11328065563151668 ) ;
#5995=AXIS2_PLACEMENT_3D ( 'NONE', #20480, #17138, #16915 ) ;
#5997=ORIENTED_EDGE ( 'NONE', *, *, #15433, .F. ) ;
#6002=CARTESIAN_POINT ( 'NONE',  ( 31.11077005834439291, -4.936596639065371050, -6.999999999999950262 ) ) ;
#6006=AXIS2_PLACEMENT_3D ( 'NONE', #21992, #17123, #16708 ) ;
#6007=AXIS2_PLACEMENT_3D ( 'NONE', #1261, #22015, #20411 ) ;
#6015=DIRECTION ( 'NONE',  ( -6.505213034913038160E-19, -3.903127820947822896E-18, -1.000000000000000000 ) ) ;
#6021=DIRECTION ( 'NONE',  ( 1.000000000000000000, 0.000000000000000000, 0.000000000000000000 ) ) ;
#6023=CIRCLE ( 'NONE', #16612, 2.999999999999999112 ) ;
#6025=CARTESIAN_POINT ( 'NONE',  ( -18.22261011550273224, -31.92986134326242365, -2.800654218530485018 ) ) ;
#6031=AXIS2_PLACEMENT_3D ( 'NONE', #18768, #8016, #6287 ) ;
#6032=EDGE_CURVE ( 'NONE', #3715, #14229, #7623, .T. ) ;
#6034=CARTESIAN_POINT ( 'NONE',  ( -32.35999952201586183, 1.423424233832598640, 2.999999999999995559 ) ) ;
#6036=EDGE_LOOP ( 'NONE', ( #20811, #10587, #15420, #2760 ) ) ;
#6040=CIRCLE ( 'NONE', #7500, 2.999999999999999112 ) ;
#6049=ORIENTED_EDGE ( 'NONE', *, *, #2294, .F. ) ;
#6052=CARTESIAN_POINT ( 'NONE',  ( 14.76298474240531000, 28.95348479018561250, -7.000000000000006217 ) ) ;
#6053=AXIS2_PLACEMENT_3D ( 'NONE', #2920, #17098, #1414 ) ;
#6055=EDGE_CURVE ( 'NONE', #18413, #16878, #19458, .T. ) ;
#6056=ORIENTED_EDGE ( 'NONE', *, *, #11607, .T. ) ;
#6058=CARTESIAN_POINT ( 'NONE',  ( 35.16985127952396084, 10.70799354677376414, 2.800654218530485018 ) ) ;
#6059=CIRCLE ( 'NONE', #6854, 19.11328065563150957 ) ;
#6060=VECTOR ( 'NONE', #21273, 1000.000000000000000 ) ;
#6063=ADVANCED_FACE ( 'NONE', ( #2730 ), #18531, .T. ) ;
#6064=DIRECTION ( 'NONE',  ( 6.505213034913038160E-19, 3.903127820947822896E-18, 1.000000000000000000 ) ) ;
#6065=AXIS2_PLACEMENT_3D ( 'NONE', #12034, #19029, #16854 ) ;
#6066=CIRCLE ( 'NONE', #3153, 34.90673715956759082 ) ;
#6069=CIRCLE ( 'NONE', #2043, 19.11328065563150957 ) ;
#6073=DIRECTION ( 'NONE',  ( -1.000000000000000000, -1.208970125616046080E-17, 6.505213034913038160E-19 ) ) ;
#6074=EDGE_CURVE ( 'NONE', #22110, #12599, #4343, .T. ) ;
#6081=CYLINDRICAL_SURFACE ( 'NONE', #22209, 36.76383501243555685 ) ;
#6091=CIRCLE ( 'NONE', #8655, 19.11328065563152379 ) ;
#6092=VERTEX_POINT ( 'NONE', #3276 ) ;
#6104=CARTESIAN_POINT ( 'NONE',  ( -15.00428685838175724, 32.89708536800382888, 2.932460736555835279 ) ) ;
#6105=CARTESIAN_POINT ( 'NONE',  ( 22.28024240313503057, 22.26748298433264850, 3.000000000000023537 ) ) ;
#6108=CIRCLE ( 'NONE', #9770, 34.90673715956759082 ) ;
#6109=EDGE_CURVE ( 'NONE', #8183, #2221, #14228, .T. ) ;
#6112=ORIENTED_EDGE ( 'NONE', *, *, #13920, .F. ) ;
#6126=AXIS2_PLACEMENT_3D ( 'NONE', #456, #4135, #4037 ) ;
#6131=VERTEX_POINT ( 'NONE', #10795 ) ;
#6133=TOROIDAL_SURFACE ( 'NONE', #11980, 34.90673715956759082, 8.750000000000000000 ) ;
#6136=CARTESIAN_POINT ( 'NONE',  ( -9.999999999999980460, -3.000000000000002665, 4.999999999999997335 ) ) ;
#6140=AXIS2_PLACEMENT_3D ( 'NONE', #6220, #9767, #13405 ) ;
#6142=FACE_OUTER_BOUND ( 'NONE', #12733, .T. ) ;
#6143=CIRCLE ( 'NONE', #15281, 1.000000000000000888 ) ;
#6148=ADVANCED_FACE ( 'NONE', ( #17345 ), #21244, .F. ) ;
#6176=VECTOR ( 'NONE', #5288, 1000.000000000000000 ) ;
#6178=CARTESIAN_POINT ( 'NONE',  ( 22.98755168577445929, 22.97438720605740770, -6.999999999999950262 ) ) ;
#6187=VERTEX_POINT ( 'NONE', #8643 ) ;
#6193=B_SPLINE_CURVE_WITH_KNOTS ( 'NONE', 3,
 ( #20619, #20742, #5051, #19025 ),
 .UNSPECIFIED., .F., .F.,
 ( 4, 4 ),
 ( 0.001875451646902783712, 0.003761979286331212577 ),
 .UNSPECIFIED. ) ;
#6203=ADVANCED_FACE ( 'NONE', ( #15502 ), #22646, .T. ) ;
#6205=DIRECTION ( 'NONE',  ( -6.505213034913038160E-19, -3.903127820947822896E-18, -1.000000000000000000 ) ) ;
#6211=VERTEX_POINT ( 'NONE', #12305 ) ;
#6214=DIRECTION ( 'NONE',  ( 1.000000000000000000, 0.000000000000000000, 0.000000000000000000 ) ) ;
#6215=DIRECTION ( 'NONE',  ( 1.000000000000000000, 0.000000000000000000, 0.000000000000000000 ) ) ;
#6217=DIRECTION ( 'NONE',  ( 6.505213034913038160E-19, 3.903127820947822896E-18, 1.000000000000000000 ) ) ;
#6220=CARTESIAN_POINT ( 'NONE',  ( -37.07861450834799655, 3.656418565263969356, -7.000000000000006217 ) ) ;
#6221=ORIENTED_EDGE ( 'NONE', *, *, #8412, .T. ) ;
#6222=DIRECTION ( 'NONE',  ( -6.505213034913038160E-19, -3.903127820947822896E-18, -1.000000000000000000 ) ) ;
#6230=ORIENTED_EDGE ( 'NONE', *, *, #11869, .F. ) ;
#6233=VERTEX_POINT ( 'NONE', #3947 ) ;
#6235=EDGE_CURVE ( 'NONE', #3953, #14343, #7717, .T. ) ;
#6238=DIRECTION ( 'NONE',  ( 1.000000000000000000, 1.208970125616062874E-17, 0.000000000000000000 ) ) ;
#6242=AXIS2_PLACEMENT_3D ( 'NONE', #318, #195, #7191 ) ;
#6247=LINE ( 'NONE', #13206, #2611 ) ;
#6255=FACE_OUTER_BOUND ( 'NONE', #20097, .T. ) ;
#6256=EDGE_CURVE ( 'NONE', #5255, #14343, #10170, .T. ) ;
#6258=DIRECTION ( 'NONE',  ( -1.000000000000000000, -1.208970125616081209E-17, 0.000000000000000000 ) ) ;
#6263=CARTESIAN_POINT ( 'NONE',  ( -16.06969024216331476, -19.15111107797465451, 2.999999999999995559 ) ) ;
#6269=CARTESIAN_POINT ( 'NONE',  ( 29.33526866242108611, -22.15900668633799597, -1.999999999999980904 ) ) ;
#6270=VECTOR ( 'NONE', #10305, 1000.000000000000000 ) ;
#6275=DIRECTION ( 'NONE',  ( -1.000000000000000000, -4.175647542716197082E-14, 0.000000000000000000 ) ) ;
#6279=VECTOR ( 'NONE', #17667, 1000.000000000000000 ) ;
#6280=AXIS2_PLACEMENT_3D ( 'NONE', #7933, #15119, #18587 ) ;
#6284=DIRECTION ( 'NONE',  ( -6.505213034913038160E-19, -3.903127820947822896E-18, -1.000000000000000000 ) ) ;
#6286=DIRECTION ( 'NONE',  ( -6.505213034913038160E-19, -3.903127820947822896E-18, -1.000000000000000000 ) ) ;
#6287=DIRECTION ( 'NONE',  ( -1.000000000000000000, -1.208970125616044077E-17, 0.000000000000000000 ) ) ;
#6288=DIRECTION ( 'NONE',  ( 1.000000000000000000, 0.000000000000000000, 0.000000000000000000 ) ) ;
#6291=VECTOR ( 'NONE', #10886, 1000.000000000000000 ) ;
#6303=DIRECTION ( 'NONE',  ( -6.505213034913038160E-19, -3.903127820947822896E-18, -1.000000000000000000 ) ) ;
#6304=DIRECTION ( 'NONE',  ( 1.000000000000000000, 0.000000000000000000, 0.000000000000000000 ) ) ;
#6305=CARTESIAN_POINT ( 'NONE',  ( -29.33526866242079478, 22.15900668633771886, 2.800654218530485018 ) ) ;
#6306=EDGE_CURVE ( 'NONE', #15747, #7646, #16027, .T. ) ;
#6313=ORIENTED_EDGE ( 'NONE', *, *, #21498, .F. ) ;
#6319=AXIS2_PLACEMENT_3D ( 'NONE', #13885, #20902, #8299 ) ;
#6321=CARTESIAN_POINT ( 'NONE',  ( -10.34893680499411239, 34.64233806479123956, 2.932969818539072016 ) ) ;
#6324=CARTESIAN_POINT ( 'NONE',  ( -14.67611967928904271, 31.67162468655987340, 3.000000000000009770 ) ) ;
#6336=DIRECTION ( 'NONE',  ( 1.000000000000000000, 1.208970125616063490E-17, 0.000000000000000000 ) ) ;
#6339=EDGE_LOOP ( 'NONE', ( #20543, #3126, #6966, #9548, #10328, #5530 ) ) ;
#6343=VECTOR ( 'NONE', #8104, 1000.000000000000000 ) ;
#6346=ORIENTED_EDGE ( 'NONE', *, *, #8898, .F. ) ;
#6351=FACE_OUTER_BOUND ( 'NONE', #11182, .T. ) ;
#6357=DIRECTION ( 'NONE',  ( 6.505213034913038160E-19, 3.903127820947822896E-18, 1.000000000000000000 ) ) ;
#6361=CARTESIAN_POINT ( 'NONE',  ( -1.128083539116253586, -34.88850421923977763, -2.999999999999971578 ) ) ;
#6363=CARTESIAN_POINT ( 'NONE',  ( 2.220446049250313081E-13, -2.498001805406602216E-13, -6.859353255829918616 ) ) ;
#6364=ADVANCED_FACE ( 'NONE', ( #20207 ), #4628, .F. ) ;
#6367=FACE_OUTER_BOUND ( 'NONE', #3757, .T. ) ;
#6373=VECTOR ( 'NONE', #811, 1000.000000000000000 ) ;
#6377=EDGE_CURVE ( 'NONE', #19404, #6211, #687, .T. ) ;
#6384=CARTESIAN_POINT ( 'NONE',  ( 29.14949368109878591, -11.93972437435561496, 3.000000000000023537 ) ) ;
#6391=EDGE_LOOP ( 'NONE', ( #13678, #4858, #16982, #3070 ) ) ;
#6392=DIRECTION ( 'NONE',  ( -6.505213034913038160E-19, -3.903127820947822896E-18, -1.000000000000000000 ) ) ;
#6393=DIRECTION ( 'NONE',  ( 1.000000000000000000, 0.000000000000000000, 0.000000000000000000 ) ) ;
#6395=EDGE_CURVE ( 'NONE', #19660, #16550, #11212, .T. ) ;
#6397=DIRECTION ( 'NONE',  ( 1.000000000000000000, 0.000000000000000000, 0.000000000000000000 ) ) ;
#6400=EDGE_CURVE ( 'NONE', #6131, #2785, #12068, .T. ) ;
#6401=ORIENTED_EDGE ( 'NONE', *, *, #6908, .F. ) ;
#6403=VERTEX_POINT ( 'NONE', #445 ) ;
#6409=CARTESIAN_POINT ( 'NONE',  ( 28.96193690644957641, 14.74639653023213093, -6.999999999999950262 ) ) ;
#6410=FACE_OUTER_BOUND ( 'NONE', #8750, .T. ) ;
#6411=CIRCLE ( 'NONE', #8953, 34.90673715956759082 ) ;
#6414=AXIS2_PLACEMENT_3D ( 'NONE', #700, #20062, #2534 ) ;
#6416=VERTEX_POINT ( 'NONE', #5948 ) ;
#6418=DIRECTION ( 'NONE',  ( -6.505213034913038160E-19, -3.903127820947822896E-18, -1.000000000000000000 ) ) ;
#6420=DIRECTION ( 'NONE',  ( 1.000000000000000000, 0.000000000000000000, 0.000000000000000000 ) ) ;
#6421=EDGE_CURVE ( 'NONE', #691, #6233, #22465, .T. ) ;
#6424=CARTESIAN_POINT ( 'NONE',  ( -2.422192751863727622, -32.40961249803553557, -6.999999999999950262 ) ) ;
#6426=ADVANCED_FACE ( 'NONE', ( #12809 ), #14530, .T. ) ;
#6429=TOROIDAL_SURFACE ( 'NONE', #5339, 34.90673715956759082, 8.750000000000000000 ) ;
#6430=AXIS2_PLACEMENT_3D ( 'NONE', #22070, #14826, #20236 ) ;
#6434=ORIENTED_EDGE ( 'NONE', *, *, #13250, .T. ) ;
#6443=EDGE_LOOP ( 'NONE', ( #14324, #4513, #18662, #19273 ) ) ;
#6445=CYLINDRICAL_SURFACE ( 'NONE', #9750, 19.11328065563151668 ) ;
#6448=CARTESIAN_POINT ( 'NONE',  ( -36.75746821813285692, 0.6841746959066752343, -2.800654218530457484 ) ) ;
#6449=ORIENTED_EDGE ( 'NONE', *, *, #14981, .T. ) ;
#6465=ORIENTED_EDGE ( 'NONE', *, *, #8090, .F. ) ;
#6466=AXIS2_PLACEMENT_3D ( 'NONE', #2222, #16182, #492 ) ;
#6474=CARTESIAN_POINT ( 'NONE',  ( -10.00000000000000888, 3.000000000000002665, 5.000000000000000888 ) ) ;
#6475=EDGE_CURVE ( 'NONE', #1368, #8806, #7438, .T. ) ;
#6476=AXIS2_PLACEMENT_3D ( 'NONE', #2717, #7863, #4096 ) ;
#6479=DIRECTION ( 'NONE',  ( -6.505213034913038160E-19, -3.903127820947822896E-18, -1.000000000000000000 ) ) ;
#6480=DIRECTION ( 'NONE',  ( -1.000000000000000000, 0.000000000000000000, 0.000000000000000000 ) ) ;
#6481=DIRECTION ( 'NONE',  ( -1.000000000000000000, -1.208970125616060101E-17, 6.505213034913038160E-19 ) ) ;
#6484=EDGE_CURVE ( 'NONE', #9968, #17215, #686, .T. ) ;
#6486=ORIENTED_EDGE ( 'NONE', *, *, #12226, .F. ) ;
#6487=EDGE_CURVE ( 'NONE', #2718, #19753, #19719, .T. ) ;
#6490=CARTESIAN_POINT ( 'NONE',  ( 16.56444186175090749, -26.79308242454900224, -7.000000000000006217 ) ) ;
#6492=TOROIDAL_SURFACE ( 'NONE', #15238, 34.90673715956759082, 8.750000000000000000 ) ;
#6495=CIRCLE ( 'NONE', #18569, 1.000000000000000888 ) ;
#6496=DIRECTION ( 'NONE',  ( 6.505213034913038160E-19, 3.903127820947822896E-18, 1.000000000000000000 ) ) ;
#6497=EDGE_LOOP ( 'NONE', ( #18272, #14911, #16477, #5249 ) ) ;
#6501=DIRECTION ( 'NONE',  ( 6.505213034913038160E-19, 3.903127820947822896E-18, 1.000000000000000000 ) ) ;
#6507=CYLINDRICAL_SURFACE ( 'NONE', #4939, 31.50000000000001421 ) ;
#6508=VERTEX_POINT ( 'NONE', #9272 ) ;
#6513=AXIS2_PLACEMENT_3D ( 'NONE', #1688, #11996, #5135 ) ;
#6515=AXIS2_PLACEMENT_3D ( 'NONE', #21399, #14159, #14272 ) ;
#6520=ORIENTED_EDGE ( 'NONE', *, *, #1714, .F. ) ;
#6521=CYLINDRICAL_SURFACE ( 'NONE', #16984, 36.76383501243555685 ) ;
#6525=CYLINDRICAL_SURFACE ( 'NONE', #1116, 31.50000000000000711 ) ;
#6528=ADVANCED_FACE ( 'NONE', ( #8234 ), #6521, .T. ) ;
#6530=DIRECTION ( 'NONE',  ( -6.505213034913038160E-19, -3.903127820947822896E-18, -1.000000000000000000 ) ) ;
#6532=AXIS2_PLACEMENT_3D ( 'NONE', #8600, #12, #1507 ) ;
#6533=LINE ( 'NONE', #22349, #15173 ) ;
#6536=CARTESIAN_POINT ( 'NONE',  ( -31.09841355225989545, 5.093313992686310243, -2.999999999999971578 ) ) ;
#6542=FACE_OUTER_BOUND ( 'NONE', #21338, .T. ) ;
#6543=CARTESIAN_POINT ( 'NONE',  ( 24.10117729468400682, -26.10603996529641080, 3.000000000000047518 ) ) ;
#6545=DIRECTION ( 'NONE',  ( 6.505213034913038160E-19, 3.903127820947822896E-18, 1.000000000000000000 ) ) ;
#6552=CARTESIAN_POINT ( 'NONE',  ( 2.775557561562891351E-14, -2.775557561562891351E-14, 2.999999999999999112 ) ) ;
#6554=ADVANCED_FACE ( 'NONE', ( #18551 ), #18668, .T. ) ;
#6556=CIRCLE ( 'NONE', #8018, 31.50000000000000711 ) ;
#6562=EDGE_LOOP ( 'NONE', ( #1993, #18778, #11951, #852, #15513, #17316 ) ) ;
#6563=DIRECTION ( 'NONE',  ( -1.000000000000000000, -1.208970125616060717E-17, 0.000000000000000000 ) ) ;
#6570=VERTEX_POINT ( 'NONE', #9944 ) ;
#6587=VERTEX_POINT ( 'NONE', #14975 ) ;
#6588=CYLINDRICAL_SURFACE ( 'NONE', #20073, 3.000000000000000888 ) ;
#6593=DIRECTION ( 'NONE',  ( 6.505213034913038160E-19, 3.903127820947822896E-18, 1.000000000000000000 ) ) ;
#6600=ADVANCED_FACE ( 'NONE', ( #22690 ), #11122, .T. ) ;
#6602=VERTEX_POINT ( 'NONE', #19352 ) ;
#6605=CYLINDRICAL_SURFACE ( 'NONE', #9622, 19.11328065563151668 ) ;
#6620=DIRECTION ( 'NONE',  ( 6.505213034913038160E-19, 3.903127820947822896E-18, 1.000000000000000000 ) ) ;
#6623=AXIS2_PLACEMENT_3D ( 'NONE', #1657, #18963, #7031 ) ;
#6624=ORIENTED_EDGE ( 'NONE', *, *, #20999, .F. ) ;
#6625=ADVANCED_FACE ( 'NONE', ( #2032 ), #1244, .T. ) ;
#6627=ORIENTED_EDGE ( 'NONE', *, *, #6887, .F. ) ;
#6628=DIRECTION ( 'NONE',  ( -6.505213034913038160E-19, -3.903127820947822896E-18, -1.000000000000000000 ) ) ;
#6631=DIRECTION ( 'NONE',  ( 1.000000000000000000, 0.000000000000000000, 0.000000000000000000 ) ) ;
#6636=LINE ( 'NONE', #8695, #3970 ) ;
#6650=CARTESIAN_POINT ( 'NONE',  ( -32.40961249803547872, 2.422192751863922133, 2.999999999999999112 ) ) ;
#6651=VECTOR ( 'NONE', #5875, 1000.000000000000000 ) ;
#6652=EDGE_CURVE ( 'NONE', #22056, #6570, #10279, .T. ) ;
#6654=EDGE_CURVE ( 'NONE', #19154, #8041, #20276, .T. ) ;
#6666=ORIENTED_EDGE ( 'NONE', *, *, #11764, .F. ) ;
#6668=DIRECTION ( 'NONE',  ( -6.505213034913038160E-19, -3.903127820947822896E-18, -1.000000000000000000 ) ) ;
#6669=CIRCLE ( 'NONE', #19478, 31.50000000000000000 ) ;
#6672=ORIENTED_EDGE ( 'NONE', *, *, #22688, .T. ) ;
#6687=VECTOR ( 'NONE', #4307, 1000.000000000000000 ) ;
#6692=ORIENTED_EDGE ( 'NONE', *, *, #3394, .F. ) ;
#6693=DIRECTION ( 'NONE',  ( -6.505213034913038160E-19, -3.903127820947822896E-18, -1.000000000000000000 ) ) ;
#6696=EDGE_LOOP ( 'NONE', ( #143, #22633, #13403, #4222 ) ) ;
#6697=DIRECTION ( 'NONE',  ( -6.505213034913038160E-19, -3.903127820947822896E-18, -1.000000000000000000 ) ) ;
#6698=CARTESIAN_POINT ( 'NONE',  ( 2.775557561562891351E-14, -2.775557561562891351E-14, 2.999999999999999112 ) ) ;
#6701=CARTESIAN_POINT ( 'NONE',  ( -15.02862401740807918, -32.75570538720779012, -6.999999999999950262 ) ) ;
#6707=AXIS2_PLACEMENT_3D ( 'NONE', #3255, #15482, #13975 ) ;
#6710=ORIENTED_EDGE ( 'NONE', *, *, #19425, .F. ) ;
#6715=CARTESIAN_POINT ( 'NONE',  ( 26.79308242454897382, 16.56444186175074051, -6.999999999999944045 ) ) ;
#6716=CARTESIAN_POINT ( 'NONE',  ( -11.85401191286884703, -32.83234229683740324, -2.999999999999971578 ) ) ;
#6717=CIRCLE ( 'NONE', #9636, 22.00000000000000711 ) ;
#6722=CIRCLE ( 'NONE', #5615, 22.00000000000000000 ) ;
#6723=ADVANCED_FACE ( 'NONE', ( #16573 ), #2154, .T. ) ;
#6730=EDGE_CURVE ( 'NONE', #2407, #9840, #14029, .T. ) ;
#6734=ORIENTED_EDGE ( 'NONE', *, *, #4883, .F. ) ;
#6741=ORIENTED_EDGE ( 'NONE', *, *, #18691, .F. ) ;
#6744=CARTESIAN_POINT ( 'NONE',  ( 27.64365646977290325, 17.09029715894935819, 2.999999999999995559 ) ) ;
#6748=VECTOR ( 'NONE', #17135, 1000.000000000000000 ) ;
#6757=ORIENTED_EDGE ( 'NONE', *, *, #15461, .F. ) ;
#6768=EDGE_LOOP ( 'NONE', ( #12967, #20749, #12741, #13414 ) ) ;
#6771=EDGE_LOOP ( 'NONE', ( #7631, #2894, #9433, #2605 ) ) ;
#6778=ORIENTED_EDGE ( 'NONE', *, *, #15566, .F. ) ;
#6779=CARTESIAN_POINT ( 'NONE',  ( -10.70799354677365400, 35.16985127952393242, -1.999999999999977573 ) ) ;
#6781=ORIENTED_EDGE ( 'NONE', *, *, #11725, .F. ) ;
#6785=CARTESIAN_POINT ( 'NONE',  ( -27.84804035626026320, 24.75236754129139882, -6.999999999999964473 ) ) ;
#6790=ORIENTED_EDGE ( 'NONE', *, *, #2266, .T. ) ;
#6791=CARTESIAN_POINT ( 'NONE',  ( -32.09841355225981374, 5.093313992686310243, -7.000000000000006217 ) ) ;
#6792=CARTESIAN_POINT ( 'NONE',  ( 0.6841746959067585010, 36.75746821813302745, -2.800654218530457484 ) ) ;
#6793=CARTESIAN_POINT ( 'NONE',  ( 1.010906942018275689, 35.52192638951967041, 3.000000000000061284 ) ) ;
#6795=AXIS2_PLACEMENT_3D ( 'NONE', #20466, #13787, #6480 ) ;
#6800=AXIS2_PLACEMENT_3D ( 'NONE', #12776, #5803, #72 ) ;
#6804=EDGE_CURVE ( 'NONE', #1088, #18716, #20283, .T. ) ;
#6807=ORIENTED_EDGE ( 'NONE', *, *, #11835, .T. ) ;
#6818=CARTESIAN_POINT ( 'NONE',  ( -34.74700806321096280, 12.00937115242622966, -2.800654218530460593 ) ) ;
#6824=CARTESIAN_POINT ( 'NONE',  ( 2.775557561562891351E-14, 2.775557561562891351E-14, 5.750000000000001776 ) ) ;
#6825=CARTESIAN_POINT ( 'NONE',  ( 2.220446049250313081E-13, 2.775557561562891351E-14, -2.800654218530485018 ) ) ;
#6827=DIRECTION ( 'NONE',  ( 1.000000000000000000, 0.000000000000000000, 0.000000000000000000 ) ) ;
#6828=CARTESIAN_POINT ( 'NONE',  ( -1.010906942018023225, -35.52192638951984804, 3.000000000000060840 ) ) ;
#6834=EDGE_LOOP ( 'NONE', ( #17243, #16439, #10778, #13225 ) ) ;
#6837=DIRECTION ( 'NONE',  ( -6.505213034913038160E-19, -3.903127820947822896E-18, -1.000000000000000000 ) ) ;
#6842=ADVANCED_FACE ( 'NONE', ( #995 ), #20139, .T. ) ;
#6843=EDGE_CURVE ( 'NONE', #12187, #6131, #9701, .T. ) ;
#6844=ORIENTED_EDGE ( 'NONE', *, *, #1467, .F. ) ;
#6848=FACE_OUTER_BOUND ( 'NONE', #4910, .T. ) ;
#6850=DIRECTION ( 'NONE',  ( 6.505213034913038160E-19, 3.903127820947822896E-18, 1.000000000000000000 ) ) ;
#6851=ORIENTED_EDGE ( 'NONE', *, *, #6852, .F. ) ;
#6852=EDGE_CURVE ( 'NONE', #18279, #19756, #1213, .T. ) ;
#6854=AXIS2_PLACEMENT_3D ( 'NONE', #21348, #382, #263 ) ;
#6859=VERTEX_POINT ( 'NONE', #4556 ) ;
#6861=VECTOR ( 'NONE', #7425, 1000.000000000000000 ) ;
#6872=AXIS2_PLACEMENT_3D ( 'NONE', #16525, #7368, #3940 ) ;
#6882=DIRECTION ( 'NONE',  ( -1.000000000000000000, -3.564803380056654458E-15, 0.000000000000000000 ) ) ;
#6883=EDGE_CURVE ( 'NONE', #8806, #2631, #1451, .T. ) ;
#6884=AXIS2_PLACEMENT_3D ( 'NONE', #13142, #16246, #5837 ) ;
#6887=EDGE_CURVE ( 'NONE', #18451, #7988, #9925, .T. ) ;
#6892=CIRCLE ( 'NONE', #18612, 0.9999999999999995559 ) ;
#6893=EDGE_LOOP ( 'NONE', ( #15167, #8674, #10959, #21929, #10474, #15117 ) ) ;
#6894=CARTESIAN_POINT ( 'NONE',  ( -31.92986134326215719, 18.22261011550257948, -1.999999999999998224 ) ) ;
#6896=DIRECTION ( 'NONE',  ( -1.000000000000000000, 0.000000000000000000, 0.000000000000000000 ) ) ;
#6898=CARTESIAN_POINT ( 'NONE',  ( -32.75570538720774749, 15.02862401740778786, 2.999999999999995559 ) ) ;
#6900=CARTESIAN_POINT ( 'NONE',  ( 7.463862311151453710, 35.99819890246943999, -2.800654218530457484 ) ) ;
#6901=CARTESIAN_POINT ( 'NONE',  ( 30.48934413892814987, -16.99647590252656570, -2.999999999999971578 ) ) ;
#6908=EDGE_CURVE ( 'NONE', #1434, #19293, #13458, .T. ) ;
#6918=CIRCLE ( 'NONE', #22664, 19.11328065563151668 ) ;
#6921=EDGE_CURVE ( 'NONE', #928, #20565, #17300, .T. ) ;
#6925=ORIENTED_EDGE ( 'NONE', *, *, #22440, .T. ) ;
#6926=FACE_OUTER_BOUND ( 'NONE', #11165, .T. ) ;
#6930=ORIENTED_EDGE ( 'NONE', *, *, #182, .F. ) ;
#6931=CARTESIAN_POINT ( 'NONE',  ( 8.326672684688674053E-14, -28.00000000000013500, 2.999999999999995559 ) ) ;
#6944=DIRECTION ( 'NONE',  ( 6.505213034913038160E-19, 3.903127820947822896E-18, 1.000000000000000000 ) ) ;
#6945=EDGE_CURVE ( 'NONE', #4146, #19820, #8900, .T. ) ;
#6946=DIRECTION ( 'NONE',  ( -6.505213034913038160E-19, -3.903127820947822896E-18, -1.000000000000000000 ) ) ;
#6947=ORIENTED_EDGE ( 'NONE', *, *, #7964, .F. ) ;
#6948=ORIENTED_EDGE ( 'NONE', *, *, #6421, .F. ) ;
#6951=EDGE_LOOP ( 'NONE', ( #10202, #13480, #22293, #16347, #5814 ) ) ;
#6955=EDGE_CURVE ( 'NONE', #12492, #6587, #4669, .T. ) ;
#6957=CARTESIAN_POINT ( 'NONE',  ( -14.29266125237886520, 28.07080038625062102, -2.999999999999978240 ) ) ;
#6959=ADVANCED_FACE ( 'NONE', ( #15172 ), #1332, .T. ) ;
#6960=ORIENTED_EDGE ( 'NONE', *, *, #12490, .F. ) ;
#6961=CARTESIAN_POINT ( 'NONE',  ( -20.00948735876860596, -24.79619811426206510, 2.999999999999995559 ) ) ;
#6966=ORIENTED_EDGE ( 'NONE', *, *, #2962, .T. ) ;
#6967=CYLINDRICAL_SURFACE ( 'NONE', #8070, 3.000000000000002665 ) ;
#6969=CIRCLE ( 'NONE', #18674, 34.90673715956759082 ) ;
#6972=ADVANCED_FACE ( 'NONE', ( #22322 ), #6605, .T. ) ;
#6977=AXIS2_PLACEMENT_3D ( 'NONE', #4166, #14338, #2326 ) ;
#6978=EDGE_CURVE ( 'NONE', #3604, #21131, #15570, .T. ) ;
#6986=ORIENTED_EDGE ( 'NONE', *, *, #9100, .T. ) ;
#6987=CARTESIAN_POINT ( 'NONE',  ( 21.05198877411809733, -30.13956425491237567, -2.000000000000005329 ) ) ;
#6989=CARTESIAN_POINT ( 'NONE',  ( 3.608224830031758756E-13, -2.775557561562891351E-14, -4.999999999999997335 ) ) ;
#6995=EDGE_CURVE ( 'NONE', #4971, #22365, #10256, .T. ) ;
#7005=DIRECTION ( 'NONE',  ( -6.505213034913038160E-19, -3.903127820947822896E-18, -1.000000000000000000 ) ) ;
#7006=DIRECTION ( 'NONE',  ( 6.505213034913038160E-19, 3.903127820947822896E-18, 1.000000000000000000 ) ) ;
#7007=ORIENTED_EDGE ( 'NONE', *, *, #6908, .T. ) ;
#7010=FACE_OUTER_BOUND ( 'NONE', #2434, .T. ) ;
#7013=VERTEX_POINT ( 'NONE', #20820 ) ;
#7014=CARTESIAN_POINT ( 'NONE',  ( 2.347663744114436568, 31.41239365194195443, 3.000000000000009770 ) ) ;
#7016=ORIENTED_EDGE ( 'NONE', *, *, #12763, .F. ) ;
#7017=EDGE_CURVE ( 'NONE', #9840, #15288, #13617, .T. ) ;
#7022=ORIENTED_EDGE ( 'NONE', *, *, #16055, .F. ) ;
#7023=ORIENTED_EDGE ( 'NONE', *, *, #9506, .T. ) ;
#7024=DIRECTION ( 'NONE',  ( -1.000000000000000000, -1.208970125616060101E-17, 6.505213034913038160E-19 ) ) ;
#7031=DIRECTION ( 'NONE',  ( 1.000000000000000000, 1.208970125616053475E-17, 0.000000000000000000 ) ) ;
#7033=CARTESIAN_POINT ( 'NONE',  ( 35.99819890246974552, -7.463862311151231665, 2.800654218530509443 ) ) ;
#7034=B_SPLINE_CURVE_WITH_KNOTS ( 'NONE', 3,
 ( #17099, #12065, #22623, #5090 ),
 .UNSPECIFIED., .F., .F.,
 ( 4, 4 ),
 ( 9.545285770394248685E-07, 0.001900595205834785563 ),
 .UNSPECIFIED. ) ;
#7037=ORIENTED_EDGE ( 'NONE', *, *, #8536, .F. ) ;
#7038=DIRECTION ( 'NONE',  ( -6.505213034913038160E-19, -3.903127820947822896E-18, -1.000000000000000000 ) ) ;
#7047=ORIENTED_EDGE ( 'NONE', *, *, #4570, .T. ) ;
#7050=ORIENTED_EDGE ( 'NONE', *, *, #20302, .F. ) ;
#7053=CARTESIAN_POINT ( 'NONE',  ( 18.00000000000035882, -2.753796099301802219E-14, -4.999999999999997335 ) ) ;
#7054=CYLINDRICAL_SURFACE ( 'NONE', #8714, 19.11328065563151668 ) ;
#7057=ORIENTED_EDGE ( 'NONE', *, *, #2140, .F. ) ;
#7058=DIRECTION ( 'NONE',  ( -1.000000000000000000, -1.815202222194848078E-15, 0.000000000000000000 ) ) ;
#7062=VECTOR ( 'NONE', #12092, 1000.000000000000000 ) ;
#7065=CARTESIAN_POINT ( 'NONE',  ( 2.220446049250313081E-13, 2.775557561562891351E-14, -2.800654218530485018 ) ) ;
#7070=EDGE_CURVE ( 'NONE', #7013, #13252, #7100, .T. ) ;
#7073=ORIENTED_EDGE ( 'NONE', *, *, #11296, .T. ) ;
#7075=DIRECTION ( 'NONE',  ( -1.000000000000000000, -1.208970125616057944E-17, 0.000000000000000000 ) ) ;
#7076=ADVANCED_FACE ( 'NONE', ( #10695 ), #1678, .F. ) ;
#7077=EDGE_CURVE ( 'NONE', #2772, #9581, #15841, .T. ) ;
#7078=ADVANCED_FACE ( 'NONE', ( #5455 ), #8533, .T. ) ;
#7083=CARTESIAN_POINT ( 'NONE',  ( 27.57461708434186320, -4.862148974673824675, 2.999999999999995559 ) ) ;
#7087=ORIENTED_EDGE ( 'NONE', *, *, #18322, .F. ) ;
#7092=DIRECTION ( 'NONE',  ( -6.505213034913038160E-19, -3.903127820947822896E-18, -1.000000000000000000 ) ) ;
#7095=ORIENTED_EDGE ( 'NONE', *, *, #19323, .F. ) ;
#7100=B_SPLINE_CURVE_WITH_KNOTS ( 'NONE', 3,
 ( #6716, #15519, #5342, #12100 ),
 .UNSPECIFIED., .F., .F.,
 ( 4, 4 ),
 ( 0.001893031756884946092, 0.003808480026563296206 ),
 .UNSPECIFIED. ) ;
#7106=DIRECTION ( 'NONE',  ( -6.505213034913038160E-19, -3.903127820947822896E-18, -1.000000000000000000 ) ) ;
#7108=ORIENTED_EDGE ( 'NONE', *, *, #16216, .F. ) ;
#7114=EDGE_CURVE ( 'NONE', #1508, #18491, #11454, .T. ) ;
#7116=ORIENTED_EDGE ( 'NONE', *, *, #5467, .T. ) ;
#7123=CYLINDRICAL_SURFACE ( 'NONE', #18862, 19.11328065563151668 ) ;
#7126=ORIENTED_EDGE ( 'NONE', *, *, #8412, .F. ) ;
#7139=ORIENTED_EDGE ( 'NONE', *, *, #1448, .T. ) ;
#7141=FACE_OUTER_BOUND ( 'NONE', #7840, .T. ) ;
#7148=AXIS2_PLACEMENT_3D ( 'NONE', #8697, #15553, #10732 ) ;
#7150=FACE_OUTER_BOUND ( 'NONE', #18446, .T. ) ;
#7154=ORIENTED_EDGE ( 'NONE', *, *, #11663, .F. ) ;
#7159=ORIENTED_EDGE ( 'NONE', *, *, #5380, .T. ) ;
#7161=ADVANCED_FACE ( 'NONE', ( #10817 ), #18276, .T. ) ;
#7163=CIRCLE ( 'NONE', #21424, 19.11328065563151668 ) ;
#7165=DIRECTION ( 'NONE',  ( -1.000000000000000000, -1.208970125616081209E-17, 0.000000000000000000 ) ) ;
#7168=ORIENTED_EDGE ( 'NONE', *, *, #11911, .T. ) ;
#7169=CARTESIAN_POINT ( 'NONE',  ( 33.52953626616048410, 9.708269511265299911, 2.999999999999995559 ) ) ;
#7177=TOROIDAL_SURFACE ( 'NONE', #19997, 34.90673715956759082, 8.750000000000000000 ) ;
#7178=CIRCLE ( 'NONE', #13014, 34.90673715956759082 ) ;
#7191=DIRECTION ( 'NONE',  ( -1.000000000000000000, 1.070969311094960327E-14, 0.000000000000000000 ) ) ;
#7196=AXIS2_PLACEMENT_3D ( 'NONE', #2162, #14735, #9595 ) ;
#7199=FACE_OUTER_BOUND ( 'NONE', #1220, .T. ) ;
#7205=CIRCLE ( 'NONE', #9042, 19.11328065563150957 ) ;
#7206=CARTESIAN_POINT ( 'NONE',  ( 3.330669073875469621E-13, -1.110223024625156540E-13, -2.999999999999971578 ) ) ;
#7209=CIRCLE ( 'NONE', #15244, 3.000000000000002665 ) ;
#7215=CARTESIAN_POINT ( 'NONE',  ( -17.99999999999963762, -2.565454789329504983E-14, -4.999999999999997335 ) ) ;
#7216=VECTOR ( 'NONE', #7006, 1000.000000000000000 ) ;
#7219=DIRECTION ( 'NONE',  ( 1.000000000000000000, 0.000000000000000000, 0.000000000000000000 ) ) ;
#7220=CIRCLE ( 'NONE', #5778, 22.00000000000000711 ) ;
#7222=CARTESIAN_POINT ( 'NONE',  ( 12.00937115242647835, 34.74700806321096280, 2.800654218530512551 ) ) ;
#7226=CARTESIAN_POINT ( 'NONE',  ( 14.76298474240519987, 28.95348479018566934, -2.999999999999999112 ) ) ;
#7230=CARTESIAN_POINT ( 'NONE',  ( 28.06260833510335218, -14.30873905802357271, -7.000000000000006217 ) ) ;
#7236=ORIENTED_EDGE ( 'NONE', *, *, #2467, .T. ) ;
#7238=DIRECTION ( 'NONE',  ( 6.505213034913038160E-19, 3.903127820947822896E-18, 1.000000000000000000 ) ) ;
#7243=CIRCLE ( 'NONE', #12369, 1.000000000000000888 ) ;
#7253=AXIS2_PLACEMENT_3D ( 'NONE', #7461, #3476, #17894 ) ;
#7258=ORIENTED_EDGE ( 'NONE', *, *, #10724, .F. ) ;
#7259=DIRECTION ( 'NONE',  ( 6.505213034913038160E-19, 3.903127820947822896E-18, 1.000000000000000000 ) ) ;
#7266=ORIENTED_EDGE ( 'NONE', *, *, #7313, .T. ) ;
#7267=CARTESIAN_POINT ( 'NONE',  ( 5.551115123125782702E-14, -1.387778780781445676E-13, -5.749999999999949374 ) ) ;
#7270=AXIS2_PLACEMENT_3D ( 'NONE', #17758, #21312, #8935 ) ;
#7273=DIRECTION ( 'NONE',  ( 1.000000000000000000, 0.000000000000000000, 0.000000000000000000 ) ) ;
#7276=CARTESIAN_POINT ( 'NONE',  ( -26.64693883069154623, -24.43377932785630335, -2.933296326616347205 ) ) ;
#7277=VECTOR ( 'NONE', #8444, 1000.000000000000000 ) ;
#7287=DIRECTION ( 'NONE',  ( 6.505213034913038160E-19, 3.903127820947822896E-18, 1.000000000000000000 ) ) ;
#7293=DIRECTION ( 'NONE',  ( 6.505213034913038160E-19, 3.903127820947822896E-18, 1.000000000000000000 ) ) ;
#7294=CIRCLE ( 'NONE', #16059, 19.11328065563151668 ) ;
#7295=CARTESIAN_POINT ( 'NONE',  ( 36.54278193890323223, 4.025500340002318822, -2.000000000000005329 ) ) ;
#7298=EDGE_CURVE ( 'NONE', #728, #2190, #14742, .T. ) ;
#7299=CARTESIAN_POINT ( 'NONE',  ( 2.220446049250313081E-13, 2.775557561562891351E-14, -2.800654218530485018 ) ) ;
#7305=ORIENTED_EDGE ( 'NONE', *, *, #13581, .F. ) ;
#7307=EDGE_LOOP ( 'NONE', ( #7690, #14541, #3816, #14206 ) ) ;
#7311=CARTESIAN_POINT ( 'NONE',  ( 5.551115123125782702E-14, -1.387778780781445676E-13, -5.749999999999949374 ) ) ;
#7313=EDGE_CURVE ( 'NONE', #13542, #19759, #22296, .T. ) ;
#7315=DIRECTION ( 'NONE',  ( -6.505213034913038160E-19, -3.903127820947822896E-18, -1.000000000000000000 ) ) ;
#7316=VECTOR ( 'NONE', #6392, 1000.000000000000000 ) ;
#7318=DIRECTION ( 'NONE',  ( -6.505213034913038160E-19, -3.903127820947822896E-18, -1.000000000000000000 ) ) ;
#7327=CARTESIAN_POINT ( 'NONE',  ( -4.936596639065260916, -31.11077005834428277, 2.999999999999999112 ) ) ;
#7328=AXIS2_PLACEMENT_3D ( 'NONE', #20958, #3549, #10967 ) ;
#7336=DIRECTION ( 'NONE',  ( 6.505213034913038160E-19, 3.903127820947822896E-18, 1.000000000000000000 ) ) ;
#7338=ORIENTED_EDGE ( 'NONE', *, *, #17720, .T. ) ;
#7341=EDGE_CURVE ( 'NONE', #16319, #17133, #7444, .T. ) ;
#7343=AXIS2_PLACEMENT_3D ( 'NONE', #10336, #11958, #15270 ) ;
#7345=ORIENTED_EDGE ( 'NONE', *, *, #5726, .F. ) ;
#7346=DIRECTION ( 'NONE',  ( 1.208970125616062874E-17, -1.000000000000000000, 3.903127820947822896E-18 ) ) ;
#7349=ORIENTED_EDGE ( 'NONE', *, *, #11747, .F. ) ;
#7350=CARTESIAN_POINT ( 'NONE',  ( 19.05255888325788050, 10.99999999999995381, -5.000000000000004441 ) ) ;
#7354=ADVANCED_FACE ( 'NONE', ( #6351 ), #19297, .T. ) ;
#7356=CIRCLE ( 'NONE', #14289, 34.90673715956759082 ) ;
#7362=DIRECTION ( 'NONE',  ( -6.505213034913038160E-19, -3.903127820947822896E-18, -1.000000000000000000 ) ) ;
#7368=DIRECTION ( 'NONE',  ( 6.505213034913038160E-19, 3.903127820947822896E-18, 1.000000000000000000 ) ) ;
#7370=B_SPLINE_CURVE_WITH_KNOTS ( 'NONE', 3,
 ( #9171, #19605, #14546, #7452 ),
 .UNSPECIFIED., .F., .F.,
 ( 4, 4 ),
 ( 0.001893031756885420322, 0.003808480026563612359 ),
 .UNSPECIFIED. ) ;
#7383=ORIENTED_EDGE ( 'NONE', *, *, #5167, .T. ) ;
#7385=EDGE_CURVE ( 'NONE', #13841, #13545, #8411, .T. ) ;
#7388=ORIENTED_EDGE ( 'NONE', *, *, #20076, .F. ) ;
#7398=CARTESIAN_POINT ( 'NONE',  ( -32.35999952201570551, 1.423424233832487618, -2.999999999999971578 ) ) ;
#7401=DIRECTION ( 'NONE',  ( -6.505213034913038160E-19, -3.903127820947822896E-18, -1.000000000000000000 ) ) ;
#7406=CARTESIAN_POINT ( 'NONE',  ( 27.84804035626065044, -24.75236754129175765, -2.999999999999971578 ) ) ;
#7407=FACE_BOUND ( 'NONE', #6696, .T. ) ;
#7410=ORIENTED_EDGE ( 'NONE', *, *, #18573, .T. ) ;
#7411=VERTEX_POINT ( 'NONE', #10449 ) ;
#7415=CARTESIAN_POINT ( 'NONE',  ( 2.220446049250313081E-13, -2.498001805406602216E-13, -6.859353255829918616 ) ) ;
#7418=DIRECTION ( 'NONE',  ( 6.505213034913038160E-19, 3.903127820947822896E-18, 1.000000000000000000 ) ) ;
#7419=CARTESIAN_POINT ( 'NONE',  ( -3.656418565264218934, -37.07861450834831629, -2.999999999999957367 ) ) ;
#7424=ORIENTED_EDGE ( 'NONE', *, *, #15444, .F. ) ;
#7425=DIRECTION ( 'NONE',  ( 6.505213034913038160E-19, 3.903127820947822896E-18, 1.000000000000000000 ) ) ;
#7426=DIRECTION ( 'NONE',  ( 1.000000000000000000, 0.000000000000000000, 0.000000000000000000 ) ) ;
#7427=FACE_OUTER_BOUND ( 'NONE', #13586, .T. ) ;
#7428=CARTESIAN_POINT ( 'NONE',  ( 27.57461708434208347, -4.862148974673990764, -5.000000000000004441 ) ) ;
#7434=CIRCLE ( 'NONE', #3424, 2.999999999999999112 ) ;
#7438=LINE ( 'NONE', #14413, #8564 ) ;
#7444=CIRCLE ( 'NONE', #21358, 31.50000000000001421 ) ;
#7447=DIRECTION ( 'NONE',  ( -1.000000000000000000, 0.000000000000000000, 0.000000000000000000 ) ) ;
#7452=CARTESIAN_POINT ( 'NONE',  ( -29.33526866242094755, 22.15900668633769044, -2.800654218530477912 ) ) ;
#7455=CARTESIAN_POINT ( 'NONE',  ( 20.36304159388363644, 24.03323817228475434, -6.999999999999992006 ) ) ;
#7460=ORIENTED_EDGE ( 'NONE', *, *, #14498, .F. ) ;
#7461=CARTESIAN_POINT ( 'NONE',  ( 12.31876324338299078, 30.07487443287970663, 3.000000000000023537 ) ) ;
#7462=CIRCLE ( 'NONE', #2714, 19.11328065563150957 ) ;
#7463=ADVANCED_FACE ( 'NONE', ( #18538 ), #1947, .T. ) ;
#7464=DIRECTION ( 'NONE',  ( -6.505213034913038160E-19, -3.903127820947822896E-18, -1.000000000000000000 ) ) ;
#7468=CIRCLE ( 'NONE', #20287, 8.999999999999998224 ) ;
#7469=EDGE_LOOP ( 'NONE', ( #9672, #20120, #4372, #849 ) ) ;
#7470=ORIENTED_EDGE ( 'NONE', *, *, #10938, .T. ) ;
#7471=ORIENTED_EDGE ( 'NONE', *, *, #13692, .F. ) ;
#7473=ORIENTED_EDGE ( 'NONE', *, *, #1783, .F. ) ;
#7476=CARTESIAN_POINT ( 'NONE',  ( -28.88846368933341324, -19.59430950039328678, 2.999999999999995559 ) ) ;
#7479=ORIENTED_EDGE ( 'NONE', *, *, #10376, .F. ) ;
#7486=VERTEX_POINT ( 'NONE', #18414 ) ;
#7491=CARTESIAN_POINT ( 'NONE',  ( -14.30873905802343415, -28.06260833510307151, -6.999999999999950262 ) ) ;
#7498=CARTESIAN_POINT ( 'NONE',  ( 17.38334492574566070, 30.99230043872318419, -3.000000000000006217 ) ) ;
#7500=AXIS2_PLACEMENT_3D ( 'NONE', #14523, #21535, #20156 ) ;
#7504=EDGE_CURVE ( 'NONE', #20345, #4779, #6717, .T. ) ;
#7506=ORIENTED_EDGE ( 'NONE', *, *, #7919, .T. ) ;
#7507=ORIENTED_EDGE ( 'NONE', *, *, #2239, .T. ) ;
#7508=CARTESIAN_POINT ( 'NONE',  ( -24.79619811426206510, 21.00948735876881202, -6.999999999999950262 ) ) ;
#7515=CIRCLE ( 'NONE', #4588, 34.90673715956759082 ) ;
#7517=ORIENTED_EDGE ( 'NONE', *, *, #5227, .T. ) ;
#7520=CARTESIAN_POINT ( 'NONE',  ( -34.74700806321096280, 12.00937115242622966, -2.800654218530460593 ) ) ;
#7529=VECTOR ( 'NONE', #5593, 1000.000000000000000 ) ;
#7535=CARTESIAN_POINT ( 'NONE',  ( -35.33352588067087652, -7.094908322883425100, -2.999999999999971578 ) ) ;
#7536=CYLINDRICAL_SURFACE ( 'NONE', #18318, 1.000000000000000888 ) ;
#7537=EDGE_CURVE ( 'NONE', #18815, #18105, #8193, .T. ) ;
#7546=DIRECTION ( 'NONE',  ( 6.505213034913038160E-19, 3.903127820947822896E-18, 1.000000000000000000 ) ) ;
#7548=CIRCLE ( 'NONE', #21828, 19.11328065563152379 ) ;
#7552=DIRECTION ( 'NONE',  ( -6.505213034913038160E-19, -3.903127820947822896E-18, -1.000000000000000000 ) ) ;
#7553=ORIENTED_EDGE ( 'NONE', *, *, #3537, .T. ) ;
#7557=ORIENTED_EDGE ( 'NONE', *, *, #21057, .F. ) ;
#7560=DIRECTION ( 'NONE',  ( -6.505213034913038160E-19, -3.903127820947822896E-18, -1.000000000000000000 ) ) ;
#7569=LINE ( 'NONE', #17650, #6291 ) ;
#7570=EDGE_LOOP ( 'NONE', ( #7116, #20861, #6434, #8460 ) ) ;
#7571=CARTESIAN_POINT ( 'NONE',  ( -36.75746821813305587, 0.6841746959067307454, 2.800654218530485018 ) ) ;
#7576=ORIENTED_EDGE ( 'NONE', *, *, #12441, .F. ) ;
#7580=VERTEX_POINT ( 'NONE', #14602 ) ;
#7582=ORIENTED_EDGE ( 'NONE', *, *, #69, .F. ) ;
#7583=VECTOR ( 'NONE', #21240, 1000.000000000000000 ) ;
#7585=AXIS2_PLACEMENT_3D ( 'NONE', #5021, #10925, #7273 ) ;
#7586=ORIENTED_EDGE ( 'NONE', *, *, #6921, .T. ) ;
#7589=CARTESIAN_POINT ( 'NONE',  ( -21.00948735876882623, -24.79619811426206510, -6.999999999999950262 ) ) ;
#7592=ORIENTED_EDGE ( 'NONE', *, *, #12367, .F. ) ;
#7594=FACE_OUTER_BOUND ( 'NONE', #14440, .T. ) ;
#7596=FACE_OUTER_BOUND ( 'NONE', #5100, .T. ) ;
#7598=DIRECTION ( 'NONE',  ( 6.505213034913038160E-19, 3.903127820947822896E-18, 1.000000000000000000 ) ) ;
#7599=VERTEX_POINT ( 'NONE', #21488 ) ;
#7603=CARTESIAN_POINT ( 'NONE',  ( 2.775557561562891351E-14, -2.775557561562891351E-14, 2.999999999999999112 ) ) ;
#7610=AXIS2_PLACEMENT_3D ( 'NONE', #3184, #4680, #11655 ) ;
#7612=CARTESIAN_POINT ( 'NONE',  ( 25.58633464742632313, 23.74488952252767859, -2.999999999999971578 ) ) ;
#7613=EDGE_CURVE ( 'NONE', #6403, #13845, #417, .T. ) ;
#7614=DIRECTION ( 'NONE',  ( 1.000000000000000000, 0.000000000000000000, 0.000000000000000000 ) ) ;
#7618=ORIENTED_EDGE ( 'NONE', *, *, #18490, .F. ) ;
#7621=CIRCLE ( 'NONE', #706, 19.11328065563151668 ) ;
#7622=CARTESIAN_POINT ( 'NONE',  ( 14.93538271375424742, 34.13396246814581758, -7.000000000000006217 ) ) ;
#7623=CIRCLE ( 'NONE', #5807, 31.50000000000000711 ) ;
#7631=ORIENTED_EDGE ( 'NONE', *, *, #15790, .T. ) ;
#7634=EDGE_CURVE ( 'NONE', #7992, #2079, #10012, .T. ) ;
#7635=CARTESIAN_POINT ( 'NONE',  ( 15.62726112422616076, 28.45046755804886374, -2.999999999999971578 ) ) ;
#7639=AXIS2_PLACEMENT_3D ( 'NONE', #17540, #7005, #3236 ) ;
#7641=AXIS2_PLACEMENT_3D ( 'NONE', #18480, #18601, #9611 ) ;
#7642=CARTESIAN_POINT ( 'NONE',  ( -30.57187188083506157, -7.711478842616581453, -2.999999999999971578 ) ) ;
#7643=DIRECTION ( 'NONE',  ( 6.505213034913038160E-19, 3.903127820947822896E-18, 1.000000000000000000 ) ) ;
#7646=VERTEX_POINT ( 'NONE', #12533 ) ;
#7649=CARTESIAN_POINT ( 'NONE',  ( 1.110223024625156540E-13, -5.551115123125782702E-14, -6.999999999999950262 ) ) ;
#7651=AXIS2_PLACEMENT_3D ( 'NONE', #21236, #12404, #8966 ) ;
#7660=ORIENTED_EDGE ( 'NONE', *, *, #17157, .F. ) ;
#7661=CARTESIAN_POINT ( 'NONE',  ( 12.00937115242650677, 34.74700806321084912, -1.999999999999977573 ) ) ;
#7662=CARTESIAN_POINT ( 'NONE',  ( 4.025500340002707844, -36.54278193890314697, -2.800654218530457484 ) ) ;
#7665=ORIENTED_EDGE ( 'NONE', *, *, #17045, .T. ) ;
#7666=FACE_BOUND ( 'NONE', #9885, .T. ) ;
#7669=CARTESIAN_POINT ( 'NONE',  ( -37.07861450834822392, 3.656418565264024423, 2.999999999999995559 ) ) ;
#7672=DIRECTION ( 'NONE',  ( 6.505213034913038160E-19, 3.903127820947822896E-18, 1.000000000000000000 ) ) ;
#7673=CARTESIAN_POINT ( 'NONE',  ( -4.170748987303213084, 34.65667543218822999, -2.999999999999971578 ) ) ;
#7676=AXIS2_PLACEMENT_3D ( 'NONE', #4903, #18878, #8119 ) ;
#7677=CYLINDRICAL_SURFACE ( 'NONE', #3256, 1.000000000000000888 ) ;
#7679=FACE_OUTER_BOUND ( 'NONE', #14124, .T. ) ;
#7684=DIRECTION ( 'NONE',  ( 6.505213034913038160E-19, 3.903127820947822896E-18, 1.000000000000000000 ) ) ;
#7685=ORIENTED_EDGE ( 'NONE', *, *, #13301, .T. ) ;
#7690=ORIENTED_EDGE ( 'NONE', *, *, #12524, .T. ) ;
#7697=ORIENTED_EDGE ( 'NONE', *, *, #527, .F. ) ;
#7700=EDGE_CURVE ( 'NONE', #18105, #22110, #8098, .T. ) ;
#7702=DIRECTION ( 'NONE',  ( -6.505213034913038160E-19, -3.903127820947822896E-18, -1.000000000000000000 ) ) ;
#7703=CIRCLE ( 'NONE', #6242, 19.11328065563152379 ) ;
#7705=CARTESIAN_POINT ( 'NONE',  ( -31.92986134326219982, 18.22261011550282817, -2.800654218530485018 ) ) ;
#7708=DIRECTION ( 'NONE',  ( -6.505213034913038160E-19, -3.903127820947822896E-18, -1.000000000000000000 ) ) ;
#7710=ORIENTED_EDGE ( 'NONE', *, *, #10953, .F. ) ;
#7713=EDGE_CURVE ( 'NONE', #8041, #22419, #6247, .T. ) ;
#7717=LINE ( 'NONE', #2569, #12366 ) ;
#7720=DIRECTION ( 'NONE',  ( 1.000000000000000000, 0.000000000000000000, 0.000000000000000000 ) ) ;
#7724=CARTESIAN_POINT ( 'NONE',  ( -31.09841355225981374, 5.093313992686310243, -7.000000000000006217 ) ) ;
#7730=EDGE_LOOP ( 'NONE', ( #22023, #20304, #9905, #4329 ) ) ;
#7736=CARTESIAN_POINT ( 'NONE',  ( -15.02862401740788556, -32.75570538720795355, 3.000000000000002665 ) ) ;
#7738=DIRECTION ( 'NONE',  ( 1.000000000000000000, 0.000000000000000000, 0.000000000000000000 ) ) ;
#7739=DIRECTION ( 'NONE',  ( -6.505213034913038160E-19, -3.903127820947822896E-18, -1.000000000000000000 ) ) ;
#7742=ORIENTED_EDGE ( 'NONE', *, *, #13596, .T. ) ;
#7743=DIRECTION ( 'NONE',  ( -1.000000000000000000, -1.208970125616081209E-17, 0.000000000000000000 ) ) ;
#7744=CARTESIAN_POINT ( 'NONE',  ( 17.86915608785696818, -27.01645732367869002, -2.999999999999971578 ) ) ;
#7745=CARTESIAN_POINT ( 'NONE',  ( 29.33526866242100439, -22.15900668633777215, -2.800654218530429507 ) ) ;
#7746=DIRECTION ( 'NONE',  ( -6.505213034913038160E-19, -3.903127820947822896E-18, -1.000000000000000000 ) ) ;
#7747=CIRCLE ( 'NONE', #11393, 31.50000000000000000 ) ;
#7752=ORIENTED_EDGE ( 'NONE', *, *, #16173, .T. ) ;
#7753=EDGE_CURVE ( 'NONE', #13978, #7988, #2973, .T. ) ;
#7757=B_SPLINE_CURVE_WITH_KNOTS ( 'NONE', 3,
 ( #10792, #12188, #5321, #7033 ),
 .UNSPECIFIED., .F., .F.,
 ( 4, 4 ),
 ( 0.001875451646902607204, 0.003761979286331133213 ),
 .UNSPECIFIED. ) ;
#7762=DIRECTION ( 'NONE',  ( -6.505213034913038160E-19, -3.903127820947822896E-18, -1.000000000000000000 ) ) ;
#7765=CARTESIAN_POINT ( 'NONE',  ( -34.24928931925748543, 6.742883674876520850, -2.999999999999957367 ) ) ;
#7766=DIRECTION ( 'NONE',  ( 6.505213034913038160E-19, 3.903127820947822896E-18, 1.000000000000000000 ) ) ;
#7769=EDGE_LOOP ( 'NONE', ( #22136, #9696, #18929, #7665, #11529, #18252 ) ) ;
#7771=DIRECTION ( 'NONE',  ( 6.505213034913038160E-19, 3.903127820947822896E-18, 1.000000000000000000 ) ) ;
#7772=DIRECTION ( 'NONE',  ( -6.505213034913038160E-19, -3.903127820947822896E-18, -1.000000000000000000 ) ) ;
#7773=AXIS2_PLACEMENT_3D ( 'NONE', #20396, #20284, #4473 ) ;
#7774=AXIS2_PLACEMENT_3D ( 'NONE', #4762, #10003, #16995 ) ;
#7780=CARTESIAN_POINT ( 'NONE',  ( -17.38064605515553041, -30.98879172160219042, 3.000000000000063505 ) ) ;
#7782=ORIENTED_EDGE ( 'NONE', *, *, #16769, .T. ) ;
#7784=LINE ( 'NONE', #11449, #11713 ) ;
#7786=VERTEX_POINT ( 'NONE', #3607 ) ;
#7790=CARTESIAN_POINT ( 'NONE',  ( 3.330669073875469621E-13, -1.110223024625156540E-13, -2.999999999999971578 ) ) ;
#7791=AXIS2_PLACEMENT_3D ( 'NONE', #11417, #20367, #7994 ) ;
#7795=CARTESIAN_POINT ( 'NONE',  ( 24.62019382530528233, -4.341204441673129466, 3.000000000000023537 ) ) ;
#7797=ORIENTED_EDGE ( 'NONE', *, *, #11966, .T. ) ;
#7800=CARTESIAN_POINT ( 'NONE',  ( -33.47097213929426829, 11.93830856187182832, 3.000000000000058620 ) ) ;
#7807=AXIS2_PLACEMENT_3D ( 'NONE', #7923, #14883, #11583 ) ;
#7819=ORIENTED_EDGE ( 'NONE', *, *, #6487, .F. ) ;
#7824=ORIENTED_EDGE ( 'NONE', *, *, #20103, .F. ) ;
#7825=CARTESIAN_POINT ( 'NONE',  ( 36.14481870267517394, -0.8626474017862676424, 2.932969818539060469 ) ) ;
#7840=EDGE_LOOP ( 'NONE', ( #20556, #20387, #12528, #17656, #10909, #22302 ) ) ;
#7849=CARTESIAN_POINT ( 'NONE',  ( -14.14132741310364416, -16.85297774861788156, -2.999999999999988898 ) ) ;
#7852=ORIENTED_EDGE ( 'NONE', *, *, #5933, .F. ) ;
#7853=DIRECTION ( 'NONE',  ( 6.505213034913038160E-19, 3.903127820947822896E-18, 1.000000000000000000 ) ) ;
#7856=DIRECTION ( 'NONE',  ( -6.505213034913038160E-19, -3.903127820947822896E-18, -1.000000000000000000 ) ) ;
#7858=B_SPLINE_CURVE_WITH_KNOTS ( 'NONE', 3,
 ( #16554, #18382, #1307, #2701 ),
 .UNSPECIFIED., .F., .F.,
 ( 4, 4 ),
 ( 0.001893031756885266799, 0.003808480026563702565 ),
 .UNSPECIFIED. ) ;
#7859=EDGE_CURVE ( 'NONE', #3604, #11652, #11746, .T. ) ;
#7861=CIRCLE ( 'NONE', #541, 0.9999999999999974465 ) ;
#7863=DIRECTION ( 'NONE',  ( 6.505213034913038160E-19, 3.903127820947822896E-18, 1.000000000000000000 ) ) ;
#7866=EDGE_CURVE ( 'NONE', #19753, #18815, #16826, .T. ) ;
#7867=EDGE_LOOP ( 'NONE', ( #22555, #12606, #11017, #754 ) ) ;
#7868=VECTOR ( 'NONE', #18660, 1000.000000000000000 ) ;
#7876=CARTESIAN_POINT ( 'NONE',  ( 12.31876324338296236, 30.07487443287962137, -6.999999999999950262 ) ) ;
#7880=DIRECTION ( 'NONE',  ( 6.505213034913038160E-19, 3.903127820947822896E-18, 1.000000000000000000 ) ) ;
#7884=ORIENTED_EDGE ( 'NONE', *, *, #5380, .F. ) ;
#7885=DIRECTION ( 'NONE',  ( 6.505213034913038160E-19, 3.903127820947822896E-18, 1.000000000000000000 ) ) ;
#7886=DIRECTION ( 'NONE',  ( -6.505213034913038160E-19, -3.903127820947822896E-18, -1.000000000000000000 ) ) ;
#7887=CYLINDRICAL_SURFACE ( 'NONE', #17900, 3.000000000000002665 ) ;
#7890=LINE ( 'NONE', #20040, #18802 ) ;
#7891=ORIENTED_EDGE ( 'NONE', *, *, #20702, .F. ) ;
#7892=AXIS2_PLACEMENT_3D ( 'NONE', #7790, #4476, #16146 ) ;
#7893=ORIENTED_EDGE ( 'NONE', *, *, #11989, .T. ) ;
#7897=EDGE_CURVE ( 'NONE', #4746, #21718, #18009, .T. ) ;
#7899=ORIENTED_EDGE ( 'NONE', *, *, #3376, .T. ) ;
#7903=VECTOR ( 'NONE', #4541, 1000.000000000000000 ) ;
#7909=B_SPLINE_CURVE_WITH_KNOTS ( 'NONE', 3,
 ( #18928, #3576, #5397, #3237 ),
 .UNSPECIFIED., .F., .F.,
 ( 4, 4 ),
 ( 0.001875451646902839224, 0.003761979286331241200 ),
 .UNSPECIFIED. ) ;
#7915=CARTESIAN_POINT ( 'NONE',  ( 18.22261011550294185, 31.92986134326200443, 2.800654218530481465 ) ) ;
#7916=ORIENTED_EDGE ( 'NONE', *, *, #5726, .T. ) ;
#7918=CARTESIAN_POINT ( 'NONE',  ( 4.936596639065565562, 31.11077005834400566, -6.999999999999950262 ) ) ;
#7919=EDGE_CURVE ( 'NONE', #2308, #22537, #10627, .T. ) ;
#7923=CARTESIAN_POINT ( 'NONE',  ( 5.551115123125782702E-14, -1.387778780781445676E-13, -5.749999999999949374 ) ) ;
#7925=VECTOR ( 'NONE', #13498, 1000.000000000000000 ) ;
#7927=CIRCLE ( 'NONE', #20737, 2.999999999999999112 ) ;
#7928=ORIENTED_EDGE ( 'NONE', *, *, #18484, .F. ) ;
#7929=ADVANCED_FACE ( 'NONE', ( #5638 ), #14101, .F. ) ;
#7933=CARTESIAN_POINT ( 'NONE',  ( 2.220446049250313081E-13, -8.326672684688674053E-14, 2.800654218530498785 ) ) ;
#7956=CARTESIAN_POINT ( 'NONE',  ( -15.62726112422574332, -28.45046755804889216, 2.999999999999995559 ) ) ;
#7960=VECTOR ( 'NONE', #116, 1000.000000000000000 ) ;
#7961=CIRCLE ( 'NONE', #3199, 19.11328065563151668 ) ;
#7962=VERTEX_POINT ( 'NONE', #4388 ) ;
#7964=EDGE_CURVE ( 'NONE', #6859, #7992, #16500, .T. ) ;
#7966=ORIENTED_EDGE ( 'NONE', *, *, #5719, .F. ) ;
#7968=AXIS2_PLACEMENT_3D ( 'NONE', #4944, #13280, #8488 ) ;
#7970=ORIENTED_EDGE ( 'NONE', *, *, #5719, .T. ) ;
#7973=ORIENTED_EDGE ( 'NONE', *, *, #5785, .F. ) ;
#7974=DIRECTION ( 'NONE',  ( 6.505213034913038160E-19, 3.903127820947822896E-18, 1.000000000000000000 ) ) ;
#7984=CARTESIAN_POINT ( 'NONE',  ( -32.14641817400179491, -18.83615802559812735, 3.000000000000023537 ) ) ;
#7987=CIRCLE ( 'NONE', #12005, 0.9999999999999974465 ) ;
#7988=VERTEX_POINT ( 'NONE', #12955 ) ;
#7992=VERTEX_POINT ( 'NONE', #15120 ) ;
#7994=DIRECTION ( 'NONE',  ( -1.000000000000000000, -1.208970125616077665E-17, 0.000000000000000000 ) ) ;
#7998=CARTESIAN_POINT ( 'NONE',  ( 31.11359284679396353, 4.918774254215635189, 2.999999999999995559 ) ) ;
#7999=AXIS2_PLACEMENT_3D ( 'NONE', #6650, #6545, #845 ) ;
#8007=AXIS2_PLACEMENT_3D ( 'NONE', #2039, #19804, #21181 ) ;
#8008=ORIENTED_EDGE ( 'NONE', *, *, #13426, .T. ) ;
#8011=DIRECTION ( 'NONE',  ( -6.505213034913038160E-19, -3.903127820947822896E-18, -1.000000000000000000 ) ) ;
#8016=DIRECTION ( 'NONE',  ( -6.505213034913038160E-19, -3.903127820947822896E-18, -1.000000000000000000 ) ) ;
#8018=AXIS2_PLACEMENT_3D ( 'NONE', #12566, #10972, #19577 ) ;
#8029=VERTEX_POINT ( 'NONE', #13064 ) ;
#8030=CARTESIAN_POINT ( 'NONE',  ( 33.52953626616073279, 9.708269511265299911, -2.999999999999999112 ) ) ;
#8037=FACE_OUTER_BOUND ( 'NONE', #4641, .T. ) ;
#8038=DIRECTION ( 'NONE',  ( -6.505213034913038160E-19, -3.903127820947822896E-18, -1.000000000000000000 ) ) ;
#8040=EDGE_CURVE ( 'NONE', #15365, #18812, #20083, .T. ) ;
#8041=VERTEX_POINT ( 'NONE', #11703 ) ;
#8045=ADVANCED_FACE ( 'NONE', ( #20309, #2443 ), #2897, .T. ) ;
#8046=ORIENTED_EDGE ( 'NONE', *, *, #17374, .T. ) ;
#8049=CARTESIAN_POINT ( 'NONE',  ( 15.62726112422596714, 28.45046755804883531, -6.999999999999992006 ) ) ;
#8050=CARTESIAN_POINT ( 'NONE',  ( -36.75746821813285692, 0.6841746959066752343, -2.800654218530457484 ) ) ;
#8054=CARTESIAN_POINT ( 'NONE',  ( 7.980461308159908285, -36.39375341857525825, -6.999999999999950262 ) ) ;
#8055=ORIENTED_EDGE ( 'NONE', *, *, #16463, .F. ) ;
#8057=B_SPLINE_CURVE_WITH_KNOTS ( 'NONE', 3,
 ( #961, #19872, #2576, #21825 ),
 .UNSPECIFIED., .F., .F.,
 ( 4, 4 ),
 ( 9.715086409935858850E-07, 0.001929643240672463279 ),
 .UNSPECIFIED. ) ;
#8068=ORIENTED_EDGE ( 'NONE', *, *, #18691, .T. ) ;
#8069=UNCERTAINTY_MEASURE_WITH_UNIT (LENGTH_MEASURE( 1.000000000000000082E-05 ), #3672, 'distance_accuracy_value', 'NONE');
#8070=AXIS2_PLACEMENT_3D ( 'NONE', #75, #14028, #22680 ) ;
#8071=CARTESIAN_POINT ( 'NONE',  ( -27.95348479018568355, 14.76298474240492276, -2.999999999999999112 ) ) ;
#8075=EDGE_CURVE ( 'NONE', #20003, #16662, #20171, .T. ) ;
#8076=ORIENTED_EDGE ( 'NONE', *, *, #13195, .F. ) ;
#8080=EDGE_CURVE ( 'NONE', #14890, #15747, #18588, .T. ) ;
#8084=DIRECTION ( 'NONE',  ( -6.505213034913038160E-19, -3.903127820947822896E-18, -1.000000000000000000 ) ) ;
#8085=ORIENTED_EDGE ( 'NONE', *, *, #7077, .T. ) ;
#8086=CARTESIAN_POINT ( 'NONE',  ( 3.656418565264246467, 37.07861450834818129, -6.999999999999950262 ) ) ;
#8090=EDGE_CURVE ( 'NONE', #3379, #12610, #7356, .T. ) ;
#8092=ORIENTED_EDGE ( 'NONE', *, *, #9036, .F. ) ;
#8095=FACE_OUTER_BOUND ( 'NONE', #1974, .T. ) ;
#8098=CIRCLE ( 'NONE', #4802, 1.000000000000000888 ) ;
#8104=DIRECTION ( 'NONE',  ( 6.505213034913038160E-19, 3.903127820947822896E-18, 1.000000000000000000 ) ) ;
#8108=EDGE_CURVE ( 'NONE', #11717, #11286, #17076, .T. ) ;
#8110=ORIENTED_EDGE ( 'NONE', *, *, #10469, .T. ) ;
#8111=DIRECTION ( 'NONE',  ( 6.505213034913038160E-19, 3.903127820947822896E-18, 1.000000000000000000 ) ) ;
#8119=DIRECTION ( 'NONE',  ( 1.000000000000000000, 0.000000000000000000, 0.000000000000000000 ) ) ;
#8123=DIRECTION ( 'NONE',  ( 6.505213034913038160E-19, 3.903127820947822896E-18, 1.000000000000000000 ) ) ;
#8128=EDGE_CURVE ( 'NONE', #8181, #5732, #10602, .T. ) ;
#8129=AXIS2_PLACEMENT_3D ( 'NONE', #2420, #7684, #12933 ) ;
#8132=CARTESIAN_POINT ( 'NONE',  ( 21.65063509461090518, 12.49999999999978861, 2.999999999999995559 ) ) ;
#8137=LINE ( 'NONE', #15097, #9216 ) ;
#8142=CYLINDRICAL_SURFACE ( 'NONE', #21362, 1.000000000000000888 ) ;
#8143=ORIENTED_EDGE ( 'NONE', *, *, #11989, .F. ) ;
#8148=ORIENTED_EDGE ( 'NONE', *, *, #12598, .F. ) ;
#8152=EDGE_LOOP ( 'NONE', ( #14009, #2806, #19500, #1309, #16780 ) ) ;
#8157=DIRECTION ( 'NONE',  ( -6.505213034913038160E-19, -3.903127820947822896E-18, -1.000000000000000000 ) ) ;
#8161=ORIENTED_EDGE ( 'NONE', *, *, #17834, .F. ) ;
#8163=AXIS2_PLACEMENT_3D ( 'NONE', #962, #16542, #13421 ) ;
#8166=LINE ( 'NONE', #22151, #19604 ) ;
#8167=ORIENTED_EDGE ( 'NONE', *, *, #21962, .T. ) ;
#8168=LINE ( 'NONE', #2912, #18086 ) ;
#8176=DIRECTION ( 'NONE',  ( 6.505213034913038160E-19, 3.903127820947822896E-18, 1.000000000000000000 ) ) ;
#8181=VERTEX_POINT ( 'NONE', #8598 ) ;
#8182=VERTEX_POINT ( 'NONE', #8381 ) ;
#8183=VERTEX_POINT ( 'NONE', #19040 ) ;
#8184=ORIENTED_EDGE ( 'NONE', *, *, #1905, .T. ) ;
#8193=CIRCLE ( 'NONE', #21003, 19.11328065563151668 ) ;
#8194=EDGE_CURVE ( 'NONE', #20949, #2722, #5865, .T. ) ;
#8204=AXIS2_PLACEMENT_3D ( 'NONE', #5446, #10687, #19431 ) ;
#8206=ORIENTED_EDGE ( 'NONE', *, *, #19432, .F. ) ;
#8211=ORIENTED_EDGE ( 'NONE', *, *, #13900, .F. ) ;
#8216=EDGE_LOOP ( 'NONE', ( #19479, #4957, #15945, #5387 ) ) ;
#8218=CYLINDRICAL_SURFACE ( 'NONE', #2521, 36.76383501243555685 ) ;
#8223=ORIENTED_EDGE ( 'NONE', *, *, #11640, .F. ) ;
#8225=CARTESIAN_POINT ( 'NONE',  ( -27.95348479018550591, 14.76298474240492276, -6.999999999999950262 ) ) ;
#8226=EDGE_LOOP ( 'NONE', ( #7685, #13794, #19507, #11734 ) ) ;
#8229=LINE ( 'NONE', #8342, #11573 ) ;
#8230=ADVANCED_FACE ( 'NONE', ( #10417 ), #10, .F. ) ;
#8231=VERTEX_POINT ( 'NONE', #21093 ) ;
#8234=FACE_OUTER_BOUND ( 'NONE', #326, .T. ) ;
#8236=DIRECTION ( 'NONE',  ( -6.505213034913038160E-19, -3.903127820947822896E-18, -1.000000000000000000 ) ) ;
#8238=CARTESIAN_POINT ( 'NONE',  ( 17.66631876130941947, -31.41173278719250206, -6.999999999999950262 ) ) ;
#8240=DIRECTION ( 'NONE',  ( -6.505213034913038160E-19, -3.903127820947822896E-18, -1.000000000000000000 ) ) ;
#8241=CIRCLE ( 'NONE', #13701, 31.50000000000001421 ) ;
#8247=DIRECTION ( 'NONE',  ( -1.000000000000000000, 0.000000000000000000, 0.000000000000000000 ) ) ;
#8249=CARTESIAN_POINT ( 'NONE',  ( -34.65667543218827973, -4.170748987303380062, 3.000000000000002665 ) ) ;
#8252=LINE ( 'NONE', #20517, #4698 ) ;
#8253=CARTESIAN_POINT ( 'NONE',  ( -7.196011215416630691, -35.43002037646316182, -2.933296326616338767 ) ) ;
#8254=CARTESIAN_POINT ( 'NONE',  ( -28.95348479018568355, 14.76298474240497782, -2.999999999999999112 ) ) ;
#8257=ORIENTED_EDGE ( 'NONE', *, *, #19893, .F. ) ;
#8258=VECTOR ( 'NONE', #10124, 1000.000000000000000 ) ;
#8261=CIRCLE ( 'NONE', #2416, 36.76383501243555685 ) ;
#8263=DIRECTION ( 'NONE',  ( 6.505213034913038160E-19, 3.903127820947822896E-18, 1.000000000000000000 ) ) ;
#8266=CARTESIAN_POINT ( 'NONE',  ( 2.775557561562891351E-14, -2.775557561562891351E-14, 2.999999999999999112 ) ) ;
#8267=FACE_OUTER_BOUND ( 'NONE', #6768, .T. ) ;
#8270=DIRECTION ( 'NONE',  ( -1.000000000000000000, 6.171687555462485044E-15, 0.000000000000000000 ) ) ;
#8274=ADVANCED_FACE ( 'NONE', ( #3685 ), #571, .T. ) ;
#8278=ORIENTED_EDGE ( 'NONE', *, *, #5324, .F. ) ;
#8281=FACE_OUTER_BOUND ( 'NONE', #10213, .T. ) ;
#8282=VECTOR ( 'NONE', #17454, 1000.000000000000000 ) ;
#8295=ORIENTED_EDGE ( 'NONE', *, *, #17139, .T. ) ;
#8299=DIRECTION ( 'NONE',  ( 1.000000000000000000, 0.000000000000000000, 0.000000000000000000 ) ) ;
#8305=CARTESIAN_POINT ( 'NONE',  ( -22.28024240313483517, -22.26748298433275863, -6.999999999999957367 ) ) ;
#8307=VERTEX_POINT ( 'NONE', #12583 ) ;
#8314=CIRCLE ( 'NONE', #10864, 19.11328065563151668 ) ;
#8315=DIRECTION ( 'NONE',  ( -0.7071067811865522357, 8.080682403282904861E-17, 0.7071067811865429098 ) ) ;
#8322=CARTESIAN_POINT ( 'NONE',  ( 3.330669073875469621E-13, -1.110223024625156540E-13, -2.999999999999971578 ) ) ;
#8329=DIRECTION ( 'NONE',  ( -1.000000000000000000, -1.208970125616044077E-17, 0.000000000000000000 ) ) ;
#8330=ORIENTED_EDGE ( 'NONE', *, *, #7859, .T. ) ;
#8333=CARTESIAN_POINT ( 'NONE',  ( 3.330669073875469621E-13, -1.110223024625156540E-13, -2.999999999999971578 ) ) ;
#8334=EDGE_LOOP ( 'NONE', ( #17450, #2574, #3016, #1919 ) ) ;
#8341=AXIS2_PLACEMENT_3D ( 'NONE', #8333, #13575, #12108 ) ;
#8342=CARTESIAN_POINT ( 'NONE',  ( 31.41239365194212141, -2.347663744114298012, -6.999999999999999112 ) ) ;
#8349=AXIS2_PLACEMENT_3D ( 'NONE', #12801, #2395, #13359 ) ;
#8351=EDGE_CURVE ( 'NONE', #16045, #3371, #15343, .T. ) ;
#8352=ORIENTED_EDGE ( 'NONE', *, *, #4590, .F. ) ;
#8355=CYLINDRICAL_SURFACE ( 'NONE', #13540, 19.11328065563151668 ) ;
#8358=CARTESIAN_POINT ( 'NONE',  ( 10.01544929272322548, -34.09574698892478750, 3.000000000000064837 ) ) ;
#8361=EDGE_CURVE ( 'NONE', #1555, #15098, #12076, .T. ) ;
#8370=VECTOR ( 'NONE', #10880, 1000.000000000000000 ) ;
#8374=CIRCLE ( 'NONE', #17872, 0.9999999999999974465 ) ;
#8376=VERTEX_POINT ( 'NONE', #9163 ) ;
#8378=VERTEX_POINT ( 'NONE', #19724 ) ;
#8380=CARTESIAN_POINT ( 'NONE',  ( 36.39375341857553536, 7.980461308159658707, -2.999999999999981792 ) ) ;
#8381=CARTESIAN_POINT ( 'NONE',  ( 30.33632613426184932, -11.35354668330706929, -2.999999999999971578 ) ) ;
#8388=ORIENTED_EDGE ( 'NONE', *, *, #18322, .T. ) ;
#8389=CARTESIAN_POINT ( 'NONE',  ( 32.14641817400190860, 18.83615802559793195, 2.999999999999995559 ) ) ;
#8393=ORIENTED_EDGE ( 'NONE', *, *, #4213, .F. ) ;
#8398=VERTEX_POINT ( 'NONE', #9400 ) ;
#8400=EDGE_CURVE ( 'NONE', #16662, #22210, #4, .T. ) ;
#8409=ORIENTED_EDGE ( 'NONE', *, *, #3449, .F. ) ;
#8411=LINE ( 'NONE', #22400, #11848 ) ;
#8412=EDGE_CURVE ( 'NONE', #16827, #12526, #13887, .T. ) ;
#8413=AXIS2_PLACEMENT_3D ( 'NONE', #19483, #3787, #16032 ) ;
#8416=FACE_OUTER_BOUND ( 'NONE', #16962, .T. ) ;
#8421=VERTEX_POINT ( 'NONE', #801 ) ;
#8422=CYLINDRICAL_SURFACE ( 'NONE', #15932, 19.11328065563151668 ) ;
#8427=AXIS2_PLACEMENT_3D ( 'NONE', #1243, #17388, #6631 ) ;
#8428=DIRECTION ( 'NONE',  ( 6.505213034913038160E-19, 3.903127820947822896E-18, 1.000000000000000000 ) ) ;
#8432=ORIENTED_EDGE ( 'NONE', *, *, #13669, .F. ) ;
#8433=ORIENTED_EDGE ( 'NONE', *, *, #12806, .F. ) ;
#8436=EDGE_CURVE ( 'NONE', #12666, #13122, #18669, .T. ) ;
#8443=VERTEX_POINT ( 'NONE', #11217 ) ;
#8444=DIRECTION ( 'NONE',  ( 6.505213034913038160E-19, 3.903127820947822896E-18, 1.000000000000000000 ) ) ;
#8447=CARTESIAN_POINT ( 'NONE',  ( -27.64365646977275048, -17.09029715894938661, -6.999999999999950262 ) ) ;
#8448=EDGE_CURVE ( 'NONE', #8987, #11042, #7784, .T. ) ;
#8449=VERTEX_POINT ( 'NONE', #13254 ) ;
#8451=ORIENTED_EDGE ( 'NONE', *, *, #17139, .F. ) ;
#8452=CARTESIAN_POINT ( 'NONE',  ( -36.76383501243532947, -2.502446443229913594E-13, -6.859353255829918616 ) ) ;
#8457=ADVANCED_FACE ( 'NONE', ( #5953 ), #18436, .T. ) ;
#8460=ORIENTED_EDGE ( 'NONE', *, *, #21500, .F. ) ;
#8461=DIRECTION ( 'NONE',  ( -1.000000000000000000, 0.000000000000000000, 0.000000000000000000 ) ) ;
#8464=AXIS2_PLACEMENT_3D ( 'NONE', #3231, #22481, #8596 ) ;
#8470=EDGE_CURVE ( 'NONE', #17781, #14951, #14624, .T. ) ;
#8475=CARTESIAN_POINT ( 'NONE',  ( 35.91964150878187922, 4.104665049622501449, -2.933296326616344984 ) ) ;
#8477=DIRECTION ( 'NONE',  ( -1.000000000000000000, -9.002681209562840861E-16, 0.000000000000000000 ) ) ;
#8481=AXIS2_PLACEMENT_3D ( 'NONE', #8518, #6693, #13772 ) ;
#8485=CARTESIAN_POINT ( 'NONE',  ( 20.17230487860821597, 25.34312177887337825, -6.999999999999950262 ) ) ;
#8488=DIRECTION ( 'NONE',  ( 1.000000000000000000, 1.208970125616067650E-17, 0.000000000000000000 ) ) ;
#8495=DIRECTION ( 'NONE',  ( 6.505213034913038160E-19, 3.903127820947822896E-18, 1.000000000000000000 ) ) ;
#8502=ORIENTED_EDGE ( 'NONE', *, *, #5444, .T. ) ;
#8503=CARTESIAN_POINT ( 'NONE',  ( 5.551115123125782702E-14, -1.387778780781445676E-13, -5.749999999999949374 ) ) ;
#8510=ADVANCED_FACE ( 'NONE', ( #16839 ), #12814, .T. ) ;
#8514=ORIENTED_EDGE ( 'NONE', *, *, #5270, .F. ) ;
#8516=DIRECTION ( 'NONE',  ( -1.000000000000000000, 0.000000000000000000, 0.000000000000000000 ) ) ;
#8518=CARTESIAN_POINT ( 'NONE',  ( -3.656418565264246467, -37.07861450834820971, 2.999999999999995559 ) ) ;
#8523=CARTESIAN_POINT ( 'NONE',  ( 28.88846368933348074, 19.59430950039314823, 2.999999999999995559 ) ) ;
#8528=ORIENTED_EDGE ( 'NONE', *, *, #3197, .T. ) ;
#8529=CARTESIAN_POINT ( 'NONE',  ( -31.11077005834421527, 4.936596639065232495, -2.999999999999971578 ) ) ;
#8532=DIRECTION ( 'NONE',  ( 6.505213034913038160E-19, 3.903127820947822896E-18, 1.000000000000000000 ) ) ;
#8533=TOROIDAL_SURFACE ( 'NONE', #4881, 34.90673715956759082, 8.750000000000000000 ) ;
#8534=CARTESIAN_POINT ( 'NONE',  ( -31.88709182564695865, 6.070730550690822902, -7.000000000000006217 ) ) ;
#8536=EDGE_CURVE ( 'NONE', #8959, #12838, #9899, .T. ) ;
#8542=CARTESIAN_POINT ( 'NONE',  ( -4.025500340002485800, 36.54278193890309012, 2.800654218530485018 ) ) ;
#8543=CARTESIAN_POINT ( 'NONE',  ( -23.74488952252751162, 25.58633464742629471, -2.999999999999971578 ) ) ;
#8545=AXIS2_PLACEMENT_3D ( 'NONE', #17283, #13946, #15561 ) ;
#8553=CYLINDRICAL_SURFACE ( 'NONE', #6513, 31.50000000000001421 ) ;
#8556=ADVANCED_FACE ( 'NONE', ( #15324 ), #6525, .T. ) ;
#8559=CARTESIAN_POINT ( 'NONE',  ( 21.65063509461118230, 12.49999999999984368, -2.999999999999988898 ) ) ;
#8562=EDGE_LOOP ( 'NONE', ( #5520, #15057, #23, #1238, #20563, #17188 ) ) ;
#8563=ADVANCED_FACE ( 'NONE', ( #22345 ), #4703, .T. ) ;
#8564=VECTOR ( 'NONE', #16370, 1000.000000000000000 ) ;
#8566=DIRECTION ( 'NONE',  ( -1.000000000000000000, 0.000000000000000000, 0.000000000000000000 ) ) ;
#8569=ORIENTED_EDGE ( 'NONE', *, *, #2239, .F. ) ;
#8573=CARTESIAN_POINT ( 'NONE',  ( 16.99647590252675755, 30.48934413892762052, 3.000000000000019984 ) ) ;
#8580=AXIS2_PLACEMENT_3D ( 'NONE', #18825, #18938, #1521 ) ;
#8588=CARTESIAN_POINT ( 'NONE',  ( 3.330669073875469621E-13, -1.110223024625156540E-13, -2.999999999999971578 ) ) ;
#8589=CIRCLE ( 'NONE', #21034, 1.000000000000000888 ) ;
#8590=ORIENTED_EDGE ( 'NONE', *, *, #15224, .T. ) ;
#8591=ADVANCED_FACE ( 'NONE', ( #10390 ), #8355, .T. ) ;
#8593=CIRCLE ( 'NONE', #22161, 19.11328065563152379 ) ;
#8596=DIRECTION ( 'NONE',  ( -1.000000000000000000, -1.208970125616014957E-17, 0.000000000000000000 ) ) ;
#8597=CIRCLE ( 'NONE', #3505, 1.000000000000000888 ) ;
#8598=CARTESIAN_POINT ( 'NONE',  ( -24.03323817228468329, 20.36304159388335933, 3.000000000000009770 ) ) ;
#8600=CARTESIAN_POINT ( 'NONE',  ( 3.330669073875469621E-13, -1.110223024625156540E-13, -2.999999999999971578 ) ) ;
#8610=CARTESIAN_POINT ( 'NONE',  ( -25.34312177887333561, 20.17230487860788202, -6.999999999999950262 ) ) ;
#8611=DIRECTION ( 'NONE',  ( 6.505213034913038160E-19, 3.903127820947822896E-18, 1.000000000000000000 ) ) ;
#8620=VECTOR ( 'NONE', #11971, 1000.000000000000000 ) ;
#8626=EDGE_LOOP ( 'NONE', ( #8393, #7139, #19765, #5800 ) ) ;
#8627=ADVANCED_FACE ( 'NONE', ( #10727 ), #3695, .T. ) ;
#8635=CARTESIAN_POINT ( 'NONE',  ( -19.59430950039320152, 28.88846368933331732, -2.999999999999999112 ) ) ;
#8637=ORIENTED_EDGE ( 'NONE', *, *, #11796, .F. ) ;
#8642=EDGE_LOOP ( 'NONE', ( #11859, #5521, #10153, #1857 ) ) ;
#8643=CARTESIAN_POINT ( 'NONE',  ( -19.99999999999999289, -2.799736964075212609E-14, 2.999999999999995559 ) ) ;
#8644=ORIENTED_EDGE ( 'NONE', *, *, #15453, .T. ) ;
#8648=CIRCLE ( 'NONE', #21450, 19.11328065563152379 ) ;
#8649=ADVANCED_FACE ( 'NONE', ( #8807 ), #1475, .T. ) ;
#8655=AXIS2_PLACEMENT_3D ( 'NONE', #12274, #19280, #238 ) ;
#8657=ORIENTED_EDGE ( 'NONE', *, *, #2335, .T. ) ;
#8660=CARTESIAN_POINT ( 'NONE',  ( 2.775557561562891351E-14, -2.775557561562891351E-14, 2.999999999999999112 ) ) ;
#8664=DIRECTION ( 'NONE',  ( -1.000000000000000000, 0.000000000000000000, 0.000000000000000000 ) ) ;
#8670=CARTESIAN_POINT ( 'NONE',  ( 3.330669073875469621E-13, -1.110223024625156540E-13, -2.999999999999971578 ) ) ;
#8674=ORIENTED_EDGE ( 'NONE', *, *, #8927, .T. ) ;
#8678=ADVANCED_FACE ( 'NONE', ( #22694 ), #10848, .T. ) ;
#8682=AXIS2_PLACEMENT_3D ( 'NONE', #8830, #19044, #13962 ) ;
#8686=VERTEX_POINT ( 'NONE', #1926 ) ;
#8687=CARTESIAN_POINT ( 'NONE',  ( -7.463862311150981199, -35.99819890246952525, 2.800654218530485018 ) ) ;
#8690=ADVANCED_FACE ( 'NONE', ( #12234 ), #3322, .T. ) ;
#8691=DIRECTION ( 'NONE',  ( 1.000000000000000000, 0.000000000000000000, 0.000000000000000000 ) ) ;
#8692=AXIS2_PLACEMENT_3D ( 'NONE', #6791, #12061, #11945 ) ;
#8695=CARTESIAN_POINT ( 'NONE',  ( -27.01645732367843777, -17.86915608785696818, -6.999999999999950262 ) ) ;
#8697=CARTESIAN_POINT ( 'NONE',  ( -30.07487443287963558, 12.31876324338265860, -6.999999999999950262 ) ) ;
#8699=ORIENTED_EDGE ( 'NONE', *, *, #17157, .T. ) ;
#8703=CARTESIAN_POINT ( 'NONE',  ( 36.54278193890314697, 4.025500340002402311, -2.800654218530457484 ) ) ;
#8704=AXIS2_PLACEMENT_3D ( 'NONE', #3997, #12789, #19801 ) ;
#8707=CARTESIAN_POINT ( 'NONE',  ( 14.93538271375424742, 34.13396246814559731, -2.999999999999999112 ) ) ;
#8708=CIRCLE ( 'NONE', #22271, 1.000000000000000888 ) ;
#8709=EDGE_CURVE ( 'NONE', #12493, #18822, #11728, .T. ) ;
#8710=ORIENTED_EDGE ( 'NONE', *, *, #21309, .F. ) ;
#8714=AXIS2_PLACEMENT_3D ( 'NONE', #8785, #20932, #5345 ) ;
#8716=FACE_OUTER_BOUND ( 'NONE', #3917, .T. ) ;
#8717=EDGE_CURVE ( 'NONE', #4617, #3722, #7703, .T. ) ;
#8729=CARTESIAN_POINT ( 'NONE',  ( 2.220446049250313081E-13, -8.326672684688674053E-14, 2.800654218530498785 ) ) ;
#8730=CARTESIAN_POINT ( 'NONE',  ( 3.330669073875469621E-13, -1.110223024625156540E-13, -2.999999999999971578 ) ) ;
#8732=ORIENTED_EDGE ( 'NONE', *, *, #20815, .F. ) ;
#8736=AXIS2_PLACEMENT_3D ( 'NONE', #3852, #3974, #7738 ) ;
#8739=AXIS2_PLACEMENT_3D ( 'NONE', #2843, #4216, #9828 ) ;
#8740=EDGE_CURVE ( 'NONE', #2277, #2772, #11354, .T. ) ;
#8743=VECTOR ( 'NONE', #345, 1000.000000000000000 ) ;
#8746=EDGE_CURVE ( 'NONE', #3679, #14442, #15046, .T. ) ;
#8748=ORIENTED_EDGE ( 'NONE', *, *, #8361, .T. ) ;
#8750=EDGE_LOOP ( 'NONE', ( #953, #21327, #8799, #7473 ) ) ;
#8757=CARTESIAN_POINT ( 'NONE',  ( 29.33203831401607786, 20.06142356895397327, 3.000000000000044853 ) ) ;
#8765=CARTESIAN_POINT ( 'NONE',  ( 2.775557561562891351E-14, -2.775557561562891351E-14, 2.999999999999999112 ) ) ;
#8768=ADVANCED_FACE ( 'NONE', ( #11846 ), #7536, .F. ) ;
#8770=B_SPLINE_CURVE_WITH_KNOTS ( 'NONE', 3,
 ( #3110, #17413, #15576, #20635 ),
 .UNSPECIFIED., .F., .F.,
 ( 4, 4 ),
 ( 0.001893031756885503371, 0.003808480026563726851 ),
 .UNSPECIFIED. ) ;
#8775=EDGE_CURVE ( 'NONE', #18499, #5723, #13321, .T. ) ;
#8776=ORIENTED_EDGE ( 'NONE', *, *, #7634, .T. ) ;
#8778=ORIENTED_EDGE ( 'NONE', *, *, #2942, .T. ) ;
#8781=CARTESIAN_POINT ( 'NONE',  ( 3.330669073875469621E-13, -1.110223024625156540E-13, -2.999999999999971578 ) ) ;
#8782=DIRECTION ( 'NONE',  ( 0.7071067811865522357, 1.130863789078081945E-17, 0.7071067811865429098 ) ) ;
#8783=VECTOR ( 'NONE', #5916, 1000.000000000000000 ) ;
#8785=CARTESIAN_POINT ( 'NONE',  ( -3.656418565263996889, -37.07861450834837314, -6.999999999999950262 ) ) ;
#8788=DIRECTION ( 'NONE',  ( 6.505213034913038160E-19, 3.903127820947822896E-18, 1.000000000000000000 ) ) ;
#8791=DIRECTION ( 'NONE',  ( -1.000000000000000000, -1.208970125616060717E-17, 0.000000000000000000 ) ) ;
#8793=AXIS2_PLACEMENT_3D ( 'NONE', #4472, #912, #9514 ) ;
#8797=DIRECTION ( 'NONE',  ( 6.505213034913038160E-19, 3.903127820947822896E-18, 1.000000000000000000 ) ) ;
#8799=ORIENTED_EDGE ( 'NONE', *, *, #18807, .F. ) ;
#8800=EDGE_LOOP ( 'NONE', ( #22332, #21258, #3709, #18619 ) ) ;
#8806=VERTEX_POINT ( 'NONE', #6474 ) ;
#8807=FACE_OUTER_BOUND ( 'NONE', #11019, .T. ) ;
#8808=EDGE_CURVE ( 'NONE', #12800, #2882, #18386, .T. ) ;
#8810=DIRECTION ( 'NONE',  ( -1.000000000000000000, 0.000000000000000000, 0.000000000000000000 ) ) ;
#8814=CARTESIAN_POINT ( 'NONE',  ( -21.65063509461084834, 12.49999999999965006, 3.000000000000023537 ) ) ;
#8820=DIRECTION ( 'NONE',  ( 6.505213034913038160E-19, 3.903127820947822896E-18, 1.000000000000000000 ) ) ;
#8821=EDGE_CURVE ( 'NONE', #6187, #20709, #5508, .T. ) ;
#8830=CARTESIAN_POINT ( 'NONE',  ( 32.14641817400218571, 18.83615802559782182, -2.999999999999992450 ) ) ;
#8831=EDGE_LOOP ( 'NONE', ( #10521, #14695, #21511, #2394, #11818, #22479 ) ) ;
#8839=EDGE_CURVE ( 'NONE', #767, #13978, #1311, .T. ) ;
#8846=EDGE_CURVE ( 'NONE', #295, #20003, #15377, .T. ) ;
#8849=VERTEX_POINT ( 'NONE', #10573 ) ;
#8851=B_SPLINE_CURVE_WITH_KNOTS ( 'NONE', 3,
 ( #17287, #8253, #4719, #13269 ),
 .UNSPECIFIED., .F., .F.,
 ( 4, 4 ),
 ( 9.545285769181932779E-07, 0.001900595205834454448 ),
 .UNSPECIFIED. ) ;
#8858=EDGE_LOOP ( 'NONE', ( #12468, #14583, #7108, #5788 ) ) ;
#8862=CYLINDRICAL_SURFACE ( 'NONE', #589, 19.11328065563151313 ) ;
#8863=DIRECTION ( 'NONE',  ( 6.505213034913038160E-19, 3.903127820947822896E-18, 1.000000000000000000 ) ) ;
#8865=CARTESIAN_POINT ( 'NONE',  ( 14.29266125237937857, -28.07080038625103668, -6.999999999999999112 ) ) ;
#8867=CARTESIAN_POINT ( 'NONE',  ( 34.84717828836195253, -6.955395936296957515, -2.999999999999999556 ) ) ;
#8873=DIRECTION ( 'NONE',  ( -1.000000000000000000, -7.260808888779397243E-16, 0.000000000000000000 ) ) ;
#8874=CIRCLE ( 'NONE', #13980, 19.11328065563152379 ) ;
#8890=EDGE_CURVE ( 'NONE', #11380, #19753, #16853, .T. ) ;
#8893=CARTESIAN_POINT ( 'NONE',  ( -34.11307262910428761, 11.98990878915333091, -2.932164912090547748 ) ) ;
#8894=VECTOR ( 'NONE', #12519, 1000.000000000000000 ) ;
#8897=CARTESIAN_POINT ( 'NONE',  ( -24.43568323314231350, 26.65040777864162536, 2.932460736555809966 ) ) ;
#8898=EDGE_CURVE ( 'NONE', #22152, #18617, #16729, .T. ) ;
#8899=ORIENTED_EDGE ( 'NONE', *, *, #11274, .T. ) ;
#8900=CIRCLE ( 'NONE', #7791, 36.76383501243555685 ) ;
#8901=ORIENTED_EDGE ( 'NONE', *, *, #11138, .T. ) ;
#8908=CARTESIAN_POINT ( 'NONE',  ( 2.775557561562891351E-14, 2.775557561562891351E-14, 5.750000000000001776 ) ) ;
#8910=CARTESIAN_POINT ( 'NONE',  ( 22.15900668633799597, 29.33526866242080899, -2.800654218530477912 ) ) ;
#8911=DIRECTION ( 'NONE',  ( 1.000000000000000000, 1.208970125616053321E-17, 0.000000000000000000 ) ) ;
#8913=DIRECTION ( 'NONE',  ( -1.000000000000000000, 0.000000000000000000, 0.000000000000000000 ) ) ;
#8916=CARTESIAN_POINT ( 'NONE',  ( 2.220446049250313081E-13, -2.498001805406602216E-13, -6.859353255829918616 ) ) ;
#8918=VECTOR ( 'NONE', #9500, 1000.000000000000000 ) ;
#8922=EDGE_CURVE ( 'NONE', #17550, #1088, #19543, .T. ) ;
#8923=ORIENTED_EDGE ( 'NONE', *, *, #19973, .F. ) ;
#8924=EDGE_CURVE ( 'NONE', #9113, #8307, #11140, .T. ) ;
#8925=LINE ( 'NONE', #12361, #11184 ) ;
#8927=EDGE_CURVE ( 'NONE', #15891, #16318, #16537, .T. ) ;
#8930=VECTOR ( 'NONE', #5365, 1000.000000000000000 ) ;
#8935=DIRECTION ( 'NONE',  ( 1.000000000000000000, 0.000000000000000000, 0.000000000000000000 ) ) ;
#8936=VERTEX_POINT ( 'NONE', #14224 ) ;
#8944=ORIENTED_EDGE ( 'NONE', *, *, #12017, .T. ) ;
#8946=AXIS2_PLACEMENT_3D ( 'NONE', #20595, #20491, #17263 ) ;
#8947=CARTESIAN_POINT ( 'NONE',  ( -16.06969024216325792, -19.15111107797470780, -4.999999999999969802 ) ) ;
#8951=CARTESIAN_POINT ( 'NONE',  ( -8.550503583141495056, 23.49231551964756193, 3.000000000000023537 ) ) ;
#8953=AXIS2_PLACEMENT_3D ( 'NONE', #5118, #16928, #9936 ) ;
#8954=ORIENTED_EDGE ( 'NONE', *, *, #16549, .T. ) ;
#8958=EDGE_CURVE ( 'NONE', #4779, #1795, #5531, .T. ) ;
#8959=VERTEX_POINT ( 'NONE', #10913 ) ;
#8960=CYLINDRICAL_SURFACE ( 'NONE', #18357, 0.9999999999999974465 ) ;
#8966=DIRECTION ( 'NONE',  ( -1.000000000000000000, 0.000000000000000000, 0.000000000000000000 ) ) ;
#8975=EDGE_LOOP ( 'NONE', ( #237, #15390, #14809, #19481 ) ) ;
#8977=AXIS2_PLACEMENT_3D ( 'NONE', #10769, #19170, #14086 ) ;
#8984=AXIS2_PLACEMENT_3D ( 'NONE', #3469, #22382, #13629 ) ;
#8985=AXIS2_PLACEMENT_3D ( 'NONE', #3861, #17604, #8791 ) ;
#8987=VERTEX_POINT ( 'NONE', #2099 ) ;
#8992=TOROIDAL_SURFACE ( 'NONE', #15568, 34.90673715956759082, 8.750000000000000000 ) ;
#8993=ORIENTED_EDGE ( 'NONE', *, *, #1183, .T. ) ;
#8994=CARTESIAN_POINT ( 'NONE',  ( 4.170748987303491084, -34.65667543218836499, -2.999999999999988898 ) ) ;
#8998=FACE_OUTER_BOUND ( 'NONE', #11134, .T. ) ;
#9004=DIRECTION ( 'NONE',  ( -6.505213034913038160E-19, -3.903127820947822896E-18, -1.000000000000000000 ) ) ;
#9010=AXIS2_PLACEMENT_3D ( 'NONE', #4448, #16578, #885 ) ;
#9011=AXIS2_PLACEMENT_3D ( 'NONE', #13415, #20546, #13296 ) ;
#9012=CONICAL_SURFACE ( 'NONE', #21841, 18.00000000000000000, 0.7853981633974540522 ) ;
#9016=ORIENTED_EDGE ( 'NONE', *, *, #11783, .F. ) ;
#9017=AXIS2_PLACEMENT_3D ( 'NONE', #13824, #22443, #20841 ) ;
#9018=ORIENTED_EDGE ( 'NONE', *, *, #15267, .F. ) ;
#9019=ADVANCED_FACE ( 'NONE', ( #7596 ), #6492, .T. ) ;
#9022=CARTESIAN_POINT ( 'NONE',  ( -32.89319786336240270, -15.00354810072223977, -2.933296326616348093 ) ) ;
#9024=DIRECTION ( 'NONE',  ( 6.505213034913038160E-19, 3.903127820947822896E-18, 1.000000000000000000 ) ) ;
#9026=EDGE_CURVE ( 'NONE', #8041, #16345, #16366, .T. ) ;
#9031=AXIS2_PLACEMENT_3D ( 'NONE', #5296, #14515, #14395 ) ;
#9033=CARTESIAN_POINT ( 'NONE',  ( -18.22261011550280330, -31.92986134326242365, -2.000000000000005329 ) ) ;
#9035=( NAMED_UNIT ( * ) PLANE_ANGLE_UNIT ( ) SI_UNIT ( $, .RADIAN. ) );
#9036=EDGE_CURVE ( 'NONE', #22537, #13925, #13790, .T. ) ;
#9037=DIRECTION ( 'NONE',  ( 6.505213034913038160E-19, 3.903127820947822896E-18, 1.000000000000000000 ) ) ;
#9042=AXIS2_PLACEMENT_3D ( 'NONE', #16972, #6222, #1068 ) ;
#9050=EDGE_CURVE ( 'NONE', #12342, #3379, #7205, .T. ) ;
#9051=ORIENTED_EDGE ( 'NONE', *, *, #18428, .T. ) ;
#9053=CIRCLE ( 'NONE', #2855, 1.000000000000000888 ) ;
#9058=EDGE_CURVE ( 'NONE', #22614, #21019, #13424, .T. ) ;
#9059=ORIENTED_EDGE ( 'NONE', *, *, #20824, .F. ) ;
#9069=DIRECTION ( 'NONE',  ( 6.505213034913038160E-19, 3.903127820947822896E-18, 1.000000000000000000 ) ) ;
#9075=CARTESIAN_POINT ( 'NONE',  ( 27.19760187735878532, 24.73600648735102681, -2.800654218530485018 ) ) ;
#9078=AXIS2_PLACEMENT_3D ( 'NONE', #1060, #6217, #21687 ) ;
#9079=ORIENTED_EDGE ( 'NONE', *, *, #3000, .F. ) ;
#9087=FACE_OUTER_BOUND ( 'NONE', #657, .T. ) ;
#9089=ORIENTED_EDGE ( 'NONE', *, *, #8924, .T. ) ;
#9091=CARTESIAN_POINT ( 'NONE',  ( -28.96193690644914653, -14.74639653023232455, -6.999999999999950262 ) ) ;
#9092=ORIENTED_EDGE ( 'NONE', *, *, #3448, .T. ) ;
#9098=ORIENTED_EDGE ( 'NONE', *, *, #16254, .F. ) ;
#9099=CARTESIAN_POINT ( 'NONE',  ( 2.220446049250313081E-13, -8.326672684688674053E-14, 2.800654218530498785 ) ) ;
#9100=EDGE_CURVE ( 'NONE', #691, #1737, #19314, .T. ) ;
#9105=ORIENTED_EDGE ( 'NONE', *, *, #20235, .T. ) ;
#9113=VERTEX_POINT ( 'NONE', #1169 ) ;
#9116=ORIENTED_EDGE ( 'NONE', *, *, #7713, .F. ) ;
#9132=LINE ( 'NONE', #19681, #5729 ) ;
#9133=ORIENTED_EDGE ( 'NONE', *, *, #15477, .T. ) ;
#9135=ORIENTED_EDGE ( 'NONE', *, *, #8846, .T. ) ;
#9136=VECTOR ( 'NONE', #21473, 1000.000000000000000 ) ;
#9138=ORIENTED_EDGE ( 'NONE', *, *, #19693, .F. ) ;
#9142=CARTESIAN_POINT ( 'NONE',  ( 20.55056392469605342, -29.75120097320042944, -2.932164912090510889 ) ) ;
#9147=CARTESIAN_POINT ( 'NONE',  ( -10.35112103033871556, 34.64554704988846368, -2.932164912090562847 ) ) ;
#9148=CIRCLE ( 'NONE', #19766, 36.76383501243555685 ) ;
#9150=LINE ( 'NONE', #19703, #6861 ) ;
#9154=CARTESIAN_POINT ( 'NONE',  ( 4.170748987303435129, -34.65667543218869895, 2.999999999999999112 ) ) ;
#9156=CARTESIAN_POINT ( 'NONE',  ( -21.00948735876882623, -24.79619811426206510, -6.999999999999950262 ) ) ;
#9158=AXIS2_PLACEMENT_3D ( 'NONE', #20566, #980, #21961 ) ;
#9163=CARTESIAN_POINT ( 'NONE',  ( 26.79308242454903066, 16.56444186175090749, -2.999999999999971578 ) ) ;
#9164=EDGE_CURVE ( 'NONE', #11367, #31, #17184, .T. ) ;
#9165=CARTESIAN_POINT ( 'NONE',  ( 11.98990878915362757, 34.11307262910417393, -2.932164912090556186 ) ) ;
#9167=DIRECTION ( 'NONE',  ( -6.505213034913038160E-19, -3.903127820947822896E-18, -1.000000000000000000 ) ) ;
#9169=ORIENTED_EDGE ( 'NONE', *, *, #9545, .F. ) ;
#9171=CARTESIAN_POINT ( 'NONE',  ( -27.56232195404058416, 21.41958700883256483, -2.999999999999971578 ) ) ;
#9174=LINE ( 'NONE', #7455, #18453 ) ;
#9175=ORIENTED_EDGE ( 'NONE', *, *, #6074, .F. ) ;
#9176=CARTESIAN_POINT ( 'NONE',  ( 1.128083539116558898, 34.88850421923955736, 3.000000000000002665 ) ) ;
#9177=CYLINDRICAL_SURFACE ( 'NONE', #1612, 36.76383501243555685 ) ;
#9181=EDGE_CURVE ( 'NONE', #18812, #21534, #22223, .T. ) ;
#9183=CARTESIAN_POINT ( 'NONE',  ( -36.39375341857525825, -7.980461308159936706, -2.999999999999971578 ) ) ;
#9184=DIRECTION ( 'NONE',  ( -1.000000000000000000, 0.000000000000000000, 0.000000000000000000 ) ) ;
#9186=ORIENTED_EDGE ( 'NONE', *, *, #16859, .T. ) ;
#9188=ORIENTED_EDGE ( 'NONE', *, *, #13504, .F. ) ;
#9197=VERTEX_POINT ( 'NONE', #10206 ) ;
#9198=CARTESIAN_POINT ( 'NONE',  ( 1.128083539116392364, 34.88850421923958578, -2.999999999999981792 ) ) ;
#9199=CARTESIAN_POINT ( 'NONE',  ( -11.31876324338254847, -30.07487443287981677, -6.999999999999950262 ) ) ;
#9208=EDGE_LOOP ( 'NONE', ( #13993, #17164, #12395, #19180, #12783, #18344 ) ) ;
#9215=ORIENTED_EDGE ( 'NONE', *, *, #7504, .F. ) ;
#9216=VECTOR ( 'NONE', #22120, 1000.000000000000000 ) ;
#9225=CYLINDRICAL_SURFACE ( 'NONE', #3630, 19.11328065563152379 ) ;
#9228=DIRECTION ( 'NONE',  ( -1.000000000000000000, -1.208970125616060717E-17, 0.000000000000000000 ) ) ;
#9240=CIRCLE ( 'NONE', #22071, 36.76383501243555685 ) ;
#9242=TOROIDAL_SURFACE ( 'NONE', #22072, 34.90673715956759082, 8.750000000000000000 ) ;
#9245=EDGE_CURVE ( 'NONE', #17600, #3953, #5384, .T. ) ;
#9256=DIRECTION ( 'NONE',  ( 6.505213034913038160E-19, 3.903127820947822896E-18, 1.000000000000000000 ) ) ;
#9261=ORIENTED_EDGE ( 'NONE', *, *, #18625, .T. ) ;
#9262=DIRECTION ( 'NONE',  ( 4.718764931986839378E-35, -3.903127820947822896E-18, -1.000000000000000000 ) ) ;
#9265=CARTESIAN_POINT ( 'NONE',  ( 2.775557561562891351E-14, -2.775557561562891351E-14, 2.999999999999999112 ) ) ;
#9266=CARTESIAN_POINT ( 'NONE',  ( -19.59430950039299546, 28.88846368933323205, 2.999999999999995559 ) ) ;
#9270=EDGE_CURVE ( 'NONE', #7486, #18033, #3118, .T. ) ;
#9272=CARTESIAN_POINT ( 'NONE',  ( -34.88850421923971368, 1.128083539116031542, -2.999999999999981792 ) ) ;
#9273=AXIS2_PLACEMENT_3D ( 'NONE', #16447, #19885, #756 ) ;
#9285=VERTEX_POINT ( 'NONE', #17646 ) ;
#9286=CARTESIAN_POINT ( 'NONE',  ( -21.41958700883256483, -27.56232195404059837, 2.999999999999995559 ) ) ;
#9287=CARTESIAN_POINT ( 'NONE',  ( -13.74639653023227481, 28.96193690644924246, 2.999999999999995559 ) ) ;
#9288=AXIS2_PLACEMENT_3D ( 'NONE', #4603, #9633, #14777 ) ;
#9289=DIRECTION ( 'NONE',  ( 1.000000000000000000, 1.208970125616063182E-17, 0.000000000000000000 ) ) ;
#9298=VECTOR ( 'NONE', #16107, 1000.000000000000000 ) ;
#9301=VECTOR ( 'NONE', #17978, 1000.000000000000000 ) ;
#9302=EDGE_CURVE ( 'NONE', #16523, #13978, #15984, .T. ) ;
#9313=DIRECTION ( 'NONE',  ( -1.000000000000000000, -1.208970125616077665E-17, 0.000000000000000000 ) ) ;
#9316=DIRECTION ( 'NONE',  ( -1.000000000000000000, -1.208970125616060717E-17, 0.000000000000000000 ) ) ;
#9317=CARTESIAN_POINT ( 'NONE',  ( -31.92986134326219982, 18.22261011550282817, -2.800654218530485018 ) ) ;
#9321=CARTESIAN_POINT ( 'NONE',  ( 35.28654656445771565, 4.153516728483715781, 3.000000000000051958 ) ) ;
#9322=ORIENTED_EDGE ( 'NONE', *, *, #12062, .T. ) ;
#9324=ORIENTED_EDGE ( 'NONE', *, *, #2741, .F. ) ;
#9326=EDGE_CURVE ( 'NONE', #5303, #3679, #2087, .T. ) ;
#9327=VECTOR ( 'NONE', #2109, 1000.000000000000000 ) ;
#9329=VERTEX_POINT ( 'NONE', #9287 ) ;
#9330=FACE_OUTER_BOUND ( 'NONE', #12874, .T. ) ;
#9332=CARTESIAN_POINT ( 'NONE',  ( 2.775557561562891351E-14, -2.775557561562891351E-14, 2.999999999999999112 ) ) ;
#9333=EDGE_CURVE ( 'NONE', #13252, #16345, #10881, .T. ) ;
#9334=CARTESIAN_POINT ( 'NONE',  ( 2.220446049250313081E-13, 2.775557561562891351E-14, -2.800654218530485018 ) ) ;
#9336=EDGE_CURVE ( 'NONE', #21534, #2308, #3956, .T. ) ;
#9339=AXIS2_PLACEMENT_3D ( 'NONE', #7669, #11091, #21536 ) ;
#9345=CARTESIAN_POINT ( 'NONE',  ( -15.12081897056664914, 33.51030287062364721, -2.800654218530457484 ) ) ;
#9347=CARTESIAN_POINT ( 'NONE',  ( -11.31876324338268880, -30.07487443287981677, 2.999999999999995559 ) ) ;
#9351=CIRCLE ( 'NONE', #20697, 19.11328065563151668 ) ;
#9352=ORIENTED_EDGE ( 'NONE', *, *, #8448, .F. ) ;
#9356=AXIS2_PLACEMENT_3D ( 'NONE', #22267, #15247, #4508 ) ;
#9359=CARTESIAN_POINT ( 'NONE',  ( -34.90673715956725687, 2.728857438001962765E-14, -2.999999999999971578 ) ) ;
#9362=AXIS2_PLACEMENT_3D ( 'NONE', #3979, #8788, #7058 ) ;
#9363=EDGE_LOOP ( 'NONE', ( #6049, #4274, #9352, #7388 ) ) ;
#9365=B_SPLINE_CURVE_WITH_KNOTS ( 'NONE', 3,
 ( #19598, #228, #9165, #12373 ),
 .UNSPECIFIED., .F., .F.,
 ( 4, 4 ),
 ( 0.001893031756885165751, 0.003808480026563545139 ),
 .UNSPECIFIED. ) ;
#9366=ORIENTED_EDGE ( 'NONE', *, *, #8839, .F. ) ;
#9372=EDGE_CURVE ( 'NONE', #1931, #8987, #7370, .T. ) ;
#9375=CIRCLE ( 'NONE', #20713, 36.76383501243555685 ) ;
#9376=CIRCLE ( 'NONE', #217, 1.000000000000000888 ) ;
#9381=CARTESIAN_POINT ( 'NONE',  ( -17.09029715894910950, 27.64365646977276469, -2.999999999999971578 ) ) ;
#9382=CIRCLE ( 'NONE', #15209, 34.90673715956759082 ) ;
#9383=ORIENTED_EDGE ( 'NONE', *, *, #22203, .F. ) ;
#9386=FACE_OUTER_BOUND ( 'NONE', #16952, .T. ) ;
#9398=ORIENTED_EDGE ( 'NONE', *, *, #12598, .T. ) ;
#9400=CARTESIAN_POINT ( 'NONE',  ( -20.00948735876881202, -24.79619811426206510, -2.999999999999995559 ) ) ;
#9401=CARTESIAN_POINT ( 'NONE',  ( -22.97438720605730822, 22.98755168577401520, -7.000000000000006217 ) ) ;
#9403=DIRECTION ( 'NONE',  ( -6.505213034913038160E-19, -3.903127820947822896E-18, -1.000000000000000000 ) ) ;
#9409=ORIENTED_EDGE ( 'NONE', *, *, #18428, .F. ) ;
#9412=CARTESIAN_POINT ( 'NONE',  ( -24.24871130596417856, 13.99999999999976197, -2.999999999999999112 ) ) ;
#9413=CIRCLE ( 'NONE', #15967, 19.11328065563150957 ) ;
#9416=DIRECTION ( 'NONE',  ( 1.000000000000000000, 0.000000000000000000, 0.000000000000000000 ) ) ;
#9421=B_SPLINE_CURVE_WITH_KNOTS ( 'NONE', 3,
 ( #10146, #13918, #1686, #10370 ),
 .UNSPECIFIED., .F., .F.,
 ( 4, 4 ),
 ( 9.715086407230427146E-07, 0.001929643240672483445 ),
 .UNSPECIFIED. ) ;
#9431=DIRECTION ( 'NONE',  ( 6.505213034913038160E-19, 3.903127820947822896E-18, 1.000000000000000000 ) ) ;
#9432=DIRECTION ( 'NONE',  ( 1.000000000000000000, 0.000000000000000000, 0.000000000000000000 ) ) ;
#9433=ORIENTED_EDGE ( 'NONE', *, *, #8740, .T. ) ;
#9435=DIRECTION ( 'NONE',  ( 1.000000000000000000, 1.208970125616053475E-17, 0.000000000000000000 ) ) ;
#9439=EDGE_CURVE ( 'NONE', #15365, #13797, #19687, .T. ) ;
#9444=CIRCLE ( 'NONE', #2489, 36.76383501243555685 ) ;
#9452=AXIS2_PLACEMENT_3D ( 'NONE', #1822, #15774, #7075 ) ;
#9456=CIRCLE ( 'NONE', #5786, 36.76383501243555685 ) ;
#9465=ORIENTED_EDGE ( 'NONE', *, *, #5139, .T. ) ;
#9467=CARTESIAN_POINT ( 'NONE',  ( -33.52953626616031357, -9.708269511265493534, 3.000000000000016431 ) ) ;
#9469=EDGE_CURVE ( 'NONE', #573, #260, #11681, .T. ) ;
#9478=VECTOR ( 'NONE', #2356, 1000.000000000000000 ) ;
#9480=CARTESIAN_POINT ( 'NONE',  ( 22.26748298433284390, -22.28024240313525439, -6.999999999999950262 ) ) ;
#9485=ORIENTED_EDGE ( 'NONE', *, *, #15882, .F. ) ;
#9496=ORIENTED_EDGE ( 'NONE', *, *, #1518, .F. ) ;
#9500=DIRECTION ( 'NONE',  ( 6.505213034913038160E-19, 3.903127820947822896E-18, 1.000000000000000000 ) ) ;
#9504=CARTESIAN_POINT ( 'NONE',  ( -24.75236754129142724, -27.84804035626062202, -2.999999999999971578 ) ) ;
#9505=CARTESIAN_POINT ( 'NONE',  ( 2.775557561562891351E-14, -2.775557561562891351E-14, 2.999999999999999112 ) ) ;
#9506=EDGE_CURVE ( 'NONE', #13932, #8686, #15639, .T. ) ;
#9507=ADVANCED_FACE ( 'NONE', ( #18221 ), #20169, .T. ) ;
#9512=EDGE_LOOP ( 'NONE', ( #22215, #13171, #4751, #4738, #11045, #11251 ) ) ;
#9514=DIRECTION ( 'NONE',  ( -1.000000000000000000, 9.802091999852178833E-15, 0.000000000000000000 ) ) ;
#9517=CARTESIAN_POINT ( 'NONE',  ( -27.64365646977275048, -17.09029715894938661, -6.999999999999950262 ) ) ;
#9519=DIRECTION ( 'NONE',  ( 6.505213034913038160E-19, 3.903127820947822896E-18, 1.000000000000000000 ) ) ;
#9520=CARTESIAN_POINT ( 'NONE',  ( -10.00000000000000888, 2.999999999999836131, -4.999999999999948486 ) ) ;
#9521=ORIENTED_EDGE ( 'NONE', *, *, #9794, .T. ) ;
#9528=LINE ( 'NONE', #19257, #2344 ) ;
#9530=ORIENTED_EDGE ( 'NONE', *, *, #2014, .F. ) ;
#9531=ORIENTED_EDGE ( 'NONE', *, *, #9970, .T. ) ;
#9533=ORIENTED_EDGE ( 'NONE', *, *, #6235, .T. ) ;
#9536=VECTOR ( 'NONE', #22304, 1000.000000000000000 ) ;
#9537=CARTESIAN_POINT ( 'NONE',  ( -8.999999999999952038, 0.000000000000000000, -4.999999999999997335 ) ) ;
#9540=ORIENTED_EDGE ( 'NONE', *, *, #8890, .F. ) ;
#9544=DIRECTION ( 'NONE',  ( -6.505213034913038160E-19, -3.903127820947822896E-18, -1.000000000000000000 ) ) ;
#9545=EDGE_CURVE ( 'NONE', #1795, #22114, #7220, .T. ) ;
#9546=DIRECTION ( 'NONE',  ( -6.505213034913038160E-19, -3.903127820947822896E-18, -1.000000000000000000 ) ) ;
#9548=ORIENTED_EDGE ( 'NONE', *, *, #5522, .T. ) ;
#9553=ORIENTED_EDGE ( 'NONE', *, *, #14038, .F. ) ;
#9554=DIRECTION ( 'NONE',  ( -6.505213034913038160E-19, -3.903127820947822896E-18, -1.000000000000000000 ) ) ;
#9559=FACE_OUTER_BOUND ( 'NONE', #7867, .T. ) ;
#9565=ORIENTED_EDGE ( 'NONE', *, *, #6995, .F. ) ;
#9566=CARTESIAN_POINT ( 'NONE',  ( 26.65040777864179944, 24.43568323314229929, 2.932460736555799752 ) ) ;
#9568=ORIENTED_EDGE ( 'NONE', *, *, #16859, .F. ) ;
#9569=CARTESIAN_POINT ( 'NONE',  ( 1.423424233832903951, 32.35999952201579077, 3.000000000000002665 ) ) ;
#9574=DIRECTION ( 'NONE',  ( 6.505213034913038160E-19, 3.903127820947822896E-18, 1.000000000000000000 ) ) ;
#9576=CARTESIAN_POINT ( 'NONE',  ( 3.330669073875469621E-13, -1.110223024625156540E-13, -2.999999999999971578 ) ) ;
#9581=VERTEX_POINT ( 'NONE', #7083 ) ;
#9587=DIRECTION ( 'NONE',  ( -6.505213034913038160E-19, -3.903127820947822896E-18, -1.000000000000000000 ) ) ;
#9594=DIRECTION ( 'NONE',  ( -1.000000000000000000, 0.000000000000000000, 0.000000000000000000 ) ) ;
#9595=DIRECTION ( 'NONE',  ( -1.000000000000000000, -1.208970125616046080E-17, 6.505213034913038160E-19 ) ) ;
#9598=EDGE_CURVE ( 'NONE', #1297, #5408, #13634, .T. ) ;
#9602=ORIENTED_EDGE ( 'NONE', *, *, #12811, .T. ) ;
#9603=DIRECTION ( 'NONE',  ( -1.000000000000000000, -1.208970125616062874E-17, 0.000000000000000000 ) ) ;
#9611=DIRECTION ( 'NONE',  ( 1.000000000000000000, 0.000000000000000000, 0.000000000000000000 ) ) ;
#9617=CARTESIAN_POINT ( 'NONE',  ( -26.64365646977265456, -17.09029715894938661, -2.999999999999981792 ) ) ;
#9619=EDGE_CURVE ( 'NONE', #14924, #2722, #427, .T. ) ;
#9622=AXIS2_PLACEMENT_3D ( 'NONE', #13569, #20581, #4443 ) ;
#9624=ORIENTED_EDGE ( 'NONE', *, *, #17951, .F. ) ;
#9625=CARTESIAN_POINT ( 'NONE',  ( 24.03323817228489290, -20.36304159388394197, -7.000000000000006217 ) ) ;
#9627=CARTESIAN_POINT ( 'NONE',  ( -31.41239365194207878, 2.347663744114270035, 3.000000000000023537 ) ) ;
#9629=ORIENTED_EDGE ( 'NONE', *, *, #4570, .F. ) ;
#9633=DIRECTION ( 'NONE',  ( -6.505213034913038160E-19, -3.903127820947822896E-18, -1.000000000000000000 ) ) ;
#9636=AXIS2_PLACEMENT_3D ( 'NONE', #15074, #784, #19918 ) ;
#9643=CARTESIAN_POINT ( 'NONE',  ( -11.93972437435557232, -29.14949368109881433, -2.999999999999971578 ) ) ;
#9646=CARTESIAN_POINT ( 'NONE',  ( -27.01645732367859054, -17.86915608785693976, -2.999999999999999112 ) ) ;
#9648=CARTESIAN_POINT ( 'NONE',  ( 24.62019382530525391, -4.341204441673101933, -2.999999999999999112 ) ) ;
#9654=CIRCLE ( 'NONE', #14808, 34.90673715956759082 ) ;
#9663=ORIENTED_EDGE ( 'NONE', *, *, #18719, .T. ) ;
#9667=LINE ( 'NONE', #21944, #16951 ) ;
#9668=CARTESIAN_POINT ( 'NONE',  ( 31.21605069118088593, 8.646032897228984382, -2.999999999999999112 ) ) ;
#9670=B_SPLINE_CURVE_WITH_KNOTS ( 'NONE', 3,
 ( #11029, #18016, #2787, #2327 ),
 .UNSPECIFIED., .F., .F.,
 ( 4, 4 ),
 ( 0.001875451646902858305, 0.003761979286331158800 ),
 .UNSPECIFIED. ) ;
#9672=ORIENTED_EDGE ( 'NONE', *, *, #16557, .T. ) ;
#9676=EDGE_LOOP ( 'NONE', ( #12787, #11279, #9790, #11955, #15254, #8076 ) ) ;
#9684=DIRECTION ( 'NONE',  ( -1.000000000000000000, -1.208970125616057944E-17, 0.000000000000000000 ) ) ;
#9685=AXIS2_PLACEMENT_3D ( 'NONE', #15370, #15710, #1408 ) ;
#9693=DIRECTION ( 'NONE',  ( -6.505213034913038160E-19, -3.903127820947822896E-18, -1.000000000000000000 ) ) ;
#9696=ORIENTED_EDGE ( 'NONE', *, *, #10802, .T. ) ;
#9700=ADVANCED_FACE ( 'NONE', ( #19102 ), #15183, .T. ) ;
#9701=LINE ( 'NONE', #21979, #6748 ) ;
#9704=DIRECTION ( 'NONE',  ( 6.505213034913038160E-19, 3.903127820947822896E-18, 1.000000000000000000 ) ) ;
#9706=FACE_OUTER_BOUND ( 'NONE', #21824, .T. ) ;
#9721=FACE_OUTER_BOUND ( 'NONE', #21418, .T. ) ;
#9725=AXIS2_PLACEMENT_3D ( 'NONE', #18305, #2622, #9594 ) ;
#9729=TOROIDAL_SURFACE ( 'NONE', #18880, 34.90673715956759082, 8.750000000000000000 ) ;
#9734=DIRECTION ( 'NONE',  ( 6.505213034913038160E-19, 3.903127820947822896E-18, 1.000000000000000000 ) ) ;
#9735=EDGE_CURVE ( 'NONE', #5053, #12342, #6143, .T. ) ;
#9741=EDGE_CURVE ( 'NONE', #18413, #20053, #18949, .T. ) ;
#9743=DIRECTION ( 'NONE',  ( -1.000000000000000000, 0.000000000000000000, 0.000000000000000000 ) ) ;
#9744=FACE_BOUND ( 'NONE', #6951, .T. ) ;
#9746=DIRECTION ( 'NONE',  ( -6.505213034913038160E-19, -3.903127820947822896E-18, -1.000000000000000000 ) ) ;
#9750=AXIS2_PLACEMENT_3D ( 'NONE', #11815, #10207, #10090 ) ;
#9753=CIRCLE ( 'NONE', #18487, 19.11328065563152379 ) ;
#9756=ORIENTED_EDGE ( 'NONE', *, *, #1783, .T. ) ;
#9765=FACE_OUTER_BOUND ( 'NONE', #6497, .T. ) ;
#9766=B_SPLINE_CURVE_WITH_KNOTS ( 'NONE', 3,
 ( #2813, #11735, #13317, #11516 ),
 .UNSPECIFIED., .F., .F.,
 ( 4, 4 ),
 ( 9.715086409671343166E-07, 0.001929643240672210443 ),
 .UNSPECIFIED. ) ;
#9767=DIRECTION ( 'NONE',  ( 6.505213034913038160E-19, 3.903127820947822896E-18, 1.000000000000000000 ) ) ;
#9768=ORIENTED_EDGE ( 'NONE', *, *, #12286, .T. ) ;
#9770=AXIS2_PLACEMENT_3D ( 'NONE', #11117, #4373, #19737 ) ;
#9772=DIRECTION ( 'NONE',  ( -1.000000000000000000, -1.208970125616077665E-17, 0.000000000000000000 ) ) ;
#9776=ORIENTED_EDGE ( 'NONE', *, *, #7504, .T. ) ;
#9784=AXIS2_PLACEMENT_3D ( 'NONE', #21692, #7259, #17676 ) ;
#9785=AXIS2_PLACEMENT_3D ( 'NONE', #18074, #5935, #4007 ) ;
#9786=ORIENTED_EDGE ( 'NONE', *, *, #11589, .F. ) ;
#9787=ADVANCED_FACE ( 'NONE', ( #5016 ), #8553, .T. ) ;
#9790=ORIENTED_EDGE ( 'NONE', *, *, #21239, .T. ) ;
#9793=AXIS2_PLACEMENT_3D ( 'NONE', #2919, #1178, #13534 ) ;
#9794=EDGE_CURVE ( 'NONE', #14529, #13542, #17479, .T. ) ;
#9798=CARTESIAN_POINT ( 'NONE',  ( 24.24871130596423185, 14.00000000000009592, -4.999999999999948486 ) ) ;
#9799=VERTEX_POINT ( 'NONE', #2960 ) ;
#9803=VERTEX_POINT ( 'NONE', #10265 ) ;
#9804=DIRECTION ( 'NONE',  ( -6.505213034913038160E-19, -3.903127820947822896E-18, -1.000000000000000000 ) ) ;
#9807=CIRCLE ( 'NONE', #6515, 31.50000000000000711 ) ;
#9809=EDGE_CURVE ( 'NONE', #19379, #4478, #19330, .T. ) ;
#9810=FACE_OUTER_BOUND ( 'NONE', #11953, .T. ) ;
#9811=AXIS2_PLACEMENT_3D ( 'NONE', #7406, #3865, #16340 ) ;
#9813=CIRCLE ( 'NONE', #22643, 19.11328065563151668 ) ;
#9815=EDGE_LOOP ( 'NONE', ( #20179, #12551, #19829, #365 ) ) ;
#9825=ORIENTED_EDGE ( 'NONE', *, *, #4636, .F. ) ;
#9827=DIRECTION ( 'NONE',  ( -1.000000000000000000, -1.208970125616044077E-17, 0.000000000000000000 ) ) ;
#9828=DIRECTION ( 'NONE',  ( -1.000000000000000000, 0.000000000000000000, 0.000000000000000000 ) ) ;
#9833=EDGE_LOOP ( 'NONE', ( #2963, #14464, #19078, #13299 ) ) ;
#9840=VERTEX_POINT ( 'NONE', #22551 ) ;
#9845=AXIS2_PLACEMENT_3D ( 'NONE', #11927, #5180, #22605 ) ;
#9847=EDGE_CURVE ( 'NONE', #13884, #5071, #15261, .T. ) ;
#9848=DIRECTION ( 'NONE',  ( 6.505213034913038160E-19, 3.903127820947822896E-18, 1.000000000000000000 ) ) ;
#9856=DIRECTION ( 'NONE',  ( -6.505213034913038160E-19, -3.903127820947822896E-18, -1.000000000000000000 ) ) ;
#9858=ORIENTED_EDGE ( 'NONE', *, *, #908, .F. ) ;
#9859=CYLINDRICAL_SURFACE ( 'NONE', #15227, 0.9999999999999974465 ) ;
#9861=CARTESIAN_POINT ( 'NONE',  ( -22.26748298433245310, 22.28024240313483517, -2.999999999999975131 ) ) ;
#9863=ORIENTED_EDGE ( 'NONE', *, *, #1400, .T. ) ;
#9864=FACE_OUTER_BOUND ( 'NONE', #11776, .T. ) ;
#9872=CARTESIAN_POINT ( 'NONE',  ( -31.57187188083515750, -7.711478842616581453, -7.000000000000006217 ) ) ;
#9875=ORIENTED_EDGE ( 'NONE', *, *, #21441, .F. ) ;
#9878=ORIENTED_EDGE ( 'NONE', *, *, #921, .T. ) ;
#9882=DIRECTION ( 'NONE',  ( 1.266830946243004623E-16, -1.000000000000000000, -3.903127820947817503E-18 ) ) ;
#9885=EDGE_LOOP ( 'NONE', ( #338, #12360 ) ) ;
#9899=CIRCLE ( 'NONE', #4415, 34.90673715956759082 ) ;
#9904=CARTESIAN_POINT ( 'NONE',  ( -5.074925817841774212, 32.10132595304123981, -2.999999999999999112 ) ) ;
#9905=ORIENTED_EDGE ( 'NONE', *, *, #1206, .F. ) ;
#9906=CARTESIAN_POINT ( 'NONE',  ( 3.330669073875469621E-13, -1.110223024625156540E-13, -2.999999999999971578 ) ) ;
#9921=ORIENTED_EDGE ( 'NONE', *, *, #18677, .T. ) ;
#9925=LINE ( 'NONE', #16691, #6343 ) ;
#9928=ORIENTED_EDGE ( 'NONE', *, *, #20605, .T. ) ;
#9931=DIRECTION ( 'NONE',  ( 6.505213034913038160E-19, 3.903127820947822896E-18, 1.000000000000000000 ) ) ;
#9935=DIRECTION ( 'NONE',  ( 6.505213034913038160E-19, 3.903127820947822896E-18, 1.000000000000000000 ) ) ;
#9936=DIRECTION ( 'NONE',  ( -1.000000000000000000, -1.208970125616063644E-17, 0.000000000000000000 ) ) ;
#9944=CARTESIAN_POINT ( 'NONE',  ( -14.29266125237881013, 28.07080038625059260, 2.999999999999995559 ) ) ;
#9946=DIRECTION ( 'NONE',  ( -1.000000000000000000, 0.000000000000000000, 0.000000000000000000 ) ) ;
#9948=EDGE_CURVE ( 'NONE', #9799, #13942, #410, .T. ) ;
#9963=AXIS2_PLACEMENT_3D ( 'NONE', #14815, #6015, #21839 ) ;
#9964=DIRECTION ( 'NONE',  ( -1.000000000000000000, 1.764267138144086878E-15, 0.000000000000000000 ) ) ;
#9967=ORIENTED_EDGE ( 'NONE', *, *, #22433, .F. ) ;
#9968=VERTEX_POINT ( 'NONE', #17941 ) ;
#9970=EDGE_CURVE ( 'NONE', #3873, #13393, #5563, .T. ) ;
#9971=DIRECTION ( 'NONE',  ( -1.000000000000000000, -1.208970125616063644E-17, 0.000000000000000000 ) ) ;
#9972=DIRECTION ( 'NONE',  ( -6.505213034913038160E-19, -3.903127820947822896E-18, -1.000000000000000000 ) ) ;
#9975=ORIENTED_EDGE ( 'NONE', *, *, #21397, .F. ) ;
#9977=DIRECTION ( 'NONE',  ( -1.000000000000000000, 0.000000000000000000, 0.000000000000000000 ) ) ;
#9998=ORIENTED_EDGE ( 'NONE', *, *, #5167, .F. ) ;
#10000=EDGE_LOOP ( 'NONE', ( #6520, #16161, #750, #4528 ) ) ;
#10003=DIRECTION ( 'NONE',  ( 6.505213034913038160E-19, 3.903127820947822896E-18, 1.000000000000000000 ) ) ;
#10008=DIRECTION ( 'NONE',  ( -6.505213034913038160E-19, -3.903127820947822896E-18, -1.000000000000000000 ) ) ;
#10012=CIRCLE ( 'NONE', #16958, 19.11328065563151668 ) ;
#10013=VERTEX_POINT ( 'NONE', #19220 ) ;
#10014=DIRECTION ( 'NONE',  ( 1.000000000000000000, 0.000000000000000000, 0.000000000000000000 ) ) ;
#10017=DIRECTION ( 'NONE',  ( -1.000000000000000000, -1.208970125616044077E-17, 0.000000000000000000 ) ) ;
#10018=CARTESIAN_POINT ( 'NONE',  ( -36.14481870267515262, 0.8626474017860440435, 2.932969818539048479 ) ) ;
#10019=AXIS2_PLACEMENT_3D ( 'NONE', #10523, #17182, #22590 ) ;
#10025=ORIENTED_EDGE ( 'NONE', *, *, #20702, .T. ) ;
#10030=DIRECTION ( 'NONE',  ( -1.000000000000000000, 0.000000000000000000, 0.000000000000000000 ) ) ;
#10031=DIRECTION ( 'NONE',  ( -1.000000000000000000, -1.208970125616060101E-17, 6.505213034913038160E-19 ) ) ;
#10032=DIRECTION ( 'NONE',  ( 1.000000000000000000, 1.208970125616053321E-17, 0.000000000000000000 ) ) ;
#10033=ORIENTED_EDGE ( 'NONE', *, *, #9970, .F. ) ;
#10034=LINE ( 'NONE', #10263, #18992 ) ;
#10041=ORIENTED_EDGE ( 'NONE', *, *, #527, .T. ) ;
#10042=DIRECTION ( 'NONE',  ( 6.505213034913038160E-19, 3.903127820947822896E-18, 1.000000000000000000 ) ) ;
#10043=DIRECTION ( 'NONE',  ( -1.000000000000000000, -1.208970125616060717E-17, 0.000000000000000000 ) ) ;
#10059=DIRECTION ( 'NONE',  ( 6.505213034913038160E-19, 3.903127820947822896E-18, 1.000000000000000000 ) ) ;
#10067=CIRCLE ( 'NONE', #13367, 8.750000000000000000 ) ;
#10070=DIRECTION ( 'NONE',  ( 1.000000000000000000, 0.000000000000000000, 0.000000000000000000 ) ) ;
#10071=CARTESIAN_POINT ( 'NONE',  ( 24.73600648735135721, -27.19760187735878532, 2.800654218530481465 ) ) ;
#10072=DIRECTION ( 'NONE',  ( -6.505213034913038160E-19, -3.903127820947822896E-18, -1.000000000000000000 ) ) ;
#10080=CIRCLE ( 'NONE', #11921, 0.9999999999999974465 ) ;
#10090=DIRECTION ( 'NONE',  ( 1.000000000000000000, 0.000000000000000000, 0.000000000000000000 ) ) ;
#10093=VERTEX_POINT ( 'NONE', #13215 ) ;
#10096=CARTESIAN_POINT ( 'NONE',  ( 3.608224830031758756E-13, -2.775557561562891351E-14, -4.999999999999997335 ) ) ;
#10100=CIRCLE ( 'NONE', #2432, 8.750000000000000000 ) ;
#10103=ORIENTED_EDGE ( 'NONE', *, *, #622, .F. ) ;
#10108=VECTOR ( 'NONE', #21507, 1000.000000000000000 ) ;
#10112=ORIENTED_EDGE ( 'NONE', *, *, #7753, .T. ) ;
#10121=ORIENTED_EDGE ( 'NONE', *, *, #21039, .F. ) ;
#10124=DIRECTION ( 'NONE',  ( 6.505213034913038160E-19, 3.903127820947822896E-18, 1.000000000000000000 ) ) ;
#10127=CARTESIAN_POINT ( 'NONE',  ( -35.79662727779865605, 4.171001175319267062, -2.999999999999971578 ) ) ;
#10131=AXIS2_PLACEMENT_3D ( 'NONE', #10804, #21251, #22435 ) ;
#10133=ORIENTED_EDGE ( 'NONE', *, *, #20469, .T. ) ;
#10134=ORIENTED_EDGE ( 'NONE', *, *, #6109, .T. ) ;
#10144=AXIS2_PLACEMENT_3D ( 'NONE', #2614, #9587, #16576 ) ;
#10145=VERTEX_POINT ( 'NONE', #4200 ) ;
#10146=CARTESIAN_POINT ( 'NONE',  ( -35.16985127952398926, -10.70799354677417980, 2.800654218530485018 ) ) ;
#10151=CYLINDRICAL_SURFACE ( 'NONE', #5333, 1.000000000000000888 ) ;
#10152=EDGE_CURVE ( 'NONE', #5255, #17600, #19786, .T. ) ;
#10153=ORIENTED_EDGE ( 'NONE', *, *, #9948, .F. ) ;
#10155=LINE ( 'NONE', #5022, #16094 ) ;
#10156=ORIENTED_EDGE ( 'NONE', *, *, #13058, .T. ) ;
#10160=CYLINDRICAL_SURFACE ( 'NONE', #2435, 1.000000000000001776 ) ;
#10164=VERTEX_POINT ( 'NONE', #18172 ) ;
#10167=CYLINDRICAL_SURFACE ( 'NONE', #17467, 19.11328065563152379 ) ;
#10169=AXIS2_PLACEMENT_3D ( 'NONE', #8086, #18731, #14933 ) ;
#10170=CIRCLE ( 'NONE', #19720, 36.76383501243555685 ) ;
#10171=CARTESIAN_POINT ( 'NONE',  ( 2.775557561562891351E-14, -2.775557561562891351E-14, 2.999999999999999112 ) ) ;
#10189=AXIS2_PLACEMENT_3D ( 'NONE', #9648, #18592, #16639 ) ;
#10190=CARTESIAN_POINT ( 'NONE',  ( 21.65063509461118230, 12.49999999999984368, -2.999999999999988898 ) ) ;
#10191=EDGE_CURVE ( 'NONE', #8443, #2570, #14918, .T. ) ;
#10195=ORIENTED_EDGE ( 'NONE', *, *, #8128, .T. ) ;
#10198=DIRECTION ( 'NONE',  ( 6.505213034913038160E-19, 3.903127820947822896E-18, 1.000000000000000000 ) ) ;
#10199=CARTESIAN_POINT ( 'NONE',  ( -10.70799354677373572, 35.16985127952371215, 2.800654218530492123 ) ) ;
#10201=CARTESIAN_POINT ( 'NONE',  ( 24.03323817228486448, -20.36304159388385671, -2.999999999999975131 ) ) ;
#10202=ORIENTED_EDGE ( 'NONE', *, *, #16466, .F. ) ;
#10205=VERTEX_POINT ( 'NONE', #4875 ) ;
#10206=CARTESIAN_POINT ( 'NONE',  ( 25.34312177887374062, -20.17230487860824439, 2.999999999999995559 ) ) ;
#10207=DIRECTION ( 'NONE',  ( 6.505213034913038160E-19, 3.903127820947822896E-18, 1.000000000000000000 ) ) ;
#10213=EDGE_LOOP ( 'NONE', ( #6948, #6986, #444, #21547 ) ) ;
#10214=CYLINDRICAL_SURFACE ( 'NONE', #10473, 28.00000000000000355 ) ;
#10218=B_SPLINE_CURVE_WITH_KNOTS ( 'NONE', 3,
 ( #1388, #13614, #4941, #5174 ),
 .UNSPECIFIED., .F., .F.,
 ( 4, 4 ),
 ( 0.001875451646902801927, 0.003761979286331116300 ),
 .UNSPECIFIED. ) ;
#10223=B_SPLINE_CURVE_WITH_KNOTS ( 'NONE', 3,
 ( #6025, #12992, #11291, #18283 ),
 .UNSPECIFIED., .F., .F.,
 ( 4, 4 ),
 ( 9.545285770017924652E-07, 0.001900595205834839339 ),
 .UNSPECIFIED. ) ;
#10224=ORIENTED_EDGE ( 'NONE', *, *, #2927, .F. ) ;
#10227=EDGE_CURVE ( 'NONE', #10164, #12187, #1041, .T. ) ;
#10229=FACE_OUTER_BOUND ( 'NONE', #15701, .T. ) ;
#10232=ORIENTED_EDGE ( 'NONE', *, *, #9469, .F. ) ;
#10235=ORIENTED_EDGE ( 'NONE', *, *, #1499, .T. ) ;
#10241=ORIENTED_EDGE ( 'NONE', *, *, #21539, .F. ) ;
#10242=LINE ( 'NONE', #17347, #21069 ) ;
#10250=ORIENTED_EDGE ( 'NONE', *, *, #7919, .F. ) ;
#10256=LINE ( 'NONE', #7053, #22446 ) ;
#10257=B_SPLINE_CURVE_WITH_KNOTS ( 'NONE', 3,
 ( #17236, #1551, #10472, #15511 ),
 .UNSPECIFIED., .F., .F.,
 ( 4, 4 ),
 ( 0.001893031756885730620, 0.003808480026564045606 ),
 .UNSPECIFIED. ) ;
#10258=DIRECTION ( 'NONE',  ( 1.000000000000000000, 1.208970125616062874E-17, 0.000000000000000000 ) ) ;
#10259=CARTESIAN_POINT ( 'NONE',  ( 32.09841355226000559, -5.093313992686448799, -6.999999999999992006 ) ) ;
#10262=VERTEX_POINT ( 'NONE', #13557 ) ;
#10263=CARTESIAN_POINT ( 'NONE',  ( -4.074925817841801745, 32.10132595304121850, -6.999999999999950262 ) ) ;
#10265=CARTESIAN_POINT ( 'NONE',  ( -14.67611967928904271, 31.67162468655987340, 3.000000000000009770 ) ) ;
#10267=CARTESIAN_POINT ( 'NONE',  ( -12.31876324338268525, -30.07487443287973505, 2.999999999999995559 ) ) ;
#10268=ORIENTED_EDGE ( 'NONE', *, *, #18355, .T. ) ;
#10271=CARTESIAN_POINT ( 'NONE',  ( 5.074925817841801745, -32.10132595304126824, -6.999999999999999112 ) ) ;
#10274=LINE ( 'NONE', #12007, #2021 ) ;
#10277=ADVANCED_FACE ( 'NONE', ( #20569 ), #18634, .T. ) ;
#10279=LINE ( 'NONE', #20952, #8930 ) ;
#10281=VERTEX_POINT ( 'NONE', #12386 ) ;
#10284=DIRECTION ( 'NONE',  ( 6.505213034913038160E-19, 3.903127820947822896E-18, 1.000000000000000000 ) ) ;
#10285=CARTESIAN_POINT ( 'NONE',  ( 9.708269511265326557, -33.52953626616050542, 3.000000000000002665 ) ) ;
#10291=EDGE_CURVE ( 'NONE', #12599, #22498, #15291, .T. ) ;
#10292=DIRECTION ( 'NONE',  ( -1.000000000000000000, -1.208970125616081209E-17, 0.000000000000000000 ) ) ;
#10293=DIRECTION ( 'NONE',  ( -6.505213034913038160E-19, -3.903127820947822896E-18, -1.000000000000000000 ) ) ;
#10294=ORIENTED_EDGE ( 'NONE', *, *, #2716, .F. ) ;
#10302=EDGE_LOOP ( 'NONE', ( #11456, #17918, #5283, #12593 ) ) ;
#10303=DIRECTION ( 'NONE',  ( 1.000000000000000000, 0.000000000000000000, 0.000000000000000000 ) ) ;
#10305=DIRECTION ( 'NONE',  ( 6.505213034913038160E-19, 3.903127820947822896E-18, 1.000000000000000000 ) ) ;
#10317=ADVANCED_FACE ( 'NONE', ( #8095 ), #22068, .T. ) ;
#10319=CARTESIAN_POINT ( 'NONE',  ( 14.67611967928950101, -31.67162468656004037, -2.999999999999995559 ) ) ;
#10320=ORIENTED_EDGE ( 'NONE', *, *, #16707, .F. ) ;
#10326=CIRCLE ( 'NONE', #458, 0.9999999999999974465 ) ;
#10328=ORIENTED_EDGE ( 'NONE', *, *, #5558, .T. ) ;
#10336=CARTESIAN_POINT ( 'NONE',  ( -22.98755168577413954, -22.97438720605751783, 2.999999999999999112 ) ) ;
#10345=CARTESIAN_POINT ( 'NONE',  ( -2.422192751863949667, -32.40961249803553557, -2.999999999999971578 ) ) ;
#10348=AXIS2_PLACEMENT_3D ( 'NONE', #13801, #1798, #19212 ) ;
#10369=ORIENTED_EDGE ( 'NONE', *, *, #2498, .F. ) ;
#10370=CARTESIAN_POINT ( 'NONE',  ( -33.52953626616031357, -9.708269511265493534, 3.000000000000016431 ) ) ;
#10376=EDGE_CURVE ( 'NONE', #20150, #14303, #20722, .T. ) ;
#10377=ORIENTED_EDGE ( 'NONE', *, *, #8821, .T. ) ;
#10378=AXIS2_PLACEMENT_3D ( 'NONE', #5815, #12788, #18061 ) ;
#10381=DIRECTION ( 'NONE',  ( -6.505213034913038160E-19, -3.903127820947822896E-18, -1.000000000000000000 ) ) ;
#10390=FACE_OUTER_BOUND ( 'NONE', #12639, .T. ) ;
#10391=ADVANCED_FACE ( 'NONE', ( #2192 ), #10764, .F. ) ;
#10392=DIRECTION ( 'NONE',  ( -1.000000000000000000, 0.000000000000000000, 0.000000000000000000 ) ) ;
#10399=DIRECTION ( 'NONE',  ( -6.505213034913038160E-19, -3.903127820947822896E-18, -1.000000000000000000 ) ) ;
#10403=CARTESIAN_POINT ( 'NONE',  ( -31.21605069118050935, -8.646032897229344982, 3.000000000000023537 ) ) ;
#10406=DIRECTION ( 'NONE',  ( -1.000000000000000000, -1.208970125616060717E-17, 0.000000000000000000 ) ) ;
#10410=PRODUCT_CONTEXT ( 'NONE', #16917, 'mechanical' ) ;
#10412=B_SPLINE_CURVE_WITH_KNOTS ( 'NONE', 3,
 ( #15284, #986, #16677, #2823 ),
 .UNSPECIFIED., .F., .F.,
 ( 4, 4 ),
 ( 9.545285769851497501E-07, 0.001900595205834582383 ),
 .UNSPECIFIED. ) ;
#10417=FACE_OUTER_BOUND ( 'NONE', #3895, .T. ) ;
#10420=ORIENTED_EDGE ( 'NONE', *, *, #22366, .F. ) ;
#10433=ADVANCED_FACE ( 'NONE', ( #17890 ), #9177, .T. ) ;
#10436=DIRECTION ( 'NONE',  ( -6.505213034913038160E-19, -3.903127820947822896E-18, -1.000000000000000000 ) ) ;
#10439=EDGE_CURVE ( 'NONE', #18993, #12370, #13497, .T. ) ;
#10440=TOROIDAL_SURFACE ( 'NONE', #203, 34.90673715956759082, 8.750000000000000000 ) ;
#10442=VECTOR ( 'NONE', #21080, 1000.000000000000000 ) ;
#10444=TOROIDAL_SURFACE ( 'NONE', #18871, 34.90673715956759082, 8.750000000000000000 ) ;
#10449=CARTESIAN_POINT ( 'NONE',  ( -11.85401191286875111, -32.83234229683740324, 3.000000000000023537 ) ) ;
#10457=AXIS2_PLACEMENT_3D ( 'NONE', #12324, #5350, #17940 ) ;
#10464=CYLINDRICAL_SURFACE ( 'NONE', #15569, 36.76383501243555685 ) ;
#10468=CARTESIAN_POINT ( 'NONE',  ( 24.79619811426203668, -21.00948735876886886, -2.999999999999999112 ) ) ;
#10469=EDGE_CURVE ( 'NONE', #7786, #2949, #6023, .T. ) ;
#10472=CARTESIAN_POINT ( 'NONE',  ( 10.35112103033899622, -34.64554704988861999, -2.932164912090521991 ) ) ;
#10473=AXIS2_PLACEMENT_3D ( 'NONE', #10096, #15135, #6336 ) ;
#10474=ORIENTED_EDGE ( 'NONE', *, *, #8194, .T. ) ;
#10477=VERTEX_POINT ( 'NONE', #4374 ) ;
#10480=DIRECTION ( 'NONE',  ( -6.505213034913038160E-19, -3.903127820947822896E-18, -1.000000000000000000 ) ) ;
#10481=CARTESIAN_POINT ( 'NONE',  ( -8.485281374238345720, -3.000000000000002665, 4.999999999999993783 ) ) ;
#10488=DIRECTION ( 'NONE',  ( -6.505213034913038160E-19, -3.903127820947822896E-18, -1.000000000000000000 ) ) ;
#10490=DIRECTION ( 'NONE',  ( -1.000000000000000000, 0.000000000000000000, 0.000000000000000000 ) ) ;
#10493=CYLINDRICAL_SURFACE ( 'NONE', #5058, 0.9999999999999974465 ) ;
#10496=DIRECTION ( 'NONE',  ( 1.000000000000000000, 1.208970125616063028E-17, 0.000000000000000000 ) ) ;
#10498=EDGE_LOOP ( 'NONE', ( #15334, #9051, #7592, #22448 ) ) ;
#10500=CIRCLE ( 'NONE', #4674, 34.90673715956759082 ) ;
#10503=CARTESIAN_POINT ( 'NONE',  ( -32.28023859650863159, -14.85562396683518749, -2.999999999999995559 ) ) ;
#10504=ORIENTED_EDGE ( 'NONE', *, *, #16466, .T. ) ;
#10505=EDGE_CURVE ( 'NONE', #17804, #14924, #3089, .T. ) ;
#10511=CARTESIAN_POINT ( 'NONE',  ( -11.35354668330684724, -30.33632613426204117, -2.999999999999971578 ) ) ;
#10512=ADVANCED_FACE ( 'NONE', ( #21904, #13385, #11228, #9744, #18227 ), #21784, .T. ) ;
#10513=TOROIDAL_SURFACE ( 'NONE', #5792, 34.90673715956759082, 8.750000000000000000 ) ;
#10521=ORIENTED_EDGE ( 'NONE', *, *, #5445, .T. ) ;
#10522=DIRECTION ( 'NONE',  ( -1.000000000000000000, -1.208970125616046080E-17, 6.505213034913038160E-19 ) ) ;
#10523=CARTESIAN_POINT ( 'NONE',  ( -7.094908322883119567, 35.33352588067076283, -6.999999999999950262 ) ) ;
#10525=VECTOR ( 'NONE', #17551, 1000.000000000000000 ) ;
#10528=AXIS2_PLACEMENT_3D ( 'NONE', #15161, #18737, #18851 ) ;
#10538=ORIENTED_EDGE ( 'NONE', *, *, #4142, .T. ) ;
#10541=DIRECTION ( 'NONE',  ( -1.000000000000000000, 0.000000000000000000, 0.000000000000000000 ) ) ;
#10545=CYLINDRICAL_SURFACE ( 'NONE', #2078, 0.9999999999999974465 ) ;
#10547=B_SPLINE_CURVE_WITH_KNOTS ( 'NONE', 3,
 ( #2463, #275, #7498, #21254 ),
 .UNSPECIFIED., .F., .F.,
 ( 4, 4 ),
 ( 9.545285770017924652E-07, 0.001900595205834748483 ),
 .UNSPECIFIED. ) ;
#10551=DIRECTION ( 'NONE',  ( -1.000000000000000000, -1.208970125616081209E-17, 0.000000000000000000 ) ) ;
#10552=DIRECTION ( 'NONE',  ( -6.505213034913038160E-19, -3.903127820947822896E-18, -1.000000000000000000 ) ) ;
#10556=ORIENTED_EDGE ( 'NONE', *, *, #8108, .T. ) ;
#10558=ORIENTED_EDGE ( 'NONE', *, *, #19075, .T. ) ;
#10560=ADVANCED_FACE ( 'NONE', ( #22010 ), #11458, .T. ) ;
#10562=EDGE_CURVE ( 'NONE', #18033, #2388, #7468, .T. ) ;
#10563=ORIENTED_EDGE ( 'NONE', *, *, #11310, .F. ) ;
#10567=CARTESIAN_POINT ( 'NONE',  ( 2.220446049250313081E-13, -8.326672684688674053E-14, 2.800654218530498785 ) ) ;
#10568=ORIENTED_EDGE ( 'NONE', *, *, #20591, .T. ) ;
#10572=CARTESIAN_POINT ( 'NONE',  ( -31.88709182564680589, 6.070730550690766947, 2.999999999999995559 ) ) ;
#10573=CARTESIAN_POINT ( 'NONE',  ( -30.60042966911723283, -7.474202570535854129, -2.999999999999971578 ) ) ;
#10587=ORIENTED_EDGE ( 'NONE', *, *, #3319, .F. ) ;
#10590=DIRECTION ( 'NONE',  ( -6.505213034913038160E-19, -3.903127820947822896E-18, -1.000000000000000000 ) ) ;
#10596=EDGE_CURVE ( 'NONE', #18180, #16900, #13306, .T. ) ;
#10601=CARTESIAN_POINT ( 'NONE',  ( -32.83234229683721850, 11.85401191286866762, -2.999999999999971578 ) ) ;
#10602=CIRCLE ( 'NONE', #4397, 31.50000000000000000 ) ;
#10609=EDGE_LOOP ( 'NONE', ( #2641, #8068, #5510, #8451 ) ) ;
#10610=ORIENTED_EDGE ( 'NONE', *, *, #5667, .T. ) ;
#10612=AXIS2_PLACEMENT_3D ( 'NONE', #17619, #3766, #15886 ) ;
#10618=CARTESIAN_POINT ( 'NONE',  ( 31.47226199422872028, -17.79229176513319288, -2.933296326616341876 ) ) ;
#10620=ORIENTED_EDGE ( 'NONE', *, *, #2034, .F. ) ;
#10627=CIRCLE ( 'NONE', #13560, 19.11328065563152023 ) ;
#10640=DIRECTION ( 'NONE',  ( -1.000000000000000000, 0.000000000000000000, 0.000000000000000000 ) ) ;
#10646=ORIENTED_EDGE ( 'NONE', *, *, #2498, .T. ) ;
#10653=CARTESIAN_POINT ( 'NONE',  ( -31.88709182564693378, 6.070730550690822902, -2.999999999999999112 ) ) ;
#10655=EDGE_CURVE ( 'NONE', #22114, #17215, #1997, .T. ) ;
#10658=ORIENTED_EDGE ( 'NONE', *, *, #15882, .T. ) ;
#10659=ORIENTED_EDGE ( 'NONE', *, *, #8924, .F. ) ;
#10669=CARTESIAN_POINT ( 'NONE',  ( 0.6841746959067585010, 36.75746821813302745, -2.800654218530457484 ) ) ;
#10687=DIRECTION ( 'NONE',  ( 6.505213034913038160E-19, 3.903127820947822896E-18, 1.000000000000000000 ) ) ;
#10688=CIRCLE ( 'NONE', #11795, 31.50000000000001421 ) ;
#10689=VERTEX_POINT ( 'NONE', #206 ) ;
#10690=VERTEX_POINT ( 'NONE', #14170 ) ;
#10693=ORIENTED_EDGE ( 'NONE', *, *, #12137, .T. ) ;
#10695=FACE_OUTER_BOUND ( 'NONE', #17272, .T. ) ;
#10706=FACE_OUTER_BOUND ( 'NONE', #15082, .T. ) ;
#10714=CARTESIAN_POINT ( 'NONE',  ( -23.74488952252773544, 25.58633464742632313, 3.000000000000023537 ) ) ;
#10724=EDGE_CURVE ( 'NONE', #11124, #18161, #14517, .T. ) ;
#10726=CARTESIAN_POINT ( 'NONE',  ( -30.33632613426162550, 11.35354668330676375, 2.999999999999995559 ) ) ;
#10727=FACE_OUTER_BOUND ( 'NONE', #2453, .T. ) ;
#10732=DIRECTION ( 'NONE',  ( 1.000000000000000000, 0.000000000000000000, 0.000000000000000000 ) ) ;
#10733=ORIENTED_EDGE ( 'NONE', *, *, #20824, .T. ) ;
#10734=DIRECTION ( 'NONE',  ( 6.505213034913038160E-19, 3.903127820947822896E-18, 1.000000000000000000 ) ) ;
#10739=AXIS2_PLACEMENT_3D ( 'NONE', #8947, #16273, #584 ) ;
#10740=VERTEX_POINT ( 'NONE', #14347 ) ;
#10745=CIRCLE ( 'NONE', #11132, 31.50000000000001421 ) ;
#10748=CIRCLE ( 'NONE', #8580, 0.9999999999999974465 ) ;
#10752=CARTESIAN_POINT ( 'NONE',  ( 20.17230487860832611, 25.34312177887321127, 3.000000000000009770 ) ) ;
#10755=CARTESIAN_POINT ( 'NONE',  ( -8.550503583141882302, 23.49231551964767206, -5.000000000000004441 ) ) ;
#10756=ORIENTED_EDGE ( 'NONE', *, *, #18807, .T. ) ;
#10757=DIRECTION ( 'NONE',  ( -1.000000000000000000, -3.564803380056654458E-15, 0.000000000000000000 ) ) ;
#10758=EDGE_CURVE ( 'NONE', #13475, #11887, #21355, .T. ) ;
#10760=CYLINDRICAL_SURFACE ( 'NONE', #4845, 19.11328065563151313 ) ;
#10764=CYLINDRICAL_SURFACE ( 'NONE', #10739, 2.999999999999999112 ) ;
#10766=CIRCLE ( 'NONE', #9339, 19.11328065563151668 ) ;
#10767=ORIENTED_EDGE ( 'NONE', *, *, #13298, .T. ) ;
#10769=CARTESIAN_POINT ( 'NONE',  ( 3.330669073875469621E-13, -1.110223024625156540E-13, -2.999999999999971578 ) ) ;
#10770=CARTESIAN_POINT ( 'NONE',  ( 34.74700806321118307, -12.00937115242653519, -2.800654218530457484 ) ) ;
#10771=B_SPLINE_CURVE_WITH_KNOTS ( 'NONE', 3,
 ( #12986, #18379, #9566, #20339 ),
 .UNSPECIFIED., .F., .F.,
 ( 4, 4 ),
 ( 0.001875451646903067990, 0.003761979286331190026 ),
 .UNSPECIFIED. ) ;
#10778=ORIENTED_EDGE ( 'NONE', *, *, #21736, .T. ) ;
#10781=B_SPLINE_CURVE_WITH_KNOTS ( 'NONE', 3,
 ( #15108, #18340, #2769, #2993 ),
 .UNSPECIFIED., .F., .F.,
 ( 4, 4 ),
 ( 0.001893031756885368063, 0.003808480026563666569 ),
 .UNSPECIFIED. ) ;
#10782=AXIS2_PLACEMENT_3D ( 'NONE', #19806, #11079, #18069 ) ;
#10786=ORIENTED_EDGE ( 'NONE', *, *, #13408, .T. ) ;
#10788=DIRECTION ( 'NONE',  ( -1.000000000000000000, 0.000000000000000000, 0.000000000000000000 ) ) ;
#10792=CARTESIAN_POINT ( 'NONE',  ( 34.24928931925769149, -6.742883674876604339, 3.000000000000002665 ) ) ;
#10794=ORIENTED_EDGE ( 'NONE', *, *, #13116, .T. ) ;
#10795=CARTESIAN_POINT ( 'NONE',  ( 34.74700806321121149, -12.00937115242670039, 2.800654218530512551 ) ) ;
#10796=ORIENTED_EDGE ( 'NONE', *, *, #18338, .T. ) ;
#10799=FACE_OUTER_BOUND ( 'NONE', #5812, .T. ) ;
#10802=EDGE_CURVE ( 'NONE', #18491, #2692, #18145, .T. ) ;
#10804=CARTESIAN_POINT ( 'NONE',  ( 2.220446049250313081E-13, -8.326672684688674053E-14, 2.800654218530498785 ) ) ;
#10807=CIRCLE ( 'NONE', #6800, 1.000000000000000888 ) ;
#10809=VERTEX_POINT ( 'NONE', #5540 ) ;
#10812=ORIENTED_EDGE ( 'NONE', *, *, #9794, .F. ) ;
#10813=AXIS2_PLACEMENT_3D ( 'NONE', #13895, #3061, #10032 ) ;
#10815=ORIENTED_EDGE ( 'NONE', *, *, #8080, .T. ) ;
#10817=FACE_OUTER_BOUND ( 'NONE', #17458, .T. ) ;
#10820=CARTESIAN_POINT ( 'NONE',  ( -31.41173278719236350, -17.66631876130928092, -6.999999999999950262 ) ) ;
#10821=DIRECTION ( 'NONE',  ( -1.000000000000000000, -1.208970125616077665E-17, 0.000000000000000000 ) ) ;
#10822=EDGE_CURVE ( 'NONE', #21718, #10976, #15756, .T. ) ;
#10824=VERTEX_POINT ( 'NONE', #5775 ) ;
#10825=LINE ( 'NONE', #15863, #4718 ) ;
#10827=CARTESIAN_POINT ( 'NONE',  ( -35.16985127952398926, -10.70799354677417980, 2.800654218530485018 ) ) ;
#10832=AXIS2_PLACEMENT_3D ( 'NONE', #8503, #22496, #15252 ) ;
#10833=DIRECTION ( 'NONE',  ( 1.000000000000000000, 1.208970125616063182E-17, 0.000000000000000000 ) ) ;
#10838=CIRCLE ( 'NONE', #15230, 0.9999999999999974465 ) ;
#10847=ADVANCED_FACE ( 'NONE', ( #19529 ), #4174, .F. ) ;
#10848=CYLINDRICAL_SURFACE ( 'NONE', #4787, 31.50000000000001421 ) ;
#10854=VECTOR ( 'NONE', #8863, 1000.000000000000000 ) ;
#10860=EDGE_LOOP ( 'NONE', ( #2583, #19877, #17019, #18528 ) ) ;
#10862=AXIS2_PLACEMENT_3D ( 'NONE', #15127, #9544, #13407 ) ;
#10864=AXIS2_PLACEMENT_3D ( 'NONE', #21888, #1022, #4470 ) ;
#10866=EDGE_LOOP ( 'NONE', ( #1328, #9531, #20927, #19129, #21430, #21422 ) ) ;
#10871=B_SPLINE_CURVE_WITH_KNOTS ( 'NONE', 3,
 ( #15158, #381, #17455, #22035 ),
 .UNSPECIFIED., .F., .F.,
 ( 4, 4 ),
 ( 0.001893031756885371316, 0.003808480026563539934 ),
 .UNSPECIFIED. ) ;
#10872=AXIS2_PLACEMENT_3D ( 'NONE', #17419, #13863, #3690 ) ;
#10874=FACE_OUTER_BOUND ( 'NONE', #11100, .T. ) ;
#10875=VECTOR ( 'NONE', #7880, 1000.000000000000000 ) ;
#10876=ORIENTED_EDGE ( 'NONE', *, *, #331, .T. ) ;
#10879=ORIENTED_EDGE ( 'NONE', *, *, #19405, .F. ) ;
#10880=DIRECTION ( 'NONE',  ( 6.505213034913038160E-19, 3.903127820947822896E-18, 1.000000000000000000 ) ) ;
#10881=LINE ( 'NONE', #16144, #7960 ) ;
#10882=AXIS2_PLACEMENT_3D ( 'NONE', #20603, #4699, #11675 ) ;
#10885=EDGE_CURVE ( 'NONE', #768, #7786, #21702, .T. ) ;
#10886=DIRECTION ( 'NONE',  ( 6.505213034913038160E-19, 3.903127820947822896E-18, 1.000000000000000000 ) ) ;
#10888=CARTESIAN_POINT ( 'NONE',  ( -34.90673715956753398, -1.391998901022310567E-13, -5.749999999999949374 ) ) ;
#10895=DIRECTION ( 'NONE',  ( 6.505213034913038160E-19, 3.903127820947822896E-18, 1.000000000000000000 ) ) ;
#10901=VERTEX_POINT ( 'NONE', #956 ) ;
#10902=ORIENTED_EDGE ( 'NONE', *, *, #443, .T. ) ;
#10904=DIRECTION ( 'NONE',  ( -1.000000000000000000, 0.000000000000000000, 0.000000000000000000 ) ) ;
#10905=CARTESIAN_POINT ( 'NONE',  ( 2.220446049250313081E-13, 2.775557561562891351E-14, -2.800654218530485018 ) ) ;
#10909=ORIENTED_EDGE ( 'NONE', *, *, #21208, .T. ) ;
#10910=CARTESIAN_POINT ( 'NONE',  ( 2.220446049250313081E-13, 2.775557561562891351E-14, -2.800654218530485018 ) ) ;
#10911=CARTESIAN_POINT ( 'NONE',  ( -21.00948735876860596, -24.79619811426211839, 2.999999999999995559 ) ) ;
#10913=CARTESIAN_POINT ( 'NONE',  ( -34.24928931925764886, 6.742883674876548383, 2.999999999999999112 ) ) ;
#10914=LINE ( 'NONE', #9199, #8282 ) ;
#10916=CARTESIAN_POINT ( 'NONE',  ( 23.74488952252801255, -25.58633464742643326, -2.999999999999978240 ) ) ;
#10918=DIRECTION ( 'NONE',  ( 6.505213034913038160E-19, 3.903127820947822896E-18, 1.000000000000000000 ) ) ;
#10924=EDGE_LOOP ( 'NONE', ( #13973, #22029, #14506, #18324, #19021, #7893 ) ) ;
#10925=DIRECTION ( 'NONE',  ( 6.505213034913038160E-19, 3.903127820947822896E-18, 1.000000000000000000 ) ) ;
#10927=CARTESIAN_POINT ( 'NONE',  ( 27.19760187735878532, 24.73600648735102681, -2.800654218530485018 ) ) ;
#10929=CIRCLE ( 'NONE', #5459, 1.000000000000000888 ) ;
#10938=EDGE_CURVE ( 'NONE', #17505, #17561, #15516, .T. ) ;
#10941=PRODUCT ( 'GEAR', 'GEAR', '', ( #10410 ) ) ;
#10944=CYLINDRICAL_SURFACE ( 'NONE', #14578, 19.11328065563152379 ) ;
#10945=CARTESIAN_POINT ( 'NONE',  ( 15.12081897056688540, -33.51030287062373247, 2.800654218530485018 ) ) ;
#10953=EDGE_CURVE ( 'NONE', #4765, #16523, #3249, .T. ) ;
#10958=EDGE_LOOP ( 'NONE', ( #9116, #19137, #15021, #5435 ) ) ;
#10959=ORIENTED_EDGE ( 'NONE', *, *, #11589, .T. ) ;
#10962=EDGE_CURVE ( 'NONE', #19759, #10205, #10748, .T. ) ;
#10965=CARTESIAN_POINT ( 'NONE',  ( -35.99819890246953946, 7.463862311151231665, 2.800654218530509443 ) ) ;
#10967=DIRECTION ( 'NONE',  ( -1.000000000000000000, -1.208970125616060101E-17, 6.505213034913038160E-19 ) ) ;
#10972=DIRECTION ( 'NONE',  ( -6.505213034913038160E-19, -3.903127820947822896E-18, -1.000000000000000000 ) ) ;
#10975=CIRCLE ( 'NONE', #16840, 1.000000000000000888 ) ;
#10976=VERTEX_POINT ( 'NONE', #10319 ) ;
#10977=CYLINDRICAL_SURFACE ( 'NONE', #16368, 31.50000000000001421 ) ;
#10979=DIRECTION ( 'NONE',  ( 1.000000000000000000, 0.000000000000000000, 0.000000000000000000 ) ) ;
#10983=DIRECTION ( 'NONE',  ( -6.505213034913038160E-19, -3.903127820947822896E-18, -1.000000000000000000 ) ) ;
#10992=ORIENTED_EDGE ( 'NONE', *, *, #2501, .T. ) ;
#10993=CARTESIAN_POINT ( 'NONE',  ( -4.104166344909047304, 35.92356703407487117, 2.932460736555809966 ) ) ;
#11000=ORIENTED_EDGE ( 'NONE', *, *, #9050, .T. ) ;
#11001=CARTESIAN_POINT ( 'NONE',  ( -21.69710536060276596, -28.14364593009914017, 3.000000000000058620 ) ) ;
#11004=CARTESIAN_POINT ( 'NONE',  ( 18.83615802559801722, -32.14641817400232071, -6.999999999999950262 ) ) ;
#11009=DIRECTION ( 'NONE',  ( 6.505213034913038160E-19, 3.903127820947822896E-18, 1.000000000000000000 ) ) ;
#11015=ORIENTED_EDGE ( 'NONE', *, *, #9598, .F. ) ;
#11017=ORIENTED_EDGE ( 'NONE', *, *, #16463, .T. ) ;
#11018=VERTEX_POINT ( 'NONE', #9627 ) ;
#11019=EDGE_LOOP ( 'NONE', ( #8143, #2373, #20006, #9079 ) ) ;
#11023=ADVANCED_FACE ( 'NONE', ( #22125 ), #8142, .F. ) ;
#11026=CARTESIAN_POINT ( 'NONE',  ( -30.99230043872318063, 17.38334492574541557, -3.000000000000012879 ) ) ;
#11029=CARTESIAN_POINT ( 'NONE',  ( -31.67162468655980589, -14.67611967928950101, 3.000000000000002665 ) ) ;
#11032=ORIENTED_EDGE ( 'NONE', *, *, #4757, .F. ) ;
#11041=CARTESIAN_POINT ( 'NONE',  ( 2.775557561562891351E-14, -2.775557561562891351E-14, 2.999999999999999112 ) ) ;
#11042=VERTEX_POINT ( 'NONE', #6305 ) ;
#11044=AXIS2_PLACEMENT_3D ( 'NONE', #165, #22541, #14130 ) ;
#11045=ORIENTED_EDGE ( 'NONE', *, *, #7713, .T. ) ;
#11046=VERTEX_POINT ( 'NONE', #9412 ) ;
#11053=DIRECTION ( 'NONE',  ( 1.000000000000000000, 0.000000000000000000, 0.000000000000000000 ) ) ;
#11056=DIRECTION ( 'NONE',  ( -6.505213034913038160E-19, -3.903127820947822896E-18, -1.000000000000000000 ) ) ;
#11058=DIRECTION ( 'NONE',  ( 6.505213034913038160E-19, 3.903127820947822896E-18, 1.000000000000000000 ) ) ;
#11066=DIRECTION ( 'NONE',  ( 1.000000000000000000, 0.000000000000000000, 0.000000000000000000 ) ) ;
#11068=ORIENTED_EDGE ( 'NONE', *, *, #21533, .T. ) ;
#11070=CIRCLE ( 'NONE', #7773, 0.9999999999999974465 ) ;
#11072=DIRECTION ( 'NONE',  ( 1.000000000000000000, 1.208970125616053321E-17, 0.000000000000000000 ) ) ;
#11074=AXIS2_PLACEMENT_3D ( 'NONE', #4296, #14591, #5544 ) ;
#11075=CARTESIAN_POINT ( 'NONE',  ( 31.92986134326233838, -18.22261011550285659, -1.999999999999998224 ) ) ;
#11079=DIRECTION ( 'NONE',  ( 6.505213034913038160E-19, 3.903127820947822896E-18, 1.000000000000000000 ) ) ;
#11086=DIRECTION ( 'NONE',  ( -6.505213034913038160E-19, -3.903127820947822896E-18, -1.000000000000000000 ) ) ;
#11091=DIRECTION ( 'NONE',  ( -6.505213034913038160E-19, -3.903127820947822896E-18, -1.000000000000000000 ) ) ;
#11096=CARTESIAN_POINT ( 'NONE',  ( 34.10919265018095103, -11.98978967046217825, 2.932969818539045370 ) ) ;
#11100=EDGE_LOOP ( 'NONE', ( #9928, #10134, #19004, #12845 ) ) ;
#11105=ORIENTED_EDGE ( 'NONE', *, *, #1725, .F. ) ;
#11109=ORIENTED_EDGE ( 'NONE', *, *, #9270, .T. ) ;
#11117=CARTESIAN_POINT ( 'NONE',  ( 3.330669073875469621E-13, -1.110223024625156540E-13, -2.999999999999971578 ) ) ;
#11118=CARTESIAN_POINT ( 'NONE',  ( -1.011722470947959973, -35.51751788033354984, -2.999999999999999112 ) ) ;
#11122=TOROIDAL_SURFACE ( 'NONE', #15870, 34.90673715956759082, 8.750000000000000000 ) ;
#11124=VERTEX_POINT ( 'NONE', #19948 ) ;
#11125=VERTEX_POINT ( 'NONE', #11229 ) ;
#11128=VERTEX_POINT ( 'NONE', #16950 ) ;
#11132=AXIS2_PLACEMENT_3D ( 'NONE', #8730, #8611, #19391 ) ;
#11134=EDGE_LOOP ( 'NONE', ( #12502, #7047, #14066, #9878, #7159, #4884 ) ) ;
#11135=DIRECTION ( 'NONE',  ( 6.505213034913038160E-19, 3.903127820947822896E-18, 1.000000000000000000 ) ) ;
#11138=EDGE_CURVE ( 'NONE', #2407, #6416, #17953, .T. ) ;
#11140=LINE ( 'NONE', #3719, #7583 ) ;
#11141=CYLINDRICAL_SURFACE ( 'NONE', #955, 31.50000000000000711 ) ;
#11144=ORIENTED_EDGE ( 'NONE', *, *, #4527, .F. ) ;
#11147=ORIENTED_EDGE ( 'NONE', *, *, #10291, .F. ) ;
#11155=CARTESIAN_POINT ( 'NONE',  ( -22.28024240313504478, -22.26748298433264850, -2.999999999999999112 ) ) ;
#11160=ORIENTED_EDGE ( 'NONE', *, *, #520, .F. ) ;
#11163=EDGE_CURVE ( 'NONE', #13942, #12412, #3479, .T. ) ;
#11165=EDGE_LOOP ( 'NONE', ( #2104, #19928, #7479, #1165 ) ) ;
#11170=DIRECTION ( 'NONE',  ( -1.000000000000000000, -1.208970125616044077E-17, 0.000000000000000000 ) ) ;
#11176=CARTESIAN_POINT ( 'NONE',  ( 27.56232195404084706, -21.41958700883264655, -2.999999999999954259 ) ) ;
#11178=DIRECTION ( 'NONE',  ( -4.718764931986839378E-35, 3.903127820947822896E-18, 1.000000000000000000 ) ) ;
#11180=CARTESIAN_POINT ( 'NONE',  ( -22.97438720605733664, 22.98755168577407204, -2.999999999999971578 ) ) ;
#11182=EDGE_LOOP ( 'NONE', ( #6710, #4979, #4937, #11032 ) ) ;
#11183=ORIENTED_EDGE ( 'NONE', *, *, #21500, .T. ) ;
#11184=VECTOR ( 'NONE', #12574, 1000.000000000000000 ) ;
#11189=EDGE_CURVE ( 'NONE', #4971, #2350, #5976, .T. ) ;
#11192=VECTOR ( 'NONE', #12451, 1000.000000000000000 ) ;
#11194=CARTESIAN_POINT ( 'NONE',  ( 3.330669073875469621E-13, -1.110223024625156540E-13, -2.999999999999971578 ) ) ;
#11196=CARTESIAN_POINT ( 'NONE',  ( 14.30873905802362778, 28.06260833510296138, 2.999999999999995559 ) ) ;
#11204=CIRCLE ( 'NONE', #11586, 1.000000000000000888 ) ;
#11205=EDGE_LOOP ( 'NONE', ( #15523, #17104, #17722, #20020, #1529, #9568 ) ) ;
#11206=ORIENTED_EDGE ( 'NONE', *, *, #19592, .T. ) ;
#11208=DIRECTION ( 'NONE',  ( -1.000000000000000000, 0.000000000000000000, 0.000000000000000000 ) ) ;
#11212=LINE ( 'NONE', #16601, #12945 ) ;
#11217=CARTESIAN_POINT ( 'NONE',  ( -17.86915608785671949, 27.01645732367855146, 2.999999999999995559 ) ) ;
#11219=DIRECTION ( 'NONE',  ( -1.000000000000000000, -1.208970125616060101E-17, 6.505213034913038160E-19 ) ) ;
#11220=FACE_OUTER_BOUND ( 'NONE', #12641, .T. ) ;
#11226=DIRECTION ( 'NONE',  ( -6.505213034913038160E-19, -3.903127820947822896E-18, -1.000000000000000000 ) ) ;
#11228=FACE_BOUND ( 'NONE', #15344, .T. ) ;
#11229=CARTESIAN_POINT ( 'NONE',  ( 12.00937115242667375, 34.74700806321082069, -2.800654218530485018 ) ) ;
#11231=ORIENTED_EDGE ( 'NONE', *, *, #14388, .T. ) ;
#11234=CARTESIAN_POINT ( 'NONE',  ( -11.93972437435557232, -29.14949368109881433, 3.000000000000023537 ) ) ;
#11238=CIRCLE ( 'NONE', #1366, 1.000000000000000888 ) ;
#11251=ORIENTED_EDGE ( 'NONE', *, *, #16707, .T. ) ;
#11252=CARTESIAN_POINT ( 'NONE',  ( 1.110223024625156540E-13, -5.551115123125782702E-14, -6.999999999999950262 ) ) ;
#11254=ORIENTED_EDGE ( 'NONE', *, *, #19789, .F. ) ;
#11259=CARTESIAN_POINT ( 'NONE',  ( 33.51030287062386748, 15.12081897056644131, -1.999999999999970468 ) ) ;
#11265=EDGE_LOOP ( 'NONE', ( #4960, #910, #7460, #13719 ) ) ;
#11273=EDGE_CURVE ( 'NONE', #2292, #4146, #6193, .T. ) ;
#11274=EDGE_CURVE ( 'NONE', #1434, #4151, #11830, .T. ) ;
#11278=ORIENTED_EDGE ( 'NONE', *, *, #9270, .F. ) ;
#11279=ORIENTED_EDGE ( 'NONE', *, *, #16812, .T. ) ;
#11280=DIRECTION ( 'NONE',  ( -6.505213034913038160E-19, -3.903127820947822896E-18, -1.000000000000000000 ) ) ;
#11284=CARTESIAN_POINT ( 'NONE',  ( -27.64365646977254443, -17.09029715894946833, 3.000000000000012879 ) ) ;
#11286=VERTEX_POINT ( 'NONE', #10403 ) ;
#11290=ORIENTED_EDGE ( 'NONE', *, *, #21092, .T. ) ;
#11291=CARTESIAN_POINT ( 'NONE',  ( -17.38334492574528767, -30.99230043872344709, -2.999999999999998224 ) ) ;
#11296=EDGE_CURVE ( 'NONE', #5732, #5053, #14747, .T. ) ;
#11298=CIRCLE ( 'NONE', #5447, 0.9999999999999991118 ) ;
#11299=DIRECTION ( 'NONE',  ( -6.505213034913038160E-19, -3.903127820947822896E-18, -1.000000000000000000 ) ) ;
#11305=ORIENTED_EDGE ( 'NONE', *, *, #20514, .F. ) ;
#11307=VERTEX_POINT ( 'NONE', #17970 ) ;
#11310=EDGE_CURVE ( 'NONE', #22272, #4064, #20617, .T. ) ;
#11320=FACE_OUTER_BOUND ( 'NONE', #10609, .T. ) ;
#11325=CARTESIAN_POINT ( 'NONE',  ( -24.41514043009178181, -26.50842683089757301, -6.999999999999999112 ) ) ;
#11327=CARTESIAN_POINT ( 'NONE',  ( 6.070730550690961458, 31.88709182564675260, -6.999999999999950262 ) ) ;
#11328=ORIENTED_EDGE ( 'NONE', *, *, #6804, .F. ) ;
#11329=FACE_BOUND ( 'NONE', #21016, .T. ) ;
#11332=DIRECTION ( 'NONE',  ( 1.000000000000000000, 0.000000000000000000, 0.000000000000000000 ) ) ;
#11349=CARTESIAN_POINT ( 'NONE',  ( 6.955395936297148474, 34.84717828836173226, -3.000000000000006217 ) ) ;
#11350=DIRECTION ( 'NONE',  ( -4.718764931986839378E-35, 3.903127820947822896E-18, 1.000000000000000000 ) ) ;
#11353=VERTEX_POINT ( 'NONE', #1835 ) ;
#11354=CIRCLE ( 'NONE', #19430, 3.000000000000000888 ) ;
#11358=ORIENTED_EDGE ( 'NONE', *, *, #13226, .F. ) ;
#11367=VERTEX_POINT ( 'NONE', #9154 ) ;
#11369=CYLINDRICAL_SURFACE ( 'NONE', #6140, 19.11328065563151668 ) ;
#11370=ORIENTED_EDGE ( 'NONE', *, *, #21564, .F. ) ;
#11371=DIRECTION ( 'NONE',  ( -6.505213034913038160E-19, -3.903127820947822896E-18, -1.000000000000000000 ) ) ;
#11372=CARTESIAN_POINT ( 'NONE',  ( 2.220446049250313081E-13, -8.326672684688674053E-14, 2.800654218530498785 ) ) ;
#11380=VERTEX_POINT ( 'NONE', #12685 ) ;
#11382=FACE_OUTER_BOUND ( 'NONE', #10498, .T. ) ;
#11383=DIRECTION ( 'NONE',  ( 6.505213034913038160E-19, 3.903127820947822896E-18, 1.000000000000000000 ) ) ;
#11393=AXIS2_PLACEMENT_3D ( 'NONE', #13955, #8263, #15350 ) ;
#11395=DIRECTION ( 'NONE',  ( 6.505213034913038160E-19, 3.903127820947822896E-18, 1.000000000000000000 ) ) ;
#11396=EDGE_CURVE ( 'NONE', #10145, #19815, #18541, .T. ) ;
#11397=VERTEX_POINT ( 'NONE', #4349 ) ;
#11398=DIRECTION ( 'NONE',  ( 1.000000000000000000, 0.000000000000000000, 0.000000000000000000 ) ) ;
#11402=ORIENTED_EDGE ( 'NONE', *, *, #15894, .T. ) ;
#11406=EDGE_CURVE ( 'NONE', #14574, #8378, #7890, .T. ) ;
#11411=EDGE_CURVE ( 'NONE', #19815, #2292, #11852, .T. ) ;
#11417=CARTESIAN_POINT ( 'NONE',  ( 2.220446049250313081E-13, -8.326672684688674053E-14, 2.800654218530498785 ) ) ;
#11418=EDGE_CURVE ( 'NONE', #5124, #18180, #1440, .T. ) ;
#11419=FACE_OUTER_BOUND ( 'NONE', #14791, .T. ) ;
#11420=CARTESIAN_POINT ( 'NONE',  ( -6.070730550690850436, -31.88709182564697286, 3.000000000000023537 ) ) ;
#11429=CARTESIAN_POINT ( 'NONE',  ( 24.24871130596442725, 14.00000000000009592, -2.999999999999947153 ) ) ;
#11440=EDGE_CURVE ( 'NONE', #15106, #12187, #17703, .T. ) ;
#11442=AXIS2_PLACEMENT_3D ( 'NONE', #7508, #17932, #3848 ) ;
#11446=FACE_OUTER_BOUND ( 'NONE', #9833, .T. ) ;
#11447=ORIENTED_EDGE ( 'NONE', *, *, #6730, .T. ) ;
#11449=CARTESIAN_POINT ( 'NONE',  ( -29.33526866242075570, 22.15900668633760517, -1.999999999999977573 ) ) ;
#11454=CIRCLE ( 'NONE', #10348, 19.11328065563151668 ) ;
#11456=ORIENTED_EDGE ( 'NONE', *, *, #13735, .T. ) ;
#11458=CYLINDRICAL_SURFACE ( 'NONE', #22118, 31.50000000000001421 ) ;
#11460=VECTOR ( 'NONE', #12515, 1000.000000000000000 ) ;
#11475=VERTEX_POINT ( 'NONE', #5938 ) ;
#11482=CARTESIAN_POINT ( 'NONE',  ( -15.02862401740787135, -32.75570538720795355, -2.999999999999971578 ) ) ;
#11484=ORIENTED_EDGE ( 'NONE', *, *, #8839, .T. ) ;
#11487=EDGE_CURVE ( 'NONE', #2202, #20150, #19902, .T. ) ;
#11494=ORIENTED_EDGE ( 'NONE', *, *, #11640, .T. ) ;
#11496=FACE_OUTER_BOUND ( 'NONE', #18730, .T. ) ;
#11500=AXIS2_PLACEMENT_3D ( 'NONE', #13029, #18321, #14862 ) ;
#11501=CARTESIAN_POINT ( 'NONE',  ( 35.79662727779903264, -4.171001175319571708, 2.999999999999999112 ) ) ;
#11507=ORIENTED_EDGE ( 'NONE', *, *, #5139, .F. ) ;
#11512=FACE_OUTER_BOUND ( 'NONE', #20109, .T. ) ;
#11513=CARTESIAN_POINT ( 'NONE',  ( 4.918774254215884767, -31.11359284679388182, -7.000000000000006217 ) ) ;
#11516=CARTESIAN_POINT ( 'NONE',  ( -27.56232195404058416, 21.41958700883256483, 2.999999999999995559 ) ) ;
#11525=LINE ( 'NONE', #13113, #5343 ) ;
#11528=EDGE_CURVE ( 'NONE', #4626, #19154, #20628, .T. ) ;
#11529=ORIENTED_EDGE ( 'NONE', *, *, #2612, .T. ) ;
#11535=DIRECTION ( 'NONE',  ( -6.505213034913038160E-19, -3.903127820947822896E-18, -1.000000000000000000 ) ) ;
#11541=FACE_OUTER_BOUND ( 'NONE', #3510, .T. ) ;
#11542=CARTESIAN_POINT ( 'NONE',  ( 32.89708536800427652, 15.00428685838163823, 2.932460736555811742 ) ) ;
#11545=EDGE_LOOP ( 'NONE', ( #16672, #13613, #7819, #20523 ) ) ;
#11546=LINE ( 'NONE', #22097, #7316 ) ;
#11551=CIRCLE ( 'NONE', #6795, 19.11328065563150957 ) ;
#11553=EDGE_CURVE ( 'NONE', #8231, #19408, #12418, .T. ) ;
#11556=VECTOR ( 'NONE', #15364, 1000.000000000000000 ) ;
#11557=AXIS2_PLACEMENT_3D ( 'NONE', #11194, #19912, #21870 ) ;
#11561=DIRECTION ( 'NONE',  ( 1.000000000000000000, 2.269002777743560714E-17, 0.000000000000000000 ) ) ;
#11563=AXIS2_PLACEMENT_3D ( 'NONE', #7876, #6496, #21866 ) ;
#11564=AXIS2_PLACEMENT_3D ( 'NONE', #10345, #18968, #3278 ) ;
#11571=DIRECTION ( 'NONE',  ( 1.000000000000000000, 1.208970125616063182E-17, 0.000000000000000000 ) ) ;
#11573=VECTOR ( 'NONE', #22685, 1000.000000000000000 ) ;
#11575=ORIENTED_EDGE ( 'NONE', *, *, #3874, .T. ) ;
#11576=CARTESIAN_POINT ( 'NONE',  ( -14.76298474240489433, -28.95348479018575105, -2.999999999999971578 ) ) ;
#11577=CARTESIAN_POINT ( 'NONE',  ( -19.99999999999982236, -5.551115123125782702E-14, 3.000000000000016431 ) ) ;
#11583=DIRECTION ( 'NONE',  ( -1.000000000000000000, -1.208970125616046080E-17, 6.505213034913038160E-19 ) ) ;
#11586=AXIS2_PLACEMENT_3D ( 'NONE', #11180, #9693, #13119 ) ;
#11589=EDGE_CURVE ( 'NONE', #16318, #4151, #19316, .T. ) ;
#11590=ORIENTED_EDGE ( 'NONE', *, *, #17744, .F. ) ;
#11593=CARTESIAN_POINT ( 'NONE',  ( 21.65063509461090518, 12.49999999999978861, 2.999999999999995559 ) ) ;
#11596=ORIENTED_EDGE ( 'NONE', *, *, #182, .T. ) ;
#11597=CARTESIAN_POINT ( 'NONE',  ( -15.12081897056651059, 33.51030287062345536, 2.800654218530485018 ) ) ;
#11599=VERTEX_POINT ( 'NONE', #15626 ) ;
#11603=CARTESIAN_POINT ( 'NONE',  ( -34.88850421923971368, 1.128083539116031542, -2.999999999999981792 ) ) ;
#11607=EDGE_CURVE ( 'NONE', #22470, #3870, #15450, .T. ) ;
#11608=EDGE_LOOP ( 'NONE', ( #15168, #9261, #4828, #15573 ) ) ;
#11609=DIRECTION ( 'NONE',  ( -6.505213034913038160E-19, -3.903127820947822896E-18, -1.000000000000000000 ) ) ;
#11611=ORIENTED_EDGE ( 'NONE', *, *, #22321, .T. ) ;
#11616=AXIS2_PLACEMENT_3D ( 'NONE', #13183, #4742, #12964 ) ;
#11626=CARTESIAN_POINT ( 'NONE',  ( 32.40961249803578426, -2.422192751864060689, -6.999999999999950262 ) ) ;
#11627=CIRCLE ( 'NONE', #21510, 1.000000000000000888 ) ;
#11633=CIRCLE ( 'NONE', #2494, 1.000000000000000888 ) ;
#11634=DIRECTION ( 'NONE',  ( -1.000000000000000000, -1.208970125616060101E-17, 6.505213034913038160E-19 ) ) ;
#11637=CIRCLE ( 'NONE', #7253, 0.9999999999999991118 ) ;
#11640=EDGE_CURVE ( 'NONE', #12190, #17561, #15509, .T. ) ;
#11642=ORIENTED_EDGE ( 'NONE', *, *, #13505, .F. ) ;
#11644=TOROIDAL_SURFACE ( 'NONE', #17862, 34.90673715956759082, 8.750000000000000000 ) ;
#11647=DIRECTION ( 'NONE',  ( 6.505213034913038160E-19, 3.903127820947822896E-18, 1.000000000000000000 ) ) ;
#11650=EDGE_CURVE ( 'NONE', #586, #7599, #1569, .T. ) ;
#11651=CIRCLE ( 'NONE', #4357, 0.9999999999999974465 ) ;
#11652=VERTEX_POINT ( 'NONE', #13791 ) ;
#11654=DIRECTION ( 'NONE',  ( 1.000000000000000000, 0.000000000000000000, 0.000000000000000000 ) ) ;
#11655=DIRECTION ( 'NONE',  ( -1.000000000000000000, 0.000000000000000000, 0.000000000000000000 ) ) ;
#11657=B_SPLINE_CURVE_WITH_KNOTS ( 'NONE', 3,
 ( #10927, #21361, #2228, #7612 ),
 .UNSPECIFIED., .F., .F.,
 ( 4, 4 ),
 ( 9.545285769941151703E-07, 0.001900595205834767999 ),
 .UNSPECIFIED. ) ;
#11661=DIRECTION ( 'NONE',  ( 6.505213034913038160E-19, 3.903127820947822896E-18, 1.000000000000000000 ) ) ;
#11662=DIRECTION ( 'NONE',  ( 1.000000000000000000, 1.208970125616063028E-17, 0.000000000000000000 ) ) ;
#11663=EDGE_CURVE ( 'NONE', #4123, #22470, #10688, .T. ) ;
#11675=DIRECTION ( 'NONE',  ( 1.000000000000000000, 0.000000000000000000, 0.000000000000000000 ) ) ;
#11679=DIRECTION ( 'NONE',  ( 6.505213034913038160E-19, 3.903127820947822896E-18, 1.000000000000000000 ) ) ;
#11681=LINE ( 'NONE', #14656, #22626 ) ;
#11683=CARTESIAN_POINT ( 'NONE',  ( 16.99647590252675755, 30.48934413892762052, 3.000000000000019984 ) ) ;
#11684=MECHANICAL_DESIGN_GEOMETRIC_PRESENTATION_REPRESENTATION('',(#15333),#19382);
#11686=DIRECTION ( 'NONE',  ( 6.505213034913038160E-19, 3.903127820947822896E-18, 1.000000000000000000 ) ) ;
#11687=CARTESIAN_POINT ( 'NONE',  ( 1.942890293094023946E-13, -8.326672684688674053E-14, 5.000000000000000888 ) ) ;
#11689=ADVANCED_FACE ( 'NONE', ( #7150 ), #14121, .T. ) ;
#11694=CARTESIAN_POINT ( 'NONE',  ( 3.330669073875469621E-13, -1.110223024625156540E-13, -2.999999999999971578 ) ) ;
#11695=ADVANCED_FACE ( 'NONE', ( #17924 ), #18028, .T. ) ;
#11698=ORIENTED_EDGE ( 'NONE', *, *, #18376, .T. ) ;
#11699=ADVANCED_FACE ( 'NONE', ( #14467 ), #14356, .T. ) ;
#11703=CARTESIAN_POINT ( 'NONE',  ( -7.463862311150981199, -35.99819890246952525, 2.800654218530485018 ) ) ;
#11708=CARTESIAN_POINT ( 'NONE',  ( 18.22261011550294185, 31.92986134326200443, 2.800654218530481465 ) ) ;
#11713=VECTOR ( 'NONE', #18216, 1000.000000000000000 ) ;
#11717=VERTEX_POINT ( 'NONE', #19991 ) ;
#11725=EDGE_CURVE ( 'NONE', #14674, #18815, #15084, .T. ) ;
#11728=CIRCLE ( 'NONE', #10612, 31.50000000000001421 ) ;
#11732=DIRECTION ( 'NONE',  ( 6.505213034913038160E-19, 3.903127820947822896E-18, 1.000000000000000000 ) ) ;
#11734=ORIENTED_EDGE ( 'NONE', *, *, #17490, .F. ) ;
#11735=CARTESIAN_POINT ( 'NONE',  ( -28.73472116836718371, 21.94328778841591898, 2.932969818539058693 ) ) ;
#11736=DIRECTION ( 'NONE',  ( -6.505213034913038160E-19, -3.903127820947822896E-18, -1.000000000000000000 ) ) ;
#11737=ORIENTED_EDGE ( 'NONE', *, *, #18168, .T. ) ;
#11738=DIRECTION ( 'NONE',  ( -6.505213034913038160E-19, -3.903127820947822896E-18, -1.000000000000000000 ) ) ;
#11742=AXIS2_PLACEMENT_3D ( 'NONE', #6698, #11736, #21959 ) ;
#11744=CARTESIAN_POINT ( 'NONE',  ( -8.550503583141688679, 23.49231551964756193, -2.999999999999971578 ) ) ;
#11746=CIRCLE ( 'NONE', #20159, 36.76383501243555685 ) ;
#11747=EDGE_CURVE ( 'NONE', #12202, #11599, #11657, .T. ) ;
#11748=DIRECTION ( 'NONE',  ( -6.505213034913038160E-19, -3.903127820947822896E-18, -1.000000000000000000 ) ) ;
#11755=CARTESIAN_POINT ( 'NONE',  ( -4.025500340002458266, 36.54278193890269932, -2.000000000000005329 ) ) ;
#11764=EDGE_CURVE ( 'NONE', #5453, #19435, #5894, .T. ) ;
#11766=DIRECTION ( 'NONE',  ( 6.505213034913038160E-19, 3.903127820947822896E-18, 1.000000000000000000 ) ) ;
#11770=DIRECTION ( 'NONE',  ( 6.505213034913038160E-19, 3.903127820947822896E-18, 1.000000000000000000 ) ) ;
#11775=DIRECTION ( 'NONE',  ( 1.000000000000000000, 0.000000000000000000, 0.000000000000000000 ) ) ;
#11776=EDGE_LOOP ( 'NONE', ( #18034, #17973, #18343, #17697 ) ) ;
#11780=DIRECTION ( 'NONE',  ( 6.505213034913038160E-19, 3.903127820947822896E-18, 1.000000000000000000 ) ) ;
#11782=LINE ( 'NONE', #20288, #16656 ) ;
#11783=EDGE_CURVE ( 'NONE', #17600, #10809, #10547, .T. ) ;
#11791=ORIENTED_EDGE ( 'NONE', *, *, #3879, .F. ) ;
#11794=CARTESIAN_POINT ( 'NONE',  ( -5.093313992686365310, -32.09841355226039639, -2.999999999999995559 ) ) ;
#11795=AXIS2_PLACEMENT_3D ( 'NONE', #5119, #3391, #22656 ) ;
#11796=EDGE_CURVE ( 'NONE', #21043, #17505, #744, .T. ) ;
#11798=ORIENTED_EDGE ( 'NONE', *, *, #14377, .T. ) ;
#11802=LINE ( 'NONE', #8485, #18729 ) ;
#11803=DIRECTION ( 'NONE',  ( 6.505213034913038160E-19, 3.903127820947822896E-18, 1.000000000000000000 ) ) ;
#11809=ORIENTED_EDGE ( 'NONE', *, *, #3177, .T. ) ;
#11811=DIRECTION ( 'NONE',  ( -6.505213034913038160E-19, -3.903127820947822896E-18, -1.000000000000000000 ) ) ;
#11815=CARTESIAN_POINT ( 'NONE',  ( 32.14641817400198676, 18.83615802559776498, -7.000000000000006217 ) ) ;
#11817=DIRECTION ( 'NONE',  ( 1.000000000000000000, 0.000000000000000000, 0.000000000000000000 ) ) ;
#11818=ORIENTED_EDGE ( 'NONE', *, *, #10152, .T. ) ;
#11823=ORIENTED_EDGE ( 'NONE', *, *, #16254, .T. ) ;
#11826=DIRECTION ( 'NONE',  ( -1.000000000000000000, -1.208970125616060717E-17, 0.000000000000000000 ) ) ;
#11830=CIRCLE ( 'NONE', #8545, 36.76383501243555685 ) ;
#11834=VERTEX_POINT ( 'NONE', #15030 ) ;
#11835=EDGE_CURVE ( 'NONE', #13942, #17988, #12177, .T. ) ;
#11837=ADVANCED_FACE ( 'NONE', ( #11382 ), #19499, .T. ) ;
#11838=ORIENTED_EDGE ( 'NONE', *, *, #10822, .F. ) ;
#11842=VERTEX_POINT ( 'NONE', #14805 ) ;
#11846=FACE_OUTER_BOUND ( 'NONE', #14644, .T. ) ;
#11848=VECTOR ( 'NONE', #12075, 1000.000000000000000 ) ;
#11852=CIRCLE ( 'NONE', #4909, 19.11328065563150957 ) ;
#11855=FACE_OUTER_BOUND ( 'NONE', #18537, .T. ) ;
#11856=CIRCLE ( 'NONE', #9288, 34.90673715956759082 ) ;
#11859=ORIENTED_EDGE ( 'NONE', *, *, #20183, .F. ) ;
#11860=ORIENTED_EDGE ( 'NONE', *, *, #19592, .F. ) ;
#11869=EDGE_CURVE ( 'NONE', #13841, #17930, #8874, .T. ) ;
#11873=CARTESIAN_POINT ( 'NONE',  ( -26.79308242454879618, -16.56444186175107092, -7.000000000000006217 ) ) ;
#11879=CARTESIAN_POINT ( 'NONE',  ( 29.33526866242100439, -22.15900668633777215, -2.800654218530429507 ) ) ;
#11881=CARTESIAN_POINT ( 'NONE',  ( 3.330669073875469621E-13, -1.110223024625156540E-13, -2.999999999999971578 ) ) ;
#11886=AXIS2_PLACEMENT_3D ( 'NONE', #14946, #11748, #20574 ) ;
#11887=VERTEX_POINT ( 'NONE', #7956 ) ;
#11891=CARTESIAN_POINT ( 'NONE',  ( 14.76298474240547698, 28.95348479018558407, 2.999999999999995559 ) ) ;
#11892=ORIENTED_EDGE ( 'NONE', *, *, #1051, .T. ) ;
#11894=CARTESIAN_POINT ( 'NONE',  ( -28.06260833510291874, 14.30873905802329560, -2.999999999999981792 ) ) ;
#11901=ORIENTED_EDGE ( 'NONE', *, *, #21397, .T. ) ;
#11908=DIRECTION ( 'NONE',  ( -1.000000000000000000, -1.208970125616060101E-17, 6.505213034913038160E-19 ) ) ;
#11909=CARTESIAN_POINT ( 'NONE',  ( 21.00948735876886886, 24.79619811426206510, -2.999999999999971578 ) ) ;
#11911=EDGE_CURVE ( 'NONE', #18993, #17804, #4144, .T. ) ;
#11920=CARTESIAN_POINT ( 'NONE',  ( 1.387778780781445676E-13, -22.00000000000021316, 3.000000000000002665 ) ) ;
#11921=AXIS2_PLACEMENT_3D ( 'NONE', #16713, #7772, #21647 ) ;
#11922=DIRECTION ( 'NONE',  ( -1.000000000000000000, 1.061893299983986855E-14, 0.000000000000000000 ) ) ;
#11927=CARTESIAN_POINT ( 'NONE',  ( 2.775557561562891351E-14, 2.775557561562891351E-14, 5.750000000000001776 ) ) ;
#11930=DIRECTION ( 'NONE',  ( 1.000000000000000000, 0.000000000000000000, 0.000000000000000000 ) ) ;
#11933=FACE_OUTER_BOUND ( 'NONE', #15148, .T. ) ;
#11939=AXIS2_PLACEMENT_3D ( 'NONE', #18596, #1625, #3119 ) ;
#11945=DIRECTION ( 'NONE',  ( 1.000000000000000000, 0.000000000000000000, 0.000000000000000000 ) ) ;
#11948=EDGE_CURVE ( 'NONE', #9581, #7786, #7434, .T. ) ;
#11949=AXIS2_PLACEMENT_3D ( 'NONE', #4549, #18177, #16680 ) ;
#11951=ORIENTED_EDGE ( 'NONE', *, *, #6852, .T. ) ;
#11952=ORIENTED_EDGE ( 'NONE', *, *, #18575, .F. ) ;
#11953=EDGE_LOOP ( 'NONE', ( #7349, #2289, #7424, #9485 ) ) ;
#11954=AXIS2_PLACEMENT_3D ( 'NONE', #5376, #10734, #3438 ) ;
#11955=ORIENTED_EDGE ( 'NONE', *, *, #8922, .T. ) ;
#11956=LINE ( 'NONE', #18956, #3736 ) ;
#11958=DIRECTION ( 'NONE',  ( 6.505213034913038160E-19, 3.903127820947822896E-18, 1.000000000000000000 ) ) ;
#11961=CARTESIAN_POINT ( 'NONE',  ( 1.110223024625156540E-13, -27.99999999999999645, -2.999999999999971578 ) ) ;
#11964=AXIS2_PLACEMENT_3D ( 'NONE', #4110, #2387, #5828 ) ;
#11966=EDGE_CURVE ( 'NONE', #20409, #1875, #9667, .T. ) ;
#11971=DIRECTION ( 'NONE',  ( -6.505213034913038160E-19, -3.903127820947822896E-18, -1.000000000000000000 ) ) ;
#11977=DIRECTION ( 'NONE',  ( -1.000000000000000000, -1.208970125616060101E-17, 6.505213034913038160E-19 ) ) ;
#11980=AXIS2_PLACEMENT_3D ( 'NONE', #13083, #9554, #16429 ) ;
#11984=ORIENTED_EDGE ( 'NONE', *, *, #19694, .F. ) ;
#11986=DIRECTION ( 'NONE',  ( 6.505213034913038160E-19, 3.903127820947822896E-18, 1.000000000000000000 ) ) ;
#11989=EDGE_CURVE ( 'NONE', #15903, #13430, #7034, .T. ) ;
#11990=DIRECTION ( 'NONE',  ( 6.505213034913038160E-19, 3.903127820947822896E-18, 1.000000000000000000 ) ) ;
#11996=DIRECTION ( 'NONE',  ( 6.505213034913038160E-19, 3.903127820947822896E-18, 1.000000000000000000 ) ) ;
#11999=ORIENTED_EDGE ( 'NONE', *, *, #8128, .F. ) ;
#12004=AXIS2_PLACEMENT_3D ( 'NONE', #18500, #10008, #20228 ) ;
#12005=AXIS2_PLACEMENT_3D ( 'NONE', #20397, #14870, #22231 ) ;
#12006=DIRECTION ( 'NONE',  ( -1.000000000000000000, 0.000000000000000000, 0.000000000000000000 ) ) ;
#12007=CARTESIAN_POINT ( 'NONE',  ( -21.05198877411799785, 30.13956425491218383, -1.999999999999977573 ) ) ;
#12010=CIRCLE ( 'NONE', #14560, 1.000000000000000888 ) ;
#12014=ORIENTED_EDGE ( 'NONE', *, *, #22469, .F. ) ;
#12017=EDGE_CURVE ( 'NONE', #14229, #16393, #12198, .T. ) ;
#12020=AXIS2_PLACEMENT_3D ( 'NONE', #22172, #20564, #11398 ) ;
#12034=CARTESIAN_POINT ( 'NONE',  ( -12.31876324338254669, -30.07487443287981677, -6.999999999999950262 ) ) ;
#12035=FACE_OUTER_BOUND ( 'NONE', #1109, .T. ) ;
#12037=EDGE_CURVE ( 'NONE', #4151, #20949, #15208, .T. ) ;
#12039=ORIENTED_EDGE ( 'NONE', *, *, #17951, .T. ) ;
#12061=DIRECTION ( 'NONE',  ( 6.505213034913038160E-19, 3.903127820947822896E-18, 1.000000000000000000 ) ) ;
#12062=EDGE_CURVE ( 'NONE', #312, #11717, #20254, .T. ) ;
#12065=CARTESIAN_POINT ( 'NONE',  ( 24.43377932785621809, -26.64693883069189795, -2.933296326616325889 ) ) ;
#12068=B_SPLINE_CURVE_WITH_KNOTS ( 'NONE', 3,
 ( #907, #11096, #21769, #5842 ),
 .UNSPECIFIED., .F., .F.,
 ( 4, 4 ),
 ( 9.715086407578286637E-07, 0.001929643240672447449 ),
 .UNSPECIFIED. ) ;
#12069=ORIENTED_EDGE ( 'NONE', *, *, #6055, .F. ) ;
#12073=VERTEX_POINT ( 'NONE', #17212 ) ;
#12074=CARTESIAN_POINT ( 'NONE',  ( 30.13956425491259949, 21.05198877411795877, -2.800654218530485018 ) ) ;
#12075=DIRECTION ( 'NONE',  ( 6.505213034913038160E-19, 3.903127820947822896E-18, 1.000000000000000000 ) ) ;
#12076=CIRCLE ( 'NONE', #8413, 19.11328065563152379 ) ;
#12078=EDGE_LOOP ( 'NONE', ( #19689, #17072, #447, #12802 ) ) ;
#12081=ORIENTED_EDGE ( 'NONE', *, *, #14436, .F. ) ;
#12085=AXIS2_PLACEMENT_3D ( 'NONE', #18175, #3983, #12659 ) ;
#12087=ORIENTED_EDGE ( 'NONE', *, *, #7613, .T. ) ;
#12088=CARTESIAN_POINT ( 'NONE',  ( -9.576564013118904484, 26.31139338200535960, -4.999999999999948486 ) ) ;
#12092=DIRECTION ( 'NONE',  ( 6.505213034913038160E-19, 3.903127820947822896E-18, 1.000000000000000000 ) ) ;
#12096=EDGE_CURVE ( 'NONE', #4210, #7013, #5979, .T. ) ;
#12100=CARTESIAN_POINT ( 'NONE',  ( -12.00937115242649256, -34.74700806321106938, -2.800654218530485018 ) ) ;
#12101=CARTESIAN_POINT ( 'NONE',  ( -19.05255888325750746, 10.99999999999970512, 3.000000000000006217 ) ) ;
#12107=DIRECTION ( 'NONE',  ( 6.505213034913038160E-19, 3.903127820947822896E-18, 1.000000000000000000 ) ) ;
#12108=DIRECTION ( 'NONE',  ( -1.000000000000000000, -1.208970125616063798E-17, 0.000000000000000000 ) ) ;
#12110=ORIENTED_EDGE ( 'NONE', *, *, #10724, .T. ) ;
#12116=CARTESIAN_POINT ( 'NONE',  ( -17.66631876130905709, 31.41173278719225337, -2.999999999999971578 ) ) ;
#12118=VERTEX_POINT ( 'NONE', #128 ) ;
#12119=ORIENTED_EDGE ( 'NONE', *, *, #20577, .F. ) ;
#12121=EDGE_LOOP ( 'NONE', ( #2928, #19034, #2664, #20414 ) ) ;
#12130=CARTESIAN_POINT ( 'NONE',  ( 10.70799354677379256, -35.16985127952393242, 2.800654218530485018 ) ) ;
#12137=EDGE_CURVE ( 'NONE', #18451, #767, #22088, .T. ) ;
#12140=CARTESIAN_POINT ( 'NONE',  ( 34.65667543218853552, 4.170748987303296573, -2.999999999999975131 ) ) ;
#12147=EDGE_LOOP ( 'NONE', ( #9092, #13483, #22181, #19222 ) ) ;
#12149=CARTESIAN_POINT ( 'NONE',  ( -24.41514043009200563, -26.50842683089765828, 3.000000000000002665 ) ) ;
#12156=VERTEX_POINT ( 'NONE', #16156 ) ;
#12157=CARTESIAN_POINT ( 'NONE',  ( 4.025500340002624355, -36.54278193890314697, 2.800654218530485018 ) ) ;
#12160=CIRCLE ( 'NONE', #9963, 36.76383501243555685 ) ;
#12161=CARTESIAN_POINT ( 'NONE',  ( -0.6841746959067307454, -36.75746821813308429, 2.800654218530485018 ) ) ;
#12162=ADVANCED_FACE ( 'NONE', ( #14435 ), #4524, .T. ) ;
#12163=DIRECTION ( 'NONE',  ( -1.000000000000000000, -1.208970125616077665E-17, 0.000000000000000000 ) ) ;
#12165=ORIENTED_EDGE ( 'NONE', *, *, #16979, .T. ) ;
#12171=CARTESIAN_POINT ( 'NONE',  ( -20.36304159388362223, -24.03323817228478276, 3.000000000000023537 ) ) ;
#12172=CARTESIAN_POINT ( 'NONE',  ( 3.330669073875469621E-13, -1.110223024625156540E-13, -2.999999999999971578 ) ) ;
#12174=VECTOR ( 'NONE', #19296, 1000.000000000000000 ) ;
#12176=EDGE_LOOP ( 'NONE', ( #45, #22166, #16814, #12178 ) ) ;
#12177=CIRCLE ( 'NONE', #5241, 36.76383501243555685 ) ;
#12178=ORIENTED_EDGE ( 'NONE', *, *, #20146, .F. ) ;
#12179=DIRECTION ( 'NONE',  ( -6.505213034913038160E-19, -3.903127820947822896E-18, -1.000000000000000000 ) ) ;
#12184=VERTEX_POINT ( 'NONE', #3807 ) ;
#12185=DIRECTION ( 'NONE',  ( -1.000000000000000000, -1.208970125616046080E-17, 6.505213034913038160E-19 ) ) ;
#12187=VERTEX_POINT ( 'NONE', #10770 ) ;
#12188=CARTESIAN_POINT ( 'NONE',  ( 34.84300730320200046, -6.953913411054821303, 3.000000000000056399 ) ) ;
#12190=VERTEX_POINT ( 'NONE', #10653 ) ;
#12193=CYLINDRICAL_SURFACE ( 'NONE', #21572, 1.000000000000000888 ) ;
#12195=CARTESIAN_POINT ( 'NONE',  ( 35.33352588067123179, 7.094908322882953478, 3.000000000000009770 ) ) ;
#12198=CIRCLE ( 'NONE', #16214, 1.000000000000000888 ) ;
#12200=EDGE_CURVE ( 'NONE', #20409, #2631, #2083, .T. ) ;
#12201=ORIENTED_EDGE ( 'NONE', *, *, #21092, .F. ) ;
#12202=VERTEX_POINT ( 'NONE', #9075 ) ;
#12204=ORIENTED_EDGE ( 'NONE', *, *, #11747, .T. ) ;
#12205=DIRECTION ( 'NONE',  ( 6.505213034913038160E-19, 3.903127820947822896E-18, 1.000000000000000000 ) ) ;
#12212=CARTESIAN_POINT ( 'NONE',  ( 8.646032897229233072, -31.21605069118116305, 2.999999999999995559 ) ) ;
#12216=DIRECTION ( 'NONE',  ( 6.505213034913038160E-19, 3.903127820947822896E-18, 1.000000000000000000 ) ) ;
#12219=AXIS2_PLACEMENT_3D ( 'NONE', #11041, #2345, #16433 ) ;
#12221=VERTEX_POINT ( 'NONE', #5626 ) ;
#12226=EDGE_CURVE ( 'NONE', #13393, #15368, #20600, .T. ) ;
#12234=FACE_OUTER_BOUND ( 'NONE', #842, .T. ) ;
#12242=EDGE_LOOP ( 'NONE', ( #10693, #11484, #10112, #6627 ) ) ;
#12248=CARTESIAN_POINT ( 'NONE',  ( 25.58633464742662866, 23.74488952252781715, 2.999999999999999112 ) ) ;
#12252=AXIS2_PLACEMENT_3D ( 'NONE', #12913, #14858, #19713 ) ;
#12256=ORIENTED_EDGE ( 'NONE', *, *, #6377, .T. ) ;
#12262=CARTESIAN_POINT ( 'NONE',  ( 5.093313992686421265, 32.09841355225992743, 3.000000000000023537 ) ) ;
#12264=LINE ( 'NONE', #18813, #2522 ) ;
#12271=CYLINDRICAL_SURFACE ( 'NONE', #11964, 19.11328065563152023 ) ;
#12274=CARTESIAN_POINT ( 'NONE',  ( -26.50842683089750551, 24.41514043009185286, 2.999999999999995559 ) ) ;
#12276=ORIENTED_EDGE ( 'NONE', *, *, #9164, .F. ) ;
#12280=AXIS2_PLACEMENT_3D ( 'NONE', #19615, #7464, #21109 ) ;
#12283=B_SPLINE_CURVE_WITH_KNOTS ( 'NONE', 3,
 ( #14023, #12433, #3748, #21270 ),
 .UNSPECIFIED., .F., .F.,
 ( 4, 4 ),
 ( 9.545285770168743104E-07, 0.001900595205834662181 ),
 .UNSPECIFIED. ) ;
#12286=EDGE_CURVE ( 'NONE', #14574, #16276, #2691, .T. ) ;
#12288=EDGE_CURVE ( 'NONE', #5141, #12838, #2616, .T. ) ;
#12294=DIRECTION ( 'NONE',  ( 6.505213034913038160E-19, 3.903127820947822896E-18, 1.000000000000000000 ) ) ;
#12300=CIRCLE ( 'NONE', #11939, 0.9999999999999974465 ) ;
#12303=CARTESIAN_POINT ( 'NONE',  ( 2.220446049250313081E-13, -2.498001805406602216E-13, -6.859353255829918616 ) ) ;
#12305=CARTESIAN_POINT ( 'NONE',  ( 34.24928931925769149, -6.742883674876604339, 3.000000000000002665 ) ) ;
#12314=ORIENTED_EDGE ( 'NONE', *, *, #11273, .F. ) ;
#12317=ORIENTED_EDGE ( 'NONE', *, *, #18317, .F. ) ;
#12318=CARTESIAN_POINT ( 'NONE',  ( 2.775557561562891351E-14, -2.775557561562891351E-14, 2.999999999999999112 ) ) ;
#12319=AXIS2_PLACEMENT_3D ( 'NONE', #5432, #7598, #17678 ) ;
#12320=DIRECTION ( 'NONE',  ( 1.000000000000000000, 1.208970125616063798E-17, 0.000000000000000000 ) ) ;
#12321=CARTESIAN_POINT ( 'NONE',  ( 2.422192751863949667, 32.40961249803550714, 2.999999999999995559 ) ) ;
#12323=ORIENTED_EDGE ( 'NONE', *, *, #443, .F. ) ;
#12324=CARTESIAN_POINT ( 'NONE',  ( -4.171001175319349663, -35.79662727779881237, -6.999999999999964473 ) ) ;
#12327=DIRECTION ( 'NONE',  ( 6.505213034913038160E-19, 3.903127820947822896E-18, 1.000000000000000000 ) ) ;
#12333=EDGE_CURVE ( 'NONE', #10809, #1823, #11856, .T. ) ;
#12339=ORIENTED_EDGE ( 'NONE', *, *, #13548, .T. ) ;
#12342=VERTEX_POINT ( 'NONE', #20072 ) ;
#12343=CARTESIAN_POINT ( 'NONE',  ( -7.197698565811593951, -35.43359966464136335, 2.932460736555830394 ) ) ;
#12349=EDGE_CURVE ( 'NONE', #19349, #12202, #20182, .T. ) ;
#12355=AXIS2_PLACEMENT_3D ( 'NONE', #8670, #9931, #4899 ) ;
#12357=CARTESIAN_POINT ( 'NONE',  ( 24.73600648735124707, -27.19760187735892387, -2.800654218530457484 ) ) ;
#12360=ORIENTED_EDGE ( 'NONE', *, *, #4345, .F. ) ;
#12361=CARTESIAN_POINT ( 'NONE',  ( 4.080045426412798548, -32.20238537491815123, -6.999999999999950262 ) ) ;
#12366=VECTOR ( 'NONE', #10918, 1000.000000000000000 ) ;
#12367=EDGE_CURVE ( 'NONE', #2168, #11124, #10781, .T. ) ;
#12369=AXIS2_PLACEMENT_3D ( 'NONE', #12844, #22670, #15641 ) ;
#12370=VERTEX_POINT ( 'NONE', #15000 ) ;
#12373=CARTESIAN_POINT ( 'NONE',  ( 12.00937115242667375, 34.74700806321082069, -2.800654218530485018 ) ) ;
#12374=ORIENTED_EDGE ( 'NONE', *, *, #17048, .T. ) ;
#12377=ORIENTED_EDGE ( 'NONE', *, *, #9333, .T. ) ;
#12378=EDGE_CURVE ( 'NONE', #8183, #12492, #22106, .T. ) ;
#12380=EDGE_CURVE ( 'NONE', #6233, #18161, #4181, .T. ) ;
#12381=DIRECTION ( 'NONE',  ( -6.505213034913038160E-19, -3.903127820947822896E-18, -1.000000000000000000 ) ) ;
#12385=DIRECTION ( 'NONE',  ( 6.505213034913038160E-19, 3.903127820947822896E-18, 1.000000000000000000 ) ) ;
#12386=CARTESIAN_POINT ( 'NONE',  ( -15.12081897056651059, 33.51030287062345536, 2.800654218530485018 ) ) ;
#12391=ADVANCED_FACE ( 'NONE', ( #13167 ), #17691, .T. ) ;
#12392=CARTESIAN_POINT ( 'NONE',  ( 0.6841746959068695233, 36.75746821813305587, 2.800654218530485018 ) ) ;
#12394=ORIENTED_EDGE ( 'NONE', *, *, #19548, .T. ) ;
#12395=ORIENTED_EDGE ( 'NONE', *, *, #1020, .T. ) ;
#12403=VERTEX_POINT ( 'NONE', #18572 ) ;
#12404=DIRECTION ( 'NONE',  ( -6.505213034913038160E-19, -3.903127820947822896E-18, -1.000000000000000000 ) ) ;
#12406=ORIENTED_EDGE ( 'NONE', *, *, #11911, .F. ) ;
#12407=( GEOMETRIC_REPRESENTATION_CONTEXT ( 3 ) GLOBAL_UNCERTAINTY_ASSIGNED_CONTEXT ( ( #20214 ) ) GLOBAL_UNIT_ASSIGNED_CONTEXT ( ( #17560, #16060, #14564 ) ) REPRESENTATION_CONTEXT ( 'NONE', 'WORKASPACE' ) );
#12408=EDGE_CURVE ( 'NONE', #20709, #6187, #19174, .T. ) ;
#12412=VERTEX_POINT ( 'NONE', #2886 ) ;
#12418=LINE ( 'NONE', #5221, #13610 ) ;
#12422=ORIENTED_EDGE ( 'NONE', *, *, #5104, .T. ) ;
#12428=CARTESIAN_POINT ( 'NONE',  ( -34.65667543218827973, -4.170748987303380062, 3.000000000000002665 ) ) ;
#12433=CARTESIAN_POINT ( 'NONE',  ( 32.89319786336257323, 15.00354810072174239, -2.933296326616365857 ) ) ;
#12438=AXIS2_PLACEMENT_3D ( 'NONE', #21311, #7560, #14538 ) ;
#12441=EDGE_CURVE ( 'NONE', #14737, #586, #9528, .T. ) ;
#12444=ORIENTED_EDGE ( 'NONE', *, *, #15293, .T. ) ;
#12445=B_SPLINE_CURVE_WITH_KNOTS ( 'NONE', 3,
 ( #20922, #17692, #14240, #12522 ),
 .UNSPECIFIED., .F., .F.,
 ( 4, 4 ),
 ( 9.715086411272982943E-07, 0.001929643240672562375 ),
 .UNSPECIFIED. ) ;
#12451=DIRECTION ( 'NONE',  ( 6.505213034913038160E-19, 3.903127820947822896E-18, 1.000000000000000000 ) ) ;
#12453=CARTESIAN_POINT ( 'NONE',  ( 30.99230043872329432, -17.38334492574589163, -2.999999999999984901 ) ) ;
#12454=CARTESIAN_POINT ( 'NONE',  ( 22.28024240313511584, 22.26748298433259166, -2.999999999999999112 ) ) ;
#12460=ORIENTED_EDGE ( 'NONE', *, *, #19649, .F. ) ;
#12463=B_SPLINE_CURVE_WITH_KNOTS ( 'NONE', 3,
 ( #448, #2177, #10993, #2286 ),
 .UNSPECIFIED., .F., .F.,
 ( 4, 4 ),
 ( 0.001875451646903029826, 0.003761979286331461510 ),
 .UNSPECIFIED. ) ;
#12464=CARTESIAN_POINT ( 'NONE',  ( -20.06142356895407275, 29.33203831401573325, 3.000000000000061284 ) ) ;
#12466=ADVANCED_FACE ( 'NONE', ( #12035 ), #13608, .T. ) ;
#12468=ORIENTED_EDGE ( 'NONE', *, *, #1237, .F. ) ;
#12470=EDGE_CURVE ( 'NONE', #7599, #7962, #18474, .T. ) ;
#12471=DIRECTION ( 'NONE',  ( -1.000000000000000000, -1.208970125616060717E-17, 0.000000000000000000 ) ) ;
#12480=DIRECTION ( 'NONE',  ( 6.505213034913038160E-19, 3.903127820947822896E-18, 1.000000000000000000 ) ) ;
#12489=CARTESIAN_POINT ( 'NONE',  ( 3.608224830031758756E-13, -2.775557561562891351E-14, -4.999999999999997335 ) ) ;
#12490=EDGE_CURVE ( 'NONE', #20847, #5303, #20620, .T. ) ;
#12492=VERTEX_POINT ( 'NONE', #3341 ) ;
#12493=VERTEX_POINT ( 'NONE', #1379 ) ;
#12498=CARTESIAN_POINT ( 'NONE',  ( -25.58633464742629471, -23.74488952252781715, -2.999999999999975131 ) ) ;
#12501=DIRECTION ( 'NONE',  ( -1.000000000000000000, 0.000000000000000000, 0.000000000000000000 ) ) ;
#12502=ORIENTED_EDGE ( 'NONE', *, *, #12665, .T. ) ;
#12504=CARTESIAN_POINT ( 'NONE',  ( -31.47226199422867410, 17.79229176513279498, -2.933296326616379623 ) ) ;
#12508=CARTESIAN_POINT ( 'NONE',  ( -15.62726112422596714, -28.45046755804883531, -2.999999999999971578 ) ) ;
#12510=DIRECTION ( 'NONE',  ( -1.000000000000000000, -1.266830946243004623E-16, -4.336808689942002810E-19 ) ) ;
#12512=CARTESIAN_POINT ( 'NONE',  ( -19.05255888325749325, 10.99999999999967670, -2.999999999999975131 ) ) ;
#12515=DIRECTION ( 'NONE',  ( 6.505213034913038160E-19, 3.903127820947822896E-18, 1.000000000000000000 ) ) ;
#12516=CYLINDRICAL_SURFACE ( 'NONE', #4301, 19.11328065563151668 ) ;
#12519=DIRECTION ( 'NONE',  ( 6.505213034913038160E-19, 3.903127820947822896E-18, 1.000000000000000000 ) ) ;
#12521=VECTOR ( 'NONE', #12205, 1000.000000000000000 ) ;
#12522=CARTESIAN_POINT ( 'NONE',  ( 27.56232195404068008, -21.41958700883258970, 2.999999999999995559 ) ) ;
#12524=EDGE_CURVE ( 'NONE', #13542, #2593, #17324, .T. ) ;
#12525=AXIS2_PLACEMENT_3D ( 'NONE', #17352, #22532, #6827 ) ;
#12526=VERTEX_POINT ( 'NONE', #12248 ) ;
#12528=ORIENTED_EDGE ( 'NONE', *, *, #13320, .T. ) ;
#12533=CARTESIAN_POINT ( 'NONE',  ( -4.918774254215691144, 31.11359284679368642, 3.000000000000023537 ) ) ;
#12534=EDGE_CURVE ( 'NONE', #8936, #17952, #13646, .T. ) ;
#12538=VECTOR ( 'NONE', #11647, 1000.000000000000000 ) ;
#12540=DIRECTION ( 'NONE',  ( 6.505213034913038160E-19, 3.903127820947822896E-18, 1.000000000000000000 ) ) ;
#12542=PRODUCT_DEFINITION_CONTEXT ( 'detailed design', #16165, 'design' ) ;
#12551=ORIENTED_EDGE ( 'NONE', *, *, #13949, .T. ) ;
#12554=AXIS2_PLACEMENT_3D ( 'NONE', #11694, #1046, #9964 ) ;
#12557=EDGE_CURVE ( 'NONE', #15629, #22134, #6722, .T. ) ;
#12560=AXIS2_PLACEMENT_3D ( 'NONE', #2944, #20688, #11977 ) ;
#12561=CARTESIAN_POINT ( 'NONE',  ( 20.05817253550624457, -29.32895111104220831, -2.999999999999998224 ) ) ;
#12566=CARTESIAN_POINT ( 'NONE',  ( 2.775557561562891351E-14, -2.775557561562891351E-14, 2.999999999999999112 ) ) ;
#12568=ORIENTED_EDGE ( 'NONE', *, *, #5444, .F. ) ;
#12571=DIRECTION ( 'NONE',  ( -1.000000000000000000, 2.831715466623964737E-14, 0.000000000000000000 ) ) ;
#12574=DIRECTION ( 'NONE',  ( 6.505213034913038160E-19, 3.903127820947822896E-18, 1.000000000000000000 ) ) ;
#12583=CARTESIAN_POINT ( 'NONE',  ( -31.11359284679367221, -4.918774254215884767, 2.999999999999995559 ) ) ;
#12592=CARTESIAN_POINT ( 'NONE',  ( -11.31876324338271544, -30.07487443287981677, -2.999999999999995559 ) ) ;
#12593=ORIENTED_EDGE ( 'NONE', *, *, #13949, .F. ) ;
#12598=EDGE_CURVE ( 'NONE', #12403, #19421, #14384, .T. ) ;
#12599=VERTEX_POINT ( 'NONE', #20971 ) ;
#12601=CARTESIAN_POINT ( 'NONE',  ( 24.75236754129178607, 27.84804035626017793, -7.000000000000006217 ) ) ;
#12606=ORIENTED_EDGE ( 'NONE', *, *, #73, .T. ) ;
#12607=CIRCLE ( 'NONE', #7892, 22.00000000000000000 ) ;
#12610=VERTEX_POINT ( 'NONE', #9266 ) ;
#12613=CARTESIAN_POINT ( 'NONE',  ( -32.10132595304128245, -5.074925817841801745, -6.999999999999999112 ) ) ;
#12616=DIRECTION ( 'NONE',  ( -6.505213034913038160E-19, -3.903127820947822896E-18, -1.000000000000000000 ) ) ;
#12621=DIRECTION ( 'NONE',  ( 6.505213034913038160E-19, 3.903127820947822896E-18, 1.000000000000000000 ) ) ;
#12632=ORIENTED_EDGE ( 'NONE', *, *, #3453, .F. ) ;
#12639=EDGE_LOOP ( 'NONE', ( #20338, #21885, #2401, #161, #16858, #6666 ) ) ;
#12641=EDGE_LOOP ( 'NONE', ( #4850, #11402, #13543, #8923 ) ) ;
#12646=CIRCLE ( 'NONE', #16326, 19.11328065563151668 ) ;
#12650=LINE ( 'NONE', #755, #9478 ) ;
#12659=DIRECTION ( 'NONE',  ( 1.000000000000000000, 0.000000000000000000, 0.000000000000000000 ) ) ;
#12660=CIRCLE ( 'NONE', #15591, 18.00000000000000000 ) ;
#12662=AXIS2_PLACEMENT_3D ( 'NONE', #19166, #24, #21105 ) ;
#12665=EDGE_CURVE ( 'NONE', #16393, #10093, #7548, .T. ) ;
#12666=VERTEX_POINT ( 'NONE', #101 ) ;
#12673=CARTESIAN_POINT ( 'NONE',  ( -34.24928931925764886, 6.742883674876548383, 2.999999999999999112 ) ) ;
#12678=DIRECTION ( 'NONE',  ( 1.000000000000000000, 0.000000000000000000, 0.000000000000000000 ) ) ;
#12683=CARTESIAN_POINT ( 'NONE',  ( -22.15900668633775794, -29.33526866242097597, 2.800654218530509443 ) ) ;
#12685=CARTESIAN_POINT ( 'NONE',  ( -27.19760187735852242, -24.73600648735135721, 2.800654218530492123 ) ) ;
#12688=EDGE_CURVE ( 'NONE', #13845, #3722, #211, .T. ) ;
#12689=ORIENTED_EDGE ( 'NONE', *, *, #1448, .F. ) ;
#12690=FACE_OUTER_BOUND ( 'NONE', #8334, .T. ) ;
#12695=ADVANCED_FACE ( 'NONE', ( #4019 ), #12805, .F. ) ;
#12697=CARTESIAN_POINT ( 'NONE',  ( -16.99647590252638452, -30.48934413892778750, 2.999999999999999112 ) ) ;
#12699=AXIS2_PLACEMENT_3D ( 'NONE', #5876, #14330, #5759 ) ;
#12701=VECTOR ( 'NONE', #13284, 1000.000000000000000 ) ;
#12703=DIRECTION ( 'NONE',  ( -1.000000000000000000, -1.208970125616060101E-17, 6.505213034913038160E-19 ) ) ;
#12706=CYLINDRICAL_SURFACE ( 'NONE', #18771, 36.76383501243555685 ) ;
#12708=ORIENTED_EDGE ( 'NONE', *, *, #8400, .T. ) ;
#12709=CARTESIAN_POINT ( 'NONE',  ( -22.15900668633775794, -29.33526866242097597, 2.800654218530509443 ) ) ;
#12713=CARTESIAN_POINT ( 'NONE',  ( -34.74700806321097701, 12.00937115242647835, -2.000000000000001776 ) ) ;
#12716=CARTESIAN_POINT ( 'NONE',  ( -1.128083539116253586, -34.88850421923977763, -2.999999999999971578 ) ) ;
#12720=CIRCLE ( 'NONE', #660, 31.50000000000000711 ) ;
#12723=CIRCLE ( 'NONE', #21525, 36.76383501243555685 ) ;
#12724=AXIS2_PLACEMENT_3D ( 'NONE', #4587, #6530, #2645 ) ;
#12728=ORIENTED_EDGE ( 'NONE', *, *, #16769, .F. ) ;
#12733=EDGE_LOOP ( 'NONE', ( #11447, #10025, #19904, #1554 ) ) ;
#12734=CARTESIAN_POINT ( 'NONE',  ( -0.6841746959065087008, -36.75746821813308429, -2.000000000000005329 ) ) ;
#12740=CARTESIAN_POINT ( 'NONE',  ( 21.65063509461093005, 12.50000000000006750, -5.000000000000004441 ) ) ;
#12741=ORIENTED_EDGE ( 'NONE', *, *, #20125, .T. ) ;
#12742=CARTESIAN_POINT ( 'NONE',  ( 19.59430950039339692, -28.88846368933353759, 3.000000000000023537 ) ) ;
#12746=AXIS2_PLACEMENT_3D ( 'NONE', #19760, #18020, #18259 ) ;
#12748=ORIENTED_EDGE ( 'NONE', *, *, #3032, .T. ) ;
#12750=EDGE_LOOP ( 'NONE', ( #22679, #1050, #16270, #5752 ) ) ;
#12755=ORIENTED_EDGE ( 'NONE', *, *, #975, .T. ) ;
#12761=ORIENTED_EDGE ( 'NONE', *, *, #10562, .F. ) ;
#12762=ORIENTED_EDGE ( 'NONE', *, *, #13900, .T. ) ;
#12763=EDGE_CURVE ( 'NONE', #1089, #17558, #10080, .T. ) ;
#12769=ORIENTED_EDGE ( 'NONE', *, *, #5252, .F. ) ;
#12771=ADVANCED_FACE ( 'NONE', ( #9721 ), #21996, .T. ) ;
#12776=CARTESIAN_POINT ( 'NONE',  ( -31.57187188083505802, -7.711478842616608986, -2.999999999999971578 ) ) ;
#12783=ORIENTED_EDGE ( 'NONE', *, *, #18581, .T. ) ;
#12787=ORIENTED_EDGE ( 'NONE', *, *, #8470, .T. ) ;
#12788=DIRECTION ( 'NONE',  ( -6.505213034913038160E-19, -3.903127820947822896E-18, -1.000000000000000000 ) ) ;
#12789=DIRECTION ( 'NONE',  ( 6.505213034913038160E-19, 3.903127820947822896E-18, 1.000000000000000000 ) ) ;
#12793=CYLINDRICAL_SURFACE ( 'NONE', #10782, 2.999999999999999112 ) ;
#12794=VECTOR ( 'NONE', #14679, 1000.000000000000000 ) ;
#12797=DIRECTION ( 'NONE',  ( 6.505213034913038160E-19, 3.903127820947822896E-18, 1.000000000000000000 ) ) ;
#12799=CARTESIAN_POINT ( 'NONE',  ( -24.75236754129155159, -27.84804035626051189, 2.999999999999995559 ) ) ;
#12800=VERTEX_POINT ( 'NONE', #18424 ) ;
#12801=CARTESIAN_POINT ( 'NONE',  ( 2.220446049250313081E-13, -8.326672684688674053E-14, 2.800654218530498785 ) ) ;
#12802=ORIENTED_EDGE ( 'NONE', *, *, #8958, .F. ) ;
#12804=LINE ( 'NONE', #901, #1263 ) ;
#12805=CYLINDRICAL_SURFACE ( 'NONE', #5714, 1.000000000000000888 ) ;
#12806=EDGE_CURVE ( 'NONE', #11307, #8182, #14093, .T. ) ;
#12809=FACE_OUTER_BOUND ( 'NONE', #7730, .T. ) ;
#12811=EDGE_CURVE ( 'NONE', #9285, #4760, #22567, .T. ) ;
#12812=ORIENTED_EDGE ( 'NONE', *, *, #11310, .T. ) ;
#12814=CYLINDRICAL_SURFACE ( 'NONE', #372, 19.11328065563152379 ) ;
#12815=FACE_OUTER_BOUND ( 'NONE', #13056, .T. ) ;
#12826=ORIENTED_EDGE ( 'NONE', *, *, #218, .F. ) ;
#12827=CARTESIAN_POINT ( 'NONE',  ( -21.97438720605730822, 22.98755168577401520, -7.000000000000006217 ) ) ;
#12834=ORIENTED_EDGE ( 'NONE', *, *, #9469, .T. ) ;
#12835=ORIENTED_EDGE ( 'NONE', *, *, #7385, .F. ) ;
#12837=EDGE_CURVE ( 'NONE', #5871, #20053, #14310, .T. ) ;
#12838=VERTEX_POINT ( 'NONE', #20046 ) ;
#12839=LINE ( 'NONE', #12734, #5917 ) ;
#12844=CARTESIAN_POINT ( 'NONE',  ( 31.57187188083543461, 7.711478842616415363, 2.999999999999995559 ) ) ;
#12845=ORIENTED_EDGE ( 'NONE', *, *, #14145, .F. ) ;
#12846=CARTESIAN_POINT ( 'NONE',  ( -20.55056392469585802, 29.75120097320018431, -2.932164912090549969 ) ) ;
#12849=CARTESIAN_POINT ( 'NONE',  ( 2.220446049250313081E-13, -8.326672684688674053E-14, 2.800654218530498785 ) ) ;
#12852=CARTESIAN_POINT ( 'NONE',  ( 28.45046755804903071, -15.62726112422607727, 3.000000000000023537 ) ) ;
#12861=LINE ( 'NONE', #6002, #16738 ) ;
#12868=ORIENTED_EDGE ( 'NONE', *, *, #3743, .T. ) ;
#12871=CARTESIAN_POINT ( 'NONE',  ( 4.025500340002707844, -36.54278193890314697, -2.800654218530457484 ) ) ;
#12874=EDGE_LOOP ( 'NONE', ( #14599, #1573, #9975, #14647 ) ) ;
#12875=DIRECTION ( 'NONE',  ( 6.505213034913038160E-19, 3.903127820947822896E-18, 1.000000000000000000 ) ) ;
#12877=VERTEX_POINT ( 'NONE', #2859 ) ;
#12889=DIRECTION ( 'NONE',  ( 1.000000000000000000, 0.000000000000000000, 0.000000000000000000 ) ) ;
#12893=CIRCLE ( 'NONE', #4879, 19.11328065563152379 ) ;
#12894=CARTESIAN_POINT ( 'NONE',  ( 2.775557561562891351E-14, -2.775557561562891351E-14, 2.999999999999999112 ) ) ;
#12902=CARTESIAN_POINT ( 'NONE',  ( -9.708269511265104512, 33.52953626616034200, -2.999999999999978240 ) ) ;
#12903=ORIENTED_EDGE ( 'NONE', *, *, #9741, .T. ) ;
#12906=CARTESIAN_POINT ( 'NONE',  ( -14.93538271375420479, -34.13396246814581758, -2.999999999999999112 ) ) ;
#12913=CARTESIAN_POINT ( 'NONE',  ( 2.422192751864033156, 32.40961249803547872, -6.999999999999950262 ) ) ;
#12914=DIRECTION ( 'NONE',  ( 6.505213034913038160E-19, 3.903127820947822896E-18, 1.000000000000000000 ) ) ;
#12916=AXIS2_PLACEMENT_3D ( 'NONE', #14557, #17775, #9184 ) ;
#12918=DIRECTION ( 'NONE',  ( -6.505213034913038160E-19, -3.903127820947822896E-18, -1.000000000000000000 ) ) ;
#12921=VERTEX_POINT ( 'NONE', #13363 ) ;
#12923=DIRECTION ( 'NONE',  ( 6.505213034913038160E-19, 3.903127820947822896E-18, 1.000000000000000000 ) ) ;
#12933=DIRECTION ( 'NONE',  ( 1.000000000000000000, 1.208970125616063798E-17, 0.000000000000000000 ) ) ;
#12934=ORIENTED_EDGE ( 'NONE', *, *, #3197, .F. ) ;
#12938=EDGE_CURVE ( 'NONE', #14924, #15891, #8648, .T. ) ;
#12939=CARTESIAN_POINT ( 'NONE',  ( 27.64365646977298852, 17.09029715894916279, -6.999999999999950262 ) ) ;
#12942=CARTESIAN_POINT ( 'NONE',  ( 1.110223024625156540E-13, -5.551115123125782702E-14, -6.999999999999950262 ) ) ;
#12945=VECTOR ( 'NONE', #16489, 1000.000000000000000 ) ;
#12946=EDGE_CURVE ( 'NONE', #14229, #2694, #8229, .T. ) ;
#12948=ORIENTED_EDGE ( 'NONE', *, *, #8436, .T. ) ;
#12954=FACE_OUTER_BOUND ( 'NONE', #3359, .T. ) ;
#12955=CARTESIAN_POINT ( 'NONE',  ( -23.65408649739124414, -22.22891329980541997, 3.000000000000023537 ) ) ;
#12958=AXIS2_PLACEMENT_3D ( 'NONE', #17811, #5897, #7614 ) ;
#12960=ORIENTED_EDGE ( 'NONE', *, *, #7866, .F. ) ;
#12962=CYLINDRICAL_SURFACE ( 'NONE', #17463, 0.9999999999999974465 ) ;
#12963=ORIENTED_EDGE ( 'NONE', *, *, #18338, .F. ) ;
#12964=DIRECTION ( 'NONE',  ( -1.000000000000000000, -1.208970125616077665E-17, 0.000000000000000000 ) ) ;
#12967=ORIENTED_EDGE ( 'NONE', *, *, #12557, .T. ) ;
#12973=ORIENTED_EDGE ( 'NONE', *, *, #13735, .F. ) ;
#12977=CIRCLE ( 'NONE', #5676, 34.90673715956759082 ) ;
#12980=CARTESIAN_POINT ( 'NONE',  ( -4.074925817841773323, 32.10132595304121850, -2.999999999999999112 ) ) ;
#12986=CARTESIAN_POINT ( 'NONE',  ( 25.58633464742662866, 23.74488952252781715, 2.999999999999999112 ) ) ;
#12989=FACE_OUTER_BOUND ( 'NONE', #9208, .T. ) ;
#12992=CARTESIAN_POINT ( 'NONE',  ( -17.79229176513264932, -31.47226199422894410, -2.933296326616350758 ) ) ;
#12996=CIRCLE ( 'NONE', #8985, 36.76383501243555685 ) ;
#12997=CARTESIAN_POINT ( 'NONE',  ( 24.73600648735135721, -27.19760187735867518, -2.000000000000005329 ) ) ;
#13003=ORIENTED_EDGE ( 'NONE', *, *, #19534, .T. ) ;
#13008=DIRECTION ( 'NONE',  ( -6.505213034913038160E-19, -3.903127820947822896E-18, -1.000000000000000000 ) ) ;
#13010=CARTESIAN_POINT ( 'NONE',  ( 32.27599279215780825, 14.85437171138566370, 3.000000000000047962 ) ) ;
#13014=AXIS2_PLACEMENT_3D ( 'NONE', #19610, #17769, #22615 ) ;
#13022=DIRECTION ( 'NONE',  ( 6.505213034913038160E-19, 3.903127820947822896E-18, 1.000000000000000000 ) ) ;
#13026=CARTESIAN_POINT ( 'NONE',  ( 33.52953626616048410, 9.708269511265299911, 2.999999999999995559 ) ) ;
#13027=ORIENTED_EDGE ( 'NONE', *, *, #21574, .T. ) ;
#13028=AXIS2_PLACEMENT_3D ( 'NONE', #1487, #5047, #18447 ) ;
#13029=CARTESIAN_POINT ( 'NONE',  ( 2.220446049250313081E-13, -2.498001805406602216E-13, -6.859353255829918616 ) ) ;
#13032=ADVANCED_FACE ( 'NONE', ( #17039 ), #10160, .F. ) ;
#13038=DIRECTION ( 'NONE',  ( 6.505213034913038160E-19, 3.903127820947822896E-18, 1.000000000000000000 ) ) ;
#13039=CARTESIAN_POINT ( 'NONE',  ( 2.775557561562891351E-14, -2.775557561562891351E-14, 2.999999999999995559 ) ) ;
#13046=DIRECTION ( 'NONE',  ( 6.505213034913038160E-19, 3.903127820947822896E-18, 1.000000000000000000 ) ) ;
#13052=DIRECTION ( 'NONE',  ( -6.505213034913038160E-19, -3.903127820947822896E-18, -1.000000000000000000 ) ) ;
#13053=EDGE_CURVE ( 'NONE', #767, #4765, #18179, .T. ) ;
#13056=EDGE_LOOP ( 'NONE', ( #5364, #19195, #16316, #7073 ) ) ;
#13058=EDGE_CURVE ( 'NONE', #3873, #4270, #10838, .T. ) ;
#13064=CARTESIAN_POINT ( 'NONE',  ( 31.92986134326233838, -18.22261011550282817, 2.800654218530512551 ) ) ;
#13065=CARTESIAN_POINT ( 'NONE',  ( 17.86915608785671949, -27.01645732367871489, 3.000000000000002665 ) ) ;
#13067=ORIENTED_EDGE ( 'NONE', *, *, #6955, .F. ) ;
#13068=CARTESIAN_POINT ( 'NONE',  ( -14.85437171138578094, 32.27599279215743167, 3.000000000000051958 ) ) ;
#13071=DIRECTION ( 'NONE',  ( -6.505213034913038160E-19, -3.903127820947822896E-18, -1.000000000000000000 ) ) ;
#13072=DIRECTION ( 'NONE',  ( -1.000000000000000000, -1.208970125616077665E-17, 0.000000000000000000 ) ) ;
#13073=CARTESIAN_POINT ( 'NONE',  ( 2.220446049250313081E-13, -8.326672684688674053E-14, 2.800654218530498785 ) ) ;
#13078=ORIENTED_EDGE ( 'NONE', *, *, #6945, .T. ) ;
#13083=CARTESIAN_POINT ( 'NONE',  ( 5.551115123125782702E-14, -1.387778780781445676E-13, -5.749999999999949374 ) ) ;
#13084=CIRCLE ( 'NONE', #3597, 19.11328065563152379 ) ;
#13093=ORIENTED_EDGE ( 'NONE', *, *, #20991, .T. ) ;
#13094=CIRCLE ( 'NONE', #6884, 28.00000000000000355 ) ;
#13099=AXIS2_PLACEMENT_3D ( 'NONE', #9906, #1093, #22060 ) ;
#13104=FACE_OUTER_BOUND ( 'NONE', #16285, .T. ) ;
#13109=ORIENTED_EDGE ( 'NONE', *, *, #12665, .F. ) ;
#13110=CARTESIAN_POINT ( 'NONE',  ( 5.551115123125782702E-14, -1.387778780781445676E-13, -5.749999999999949374 ) ) ;
#13112=CARTESIAN_POINT ( 'NONE',  ( 18.22261011550282817, 31.92986134326228509, -1.999999999999977573 ) ) ;
#13113=CARTESIAN_POINT ( 'NONE',  ( 3.053113317719180486E-13, -22.00000000000010303, -5.000000000000004441 ) ) ;
#13116=EDGE_CURVE ( 'NONE', #7486, #1368, #9132, .T. ) ;
#13119=DIRECTION ( 'NONE',  ( -1.000000000000000000, 0.000000000000000000, 0.000000000000000000 ) ) ;
#13122=VERTEX_POINT ( 'NONE', #3988 ) ;
#13128=CYLINDRICAL_SURFACE ( 'NONE', #8704, 0.9999999999999974465 ) ;
#13132=DIRECTION ( 'NONE',  ( -1.000000000000000000, 1.686330027304618723E-14, 0.000000000000000000 ) ) ;
#13140=DIRECTION ( 'NONE',  ( 6.505213034913038160E-19, 3.903127820947822896E-18, 1.000000000000000000 ) ) ;
#13142=CARTESIAN_POINT ( 'NONE',  ( 3.330669073875469621E-13, -1.110223024625156540E-13, -2.999999999999971578 ) ) ;
#13143=ORIENTED_EDGE ( 'NONE', *, *, #20991, .F. ) ;
#13146=ORIENTED_EDGE ( 'NONE', *, *, #18317, .T. ) ;
#13148=EDGE_CURVE ( 'NONE', #2570, #6570, #4268, .T. ) ;
#13158=DIRECTION ( 'NONE',  ( -6.505213034913038160E-19, -3.903127820947822896E-18, -1.000000000000000000 ) ) ;
#13167=FACE_OUTER_BOUND ( 'NONE', #10860, .T. ) ;
#13171=ORIENTED_EDGE ( 'NONE', *, *, #20274, .T. ) ;
#13181=DIRECTION ( 'NONE',  ( 1.000000000000000000, 0.000000000000000000, 0.000000000000000000 ) ) ;
#13182=EDGE_LOOP ( 'NONE', ( #16514, #281, #19233, #3078, #10879 ) ) ;
#13183=CARTESIAN_POINT ( 'NONE',  ( 2.220446049250313081E-13, -8.326672684688674053E-14, 2.800654218530498785 ) ) ;
#13195=EDGE_CURVE ( 'NONE', #17781, #18716, #17500, .T. ) ;
#13199=VERTEX_POINT ( 'NONE', #17610 ) ;
#13206=CARTESIAN_POINT ( 'NONE',  ( -7.463862311151203244, -35.99819890246958209, -2.000000000000001776 ) ) ;
#13207=ORIENTED_EDGE ( 'NONE', *, *, #18168, .F. ) ;
#13208=FACE_OUTER_BOUND ( 'NONE', #15613, .T. ) ;
#13212=EDGE_CURVE ( 'NONE', #3379, #13199, #15409, .T. ) ;
#13213=ORIENTED_EDGE ( 'NONE', *, *, #3966, .T. ) ;
#13214=DIRECTION ( 'NONE',  ( -1.000000000000000000, -1.208970125616046080E-17, 6.505213034913038160E-19 ) ) ;
#13215=CARTESIAN_POINT ( 'NONE',  ( 34.88850421923997658, -1.128083539116281342, -2.999999999999971578 ) ) ;
#13216=CARTESIAN_POINT ( 'NONE',  ( 3.330669073875469621E-13, -1.110223024625156540E-13, -2.999999999999971578 ) ) ;
#13223=DIRECTION ( 'NONE',  ( 6.505213034913038160E-19, 3.903127820947822896E-18, 1.000000000000000000 ) ) ;
#13225=ORIENTED_EDGE ( 'NONE', *, *, #16086, .F. ) ;
#13226=EDGE_CURVE ( 'NONE', #11834, #15811, #11204, .T. ) ;
#13236=ORIENTED_EDGE ( 'NONE', *, *, #8436, .F. ) ;
#13238=FACE_OUTER_BOUND ( 'NONE', #21099, .T. ) ;
#13239=DIRECTION ( 'NONE',  ( 1.000000000000000000, 0.000000000000000000, 0.000000000000000000 ) ) ;
#13241=DIRECTION ( 'NONE',  ( 1.000000000000000000, 1.208970125616063028E-17, 0.000000000000000000 ) ) ;
#13245=TOROIDAL_SURFACE ( 'NONE', #21320, 34.90673715956759082, 8.750000000000000000 ) ;
#13250=EDGE_CURVE ( 'NONE', #5266, #16827, #5008, .T. ) ;
#13252=VERTEX_POINT ( 'NONE', #20132 ) ;
#13254=CARTESIAN_POINT ( 'NONE',  ( 14.67611967928938910, -31.67162468656004037, 2.999999999999999112 ) ) ;
#13260=CARTESIAN_POINT ( 'NONE',  ( 2.220446049250313081E-13, -2.498001805406602216E-13, -6.859353255829918616 ) ) ;
#13263=CARTESIAN_POINT ( 'NONE',  ( 2.422192751863949667, 32.40961249803550714, -2.999999999999995559 ) ) ;
#13265=CARTESIAN_POINT ( 'NONE',  ( 21.66577056626875475, -3.820259908672518634, -4.999999999999969802 ) ) ;
#13268=EDGE_LOOP ( 'NONE', ( #5922, #16936, #1199, #13078 ) ) ;
#13269=CARTESIAN_POINT ( 'NONE',  ( -6.742883674876493316, -34.24928931925791176, -2.999999999999975131 ) ) ;
#13270=DIRECTION ( 'NONE',  ( -1.000000000000000000, -1.208970125616057944E-17, 0.000000000000000000 ) ) ;
#13275=AXIS2_PLACEMENT_3D ( 'NONE', #16737, #8038, #13270 ) ;
#13279=DIRECTION ( 'NONE',  ( 1.000000000000000000, 0.000000000000000000, 0.000000000000000000 ) ) ;
#13280=DIRECTION ( 'NONE',  ( 6.505213034913038160E-19, 3.903127820947822896E-18, 1.000000000000000000 ) ) ;
#13284=DIRECTION ( 'NONE',  ( 0.7071067811865524577, 9.238438721427047137E-17, -0.7071067811865426878 ) ) ;
#13287=EDGE_CURVE ( 'NONE', #22272, #22152, #2602, .T. ) ;
#13288=DIRECTION ( 'NONE',  ( -6.505213034913038160E-19, -3.903127820947822896E-18, -1.000000000000000000 ) ) ;
#13290=AXIS2_PLACEMENT_3D ( 'NONE', #3538, #3866, #1914 ) ;
#13292=EDGE_LOOP ( 'NONE', ( #5, #13869, #15719, #15279 ) ) ;
#13293=DIRECTION ( 'NONE',  ( -1.000000000000000000, 0.000000000000000000, 0.000000000000000000 ) ) ;
#13295=ORIENTED_EDGE ( 'NONE', *, *, #7298, .F. ) ;
#13296=DIRECTION ( 'NONE',  ( -1.000000000000000000, -1.208970125616063644E-17, 0.000000000000000000 ) ) ;
#13298=EDGE_CURVE ( 'NONE', #11475, #18373, #18904, .T. ) ;
#13299=ORIENTED_EDGE ( 'NONE', *, *, #13922, .F. ) ;
#13301=EDGE_CURVE ( 'NONE', #17574, #8936, #17437, .T. ) ;
#13306=CIRCLE ( 'NONE', #2358, 31.50000000000001421 ) ;
#13311=CIRCLE ( 'NONE', #5640, 36.76383501243555685 ) ;
#13317=CARTESIAN_POINT ( 'NONE',  ( -28.14364593009900517, 21.69710536060289741, 3.000000000000042633 ) ) ;
#13320=EDGE_CURVE ( 'NONE', #11887, #691, #14855, .T. ) ;
#13321=LINE ( 'NONE', #18504, #9536 ) ;
#13325=DIRECTION ( 'NONE',  ( -1.000000000000000000, -1.208970125616081209E-17, 0.000000000000000000 ) ) ;
#13329=EDGE_CURVE ( 'NONE', #19408, #1795, #7927, .T. ) ;
#13330=AXIS2_PLACEMENT_3D ( 'NONE', #16828, #5025, #12006 ) ;
#13332=CYLINDRICAL_SURFACE ( 'NONE', #11886, 36.76383501243555685 ) ;
#13341=DIRECTION ( 'NONE',  ( -6.505213034913038160E-19, -3.903127820947822896E-18, -1.000000000000000000 ) ) ;
#13343=EDGE_CURVE ( 'NONE', #4123, #18822, #4207, .T. ) ;
#13345=CYLINDRICAL_SURFACE ( 'NONE', #11563, 0.9999999999999991118 ) ;
#13346=VERTEX_POINT ( 'NONE', #6034 ) ;
#13359=DIRECTION ( 'NONE',  ( -1.000000000000000000, -1.208970125616077665E-17, 0.000000000000000000 ) ) ;
#13363=CARTESIAN_POINT ( 'NONE',  ( -7.524443153164889431, 20.67323765728973228, -2.999999999999978240 ) ) ;
#13365=TOROIDAL_SURFACE ( 'NONE', #17399, 34.90673715956759082, 8.750000000000000000 ) ;
#13367=AXIS2_PLACEMENT_3D ( 'NONE', #5137, #15650, #15414 ) ;
#13368=EDGE_CURVE ( 'NONE', #4700, #15473, #14503, .T. ) ;
#13372=VECTOR ( 'NONE', #9574, 1000.000000000000000 ) ;
#13376=CARTESIAN_POINT ( 'NONE',  ( -24.73600648735095575, 27.19760187735845136, -2.800654218530457484 ) ) ;
#13385=FACE_BOUND ( 'NONE', #21964, .T. ) ;
#13392=CIRCLE ( 'NONE', #12662, 1.000000000000000888 ) ;
#13393=VERTEX_POINT ( 'NONE', #12852 ) ;
#13400=DIRECTION ( 'NONE',  ( -1.000000000000000000, -1.208970125616063644E-17, 0.000000000000000000 ) ) ;
#13403=ORIENTED_EDGE ( 'NONE', *, *, #1866, .F. ) ;
#13404=CYLINDRICAL_SURFACE ( 'NONE', #17529, 31.50000000000000711 ) ;
#13405=DIRECTION ( 'NONE',  ( 1.000000000000000000, 2.269002777743560714E-17, 0.000000000000000000 ) ) ;
#13407=DIRECTION ( 'NONE',  ( -1.000000000000000000, -1.208970125616063644E-17, 0.000000000000000000 ) ) ;
#13408=EDGE_CURVE ( 'NONE', #4765, #8398, #16344, .T. ) ;
#13410=DIRECTION ( 'NONE',  ( -1.000000000000000000, -2.677423277737400817E-15, 0.000000000000000000 ) ) ;
#13414=ORIENTED_EDGE ( 'NONE', *, *, #15318, .F. ) ;
#13415=CARTESIAN_POINT ( 'NONE',  ( 2.775557561562891351E-14, -2.775557561562891351E-14, 2.999999999999999112 ) ) ;
#13416=DIRECTION ( 'NONE',  ( 6.505213034913038160E-19, 3.903127820947822896E-18, 1.000000000000000000 ) ) ;
#13417=EDGE_LOOP ( 'NONE', ( #21382, #9921, #19981, #4236 ) ) ;
#13418=CARTESIAN_POINT ( 'NONE',  ( 30.98879172160187423, -17.38064605515599226, 3.000000000000061728 ) ) ;
#13421=DIRECTION ( 'NONE',  ( -1.000000000000000000, -1.208970125616060101E-17, 6.505213034913038160E-19 ) ) ;
#13424=CIRCLE ( 'NONE', #11616, 36.76383501243555685 ) ;
#13426=EDGE_CURVE ( 'NONE', #12156, #16900, #17801, .T. ) ;
#13428=ORIENTED_EDGE ( 'NONE', *, *, #7897, .F. ) ;
#13429=ORIENTED_EDGE ( 'NONE', *, *, #11396, .T. ) ;
#13430=VERTEX_POINT ( 'NONE', #10916 ) ;
#13434=CIRCLE ( 'NONE', #18212, 20.00000000000002132 ) ;
#13435=ORIENTED_EDGE ( 'NONE', *, *, #21288, .F. ) ;
#13439=CARTESIAN_POINT ( 'NONE',  ( 11.93972437435558653, 29.14949368109859407, -7.000000000000006217 ) ) ;
#13440=CIRCLE ( 'NONE', #21150, 0.9999999999999974465 ) ;
#13441=ORIENTED_EDGE ( 'NONE', *, *, #12688, .T. ) ;
#13446=AXIS2_PLACEMENT_3D ( 'NONE', #17386, #16114, #3427 ) ;
#13449=ORIENTED_EDGE ( 'NONE', *, *, #16157, .F. ) ;
#13452=ORIENTED_EDGE ( 'NONE', *, *, #13368, .F. ) ;
#13455=ORIENTED_EDGE ( 'NONE', *, *, #16143, .T. ) ;
#13458=LINE ( 'NONE', #11755, #2689 ) ;
#13461=CARTESIAN_POINT ( 'NONE',  ( -30.33632613426173918, 11.35354668330684724, -6.999999999999957367 ) ) ;
#13462=CIRCLE ( 'NONE', #315, 3.000000000000002665 ) ;
#13467=CARTESIAN_POINT ( 'NONE',  ( -34.13396246814566837, 14.93538271375394189, -6.999999999999985789 ) ) ;
#13468=CARTESIAN_POINT ( 'NONE',  ( 31.88709182564697286, -6.070730550690988991, -2.999999999999971578 ) ) ;
#13469=AXIS2_PLACEMENT_3D ( 'NONE', #18210, #12918, #2639 ) ;
#13471=VERTEX_POINT ( 'NONE', #21466 ) ;
#13473=CARTESIAN_POINT ( 'NONE',  ( 1.110223024625156540E-13, -5.551115123125782702E-14, -6.999999999999950262 ) ) ;
#13475=VERTEX_POINT ( 'NONE', #12508 ) ;
#13479=ADVANCED_FACE ( 'NONE', ( #15955 ), #19758, .F. ) ;
#13480=ORIENTED_EDGE ( 'NONE', *, *, #3649, .F. ) ;
#13483=ORIENTED_EDGE ( 'NONE', *, *, #7385, .T. ) ;
#13485=DIRECTION ( 'NONE',  ( -6.505213034913038160E-19, -3.903127820947822896E-18, -1.000000000000000000 ) ) ;
#13486=ORIENTED_EDGE ( 'NONE', *, *, #12137, .F. ) ;
#13494=AXIS2_PLACEMENT_3D ( 'NONE', #6825, #21027, #5116 ) ;
#13496=CARTESIAN_POINT ( 'NONE',  ( 7.711478842616803497, -31.57187188083537777, -7.000000000000006217 ) ) ;
#13497=LINE ( 'NONE', #7918, #6373 ) ;
#13498=DIRECTION ( 'NONE',  ( 6.505213034913038160E-19, 3.903127820947822896E-18, 1.000000000000000000 ) ) ;
#13503=DIRECTION ( 'NONE',  ( -6.505213034913038160E-19, -3.903127820947822896E-18, -1.000000000000000000 ) ) ;
#13504=EDGE_CURVE ( 'NONE', #10205, #14672, #6059, .T. ) ;
#13505=EDGE_CURVE ( 'NONE', #43, #9799, #17327, .T. ) ;
#13514=CARTESIAN_POINT ( 'NONE',  ( -21.41958700883257904, -27.56232195404059837, -2.999999999999992450 ) ) ;
#13516=DIRECTION ( 'NONE',  ( -6.505213034913038160E-19, -3.903127820947822896E-18, -1.000000000000000000 ) ) ;
#13519=VERTEX_POINT ( 'NONE', #5769 ) ;
#13520=CYLINDRICAL_SURFACE ( 'NONE', #3628, 19.11328065563150957 ) ;
#13524=CARTESIAN_POINT ( 'NONE',  ( 28.07080038625115037, 14.29266125237890783, -6.999999999999950262 ) ) ;
#13534=DIRECTION ( 'NONE',  ( -1.000000000000000000, 0.000000000000000000, 0.000000000000000000 ) ) ;
#13535=CARTESIAN_POINT ( 'NONE',  ( 3.330669073875469621E-13, -1.110223024625156540E-13, -2.999999999999971578 ) ) ;
#13540=AXIS2_PLACEMENT_3D ( 'NONE', #8238, #19123, #8691 ) ;
#13542=VERTEX_POINT ( 'NONE', #18137 ) ;
#13543=ORIENTED_EDGE ( 'NONE', *, *, #6074, .T. ) ;
#13545=VERTEX_POINT ( 'NONE', #4509 ) ;
#13548=EDGE_CURVE ( 'NONE', #13199, #10901, #14867, .T. ) ;
#13550=CARTESIAN_POINT ( 'NONE',  ( 31.41239365194237365, -2.347663744114464102, 3.000000000000023537 ) ) ;
#13557=CARTESIAN_POINT ( 'NONE',  ( -13.74639653023206520, 28.96193690644924246, -2.999999999999968026 ) ) ;
#13558=CARTESIAN_POINT ( 'NONE',  ( -36.75746821813305587, 0.6841746959067307454, 2.800654218530485018 ) ) ;
#13560=AXIS2_PLACEMENT_3D ( 'NONE', #21122, #601, #14567 ) ;
#13563=VERTEX_POINT ( 'NONE', #1072 ) ;
#13565=ORIENTED_EDGE ( 'NONE', *, *, #9847, .F. ) ;
#13569=CARTESIAN_POINT ( 'NONE',  ( 26.50842683089782525, -24.41514043009201984, -6.999999999999992006 ) ) ;
#13570=FACE_OUTER_BOUND ( 'NONE', #5745, .T. ) ;
#13573=LINE ( 'NONE', #11873, #7277 ) ;
#13575=DIRECTION ( 'NONE',  ( -6.505213034913038160E-19, -3.903127820947822896E-18, -1.000000000000000000 ) ) ;
#13581=EDGE_CURVE ( 'NONE', #6508, #18887, #3389, .T. ) ;
#13582=DIRECTION ( 'NONE',  ( -1.000000000000000000, 0.000000000000000000, 0.000000000000000000 ) ) ;
#13583=LINE ( 'NONE', #4577, #15885 ) ;
#13586=EDGE_LOOP ( 'NONE', ( #21156, #2349, #9533, #20694, #7506, #22126 ) ) ;
#13588=CIRCLE ( 'NONE', #11044, 19.11328065563151668 ) ;
#13590=CARTESIAN_POINT ( 'NONE',  ( -21.65063509461084834, 12.49999999999967848, -2.999999999999988898 ) ) ;
#13593=B_SPLINE_CURVE_WITH_KNOTS ( 'NONE', 3,
 ( #9317, #12504, #11026, #2322 ),
 .UNSPECIFIED., .F., .F.,
 ( 4, 4 ),
 ( 9.545285768313558837E-07, 0.001900595205834684732 ),
 .UNSPECIFIED. ) ;
#13596=EDGE_CURVE ( 'NONE', #31, #16039, #8166, .T. ) ;
#13600=ORIENTED_EDGE ( 'NONE', *, *, #18581, .F. ) ;
#13605=ORIENTED_EDGE ( 'NONE', *, *, #1318, .T. ) ;
#13607=DIRECTION ( 'NONE',  ( 1.000000000000000000, 0.000000000000000000, 0.000000000000000000 ) ) ;
#13608=CYLINDRICAL_SURFACE ( 'NONE', #10019, 19.11328065563152379 ) ;
#13610=VECTOR ( 'NONE', #6944, 1000.000000000000000 ) ;
#13613=ORIENTED_EDGE ( 'NONE', *, *, #8890, .T. ) ;
#13614=CARTESIAN_POINT ( 'NONE',  ( 14.85437171138604207, -32.27599279215765904, 3.000000000000054179 ) ) ;
#13617=CIRCLE ( 'NONE', #14370, 34.90673715956759082 ) ;
#13619=DIRECTION ( 'NONE',  ( -1.000000000000000000, 0.000000000000000000, 0.000000000000000000 ) ) ;
#13621=LINE ( 'NONE', #6779, #15687 ) ;
#13625=CARTESIAN_POINT ( 'NONE',  ( -8.485281374238345720, 3.000000000000002665, -6.859353255829946150 ) ) ;
#13627=CARTESIAN_POINT ( 'NONE',  ( 1.942890293094023946E-13, -8.326672684688674053E-14, 4.999999999999993783 ) ) ;
#13629=DIRECTION ( 'NONE',  ( -1.000000000000000000, 1.815202222194848078E-15, 0.000000000000000000 ) ) ;
#13631=DIRECTION ( 'NONE',  ( -6.505213034913038160E-19, -3.903127820947822896E-18, -1.000000000000000000 ) ) ;
#13634=B_SPLINE_CURVE_WITH_KNOTS ( 'NONE', 3,
 ( #21295, #10618, #12453, #17623 ),
 .UNSPECIFIED., .F., .F.,
 ( 4, 4 ),
 ( 9.545285769942081322E-07, 0.001900595205834547038 ),
 .UNSPECIFIED. ) ;
#13639=CARTESIAN_POINT ( 'NONE',  ( 32.35999952201593288, -1.423424233832626395, -2.999999999999971578 ) ) ;
#13644=AXIS2_PLACEMENT_3D ( 'NONE', #16124, #14055, #17523 ) ;
#13646=CIRCLE ( 'NONE', #5273, 1.000000000000000888 ) ;
#13648=ORIENTED_EDGE ( 'NONE', *, *, #1957, .F. ) ;
#13649=ADVANCED_FACE ( 'NONE', ( #11933 ), #4847, .T. ) ;
#13650=ORIENTED_EDGE ( 'NONE', *, *, #3319, .T. ) ;
#13652=CARTESIAN_POINT ( 'NONE',  ( 2.775557561562891351E-14, 2.775557561562891351E-14, 5.750000000000001776 ) ) ;
#13656=ORIENTED_EDGE ( 'NONE', *, *, #10439, .F. ) ;
#13657=DIRECTION ( 'NONE',  ( -1.000000000000000000, -1.208970125616092456E-17, 0.000000000000000000 ) ) ;
#13661=AXIS2_PLACEMENT_3D ( 'NONE', #7649, #14620, #16227 ) ;
#13662=ORIENTED_EDGE ( 'NONE', *, *, #331, .F. ) ;
#13669=EDGE_CURVE ( 'NONE', #5811, #5141, #16674, .T. ) ;
#13676=VECTOR ( 'NONE', #3175, 1000.000000000000000 ) ;
#13678=ORIENTED_EDGE ( 'NONE', *, *, #21539, .T. ) ;
#13686=ORIENTED_EDGE ( 'NONE', *, *, #20469, .F. ) ;
#13692=EDGE_CURVE ( 'NONE', #18082, #2079, #1402, .T. ) ;
#13697=CARTESIAN_POINT ( 'NONE',  ( -13.06969024216331476, -19.15111107797470780, 2.999999999999995559 ) ) ;
#13701=AXIS2_PLACEMENT_3D ( 'NONE', #20920, #5220, #11662 ) ;
#13710=VERTEX_POINT ( 'NONE', #4954 ) ;
#13711=EDGE_CURVE ( 'NONE', #17952, #1823, #4968, .T. ) ;
#13712=DIRECTION ( 'NONE',  ( 6.505213034913038160E-19, 3.903127820947822896E-18, 1.000000000000000000 ) ) ;
#13715=AXIS2_PLACEMENT_3D ( 'NONE', #8951, #3703, #5195 ) ;
#13719=ORIENTED_EDGE ( 'NONE', *, *, #6475, .T. ) ;
#13727=LINE ( 'NONE', #3100, #2884 ) ;
#13735=EDGE_CURVE ( 'NONE', #12221, #1729, #21798, .T. ) ;
#13740=CARTESIAN_POINT ( 'NONE',  ( -7.463862311151175710, -35.99819890246952525, -2.800654218530457484 ) ) ;
#13744=ORIENTED_EDGE ( 'NONE', *, *, #12557, .F. ) ;
#13746=CARTESIAN_POINT ( 'NONE',  ( -14.93538271375417814, -34.13396246814587442, -6.999999999999950262 ) ) ;
#13748=DIRECTION ( 'NONE',  ( 6.505213034913038160E-19, 3.903127820947822896E-18, 1.000000000000000000 ) ) ;
#13754=DIRECTION ( 'NONE',  ( 6.505213034913038160E-19, 3.903127820947822896E-18, 1.000000000000000000 ) ) ;
#13761=DIRECTION ( 'NONE',  ( -1.000000000000000000, -1.208970125616081209E-17, 0.000000000000000000 ) ) ;
#13766=ORIENTED_EDGE ( 'NONE', *, *, #9948, .T. ) ;
#13769=CARTESIAN_POINT ( 'NONE',  ( -12.31876324338271367, -30.07487443287973505, -2.999999999999995559 ) ) ;
#13772=DIRECTION ( 'NONE',  ( 1.000000000000000000, 0.000000000000000000, 0.000000000000000000 ) ) ;
#13775=ADVANCED_FACE ( 'NONE', ( #11320 ), #18917, .T. ) ;
#13785=ADVANCED_FACE ( 'NONE', ( #429 ), #890, .F. ) ;
#13787=DIRECTION ( 'NONE',  ( 6.505213034913038160E-19, 3.903127820947822896E-18, 1.000000000000000000 ) ) ;
#13789=ADVANCED_FACE ( 'NONE', ( #16582 ), #12271, .T. ) ;
#13790=CIRCLE ( 'NONE', #4671, 1.000000000000000888 ) ;
#13791=CARTESIAN_POINT ( 'NONE',  ( -21.05198877411783442, 30.13956425491229396, -2.800654218530457484 ) ) ;
#13792=CARTESIAN_POINT ( 'NONE',  ( -1.128083539116059297, -34.88850421923977763, 2.999999999999995559 ) ) ;
#13794=ORIENTED_EDGE ( 'NONE', *, *, #1082, .T. ) ;
#13797=VERTEX_POINT ( 'NONE', #19807 ) ;
#13798=EDGE_CURVE ( 'NONE', #3722, #10477, #366, .T. ) ;
#13799=ORIENTED_EDGE ( 'NONE', *, *, #3680, .T. ) ;
#13801=CARTESIAN_POINT ( 'NONE',  ( -37.07861450834793970, 3.656418565264024423, -2.999999999999988898 ) ) ;
#13807=CIRCLE ( 'NONE', #5052, 0.9999999999999991118 ) ;
#13808=ORIENTED_EDGE ( 'NONE', *, *, #10227, .F. ) ;
#13809=CARTESIAN_POINT ( 'NONE',  ( 2.220446049250313081E-13, -2.498001805406602216E-13, -6.859353255829918616 ) ) ;
#13815=DIRECTION ( 'NONE',  ( -6.505213034913038160E-19, -3.903127820947822896E-18, -1.000000000000000000 ) ) ;
#13818=VERTEX_POINT ( 'NONE', #11196 ) ;
#13819=CARTESIAN_POINT ( 'NONE',  ( -1.128083539116059297, -34.88850421923977763, 2.999999999999995559 ) ) ;
#13824=CARTESIAN_POINT ( 'NONE',  ( 3.330669073875469621E-13, -1.110223024625156540E-13, -2.999999999999971578 ) ) ;
#13825=AXIS2_PLACEMENT_3D ( 'NONE', #20582, #13341, #22323 ) ;
#13829=DIRECTION ( 'NONE',  ( -1.000000000000000000, -1.208970125616046080E-17, 6.505213034913038160E-19 ) ) ;
#13831=CARTESIAN_POINT ( 'NONE',  ( 35.33352588067112521, 7.094908322882925944, -6.999999999999999112 ) ) ;
#13833=VECTOR ( 'NONE', #15274, 1000.000000000000000 ) ;
#13841=VERTEX_POINT ( 'NONE', #21751 ) ;
#13845=VERTEX_POINT ( 'NONE', #5706 ) ;
#13847=CARTESIAN_POINT ( 'NONE',  ( -16.56444186175072630, 26.79308242454869671, -6.999999999999950262 ) ) ;
#13855=DIRECTION ( 'NONE',  ( -6.505213034913038160E-19, -3.903127820947822896E-18, -1.000000000000000000 ) ) ;
#13856=DIRECTION ( 'NONE',  ( -1.000000000000000000, -1.815202222194848473E-15, 0.000000000000000000 ) ) ;
#13859=CIRCLE ( 'NONE', #13494, 36.76383501243555685 ) ;
#13863=DIRECTION ( 'NONE',  ( 6.505213034913038160E-19, 3.903127820947822896E-18, 1.000000000000000000 ) ) ;
#13864=ORIENTED_EDGE ( 'NONE', *, *, #2014, .T. ) ;
#13869=ORIENTED_EDGE ( 'NONE', *, *, #10439, .T. ) ;
#13872=ADVANCED_FACE ( 'NONE', ( #16819 ), #13365, .T. ) ;
#13879=VECTOR ( 'NONE', #9935, 1000.000000000000000 ) ;
#13880=ORIENTED_EDGE ( 'NONE', *, *, #17983, .T. ) ;
#13881=EDGE_LOOP ( 'NONE', ( #13207, #17570, #14812, #13894 ) ) ;
#13882=ORIENTED_EDGE ( 'NONE', *, *, #17010, .T. ) ;
#13884=VERTEX_POINT ( 'NONE', #20862 ) ;
#13885=CARTESIAN_POINT ( 'NONE',  ( 36.39375341857550694, 7.980461308159797262, -6.999999999999971578 ) ) ;
#13887=CIRCLE ( 'NONE', #4045, 19.11328065563150957 ) ;
#13893=CARTESIAN_POINT ( 'NONE',  ( 2.220446049250313081E-13, 2.775557561562891351E-14, -2.800654218530485018 ) ) ;
#13894=ORIENTED_EDGE ( 'NONE', *, *, #6921, .F. ) ;
#13895=CARTESIAN_POINT ( 'NONE',  ( 1.110223024625156540E-13, -5.551115123125782702E-14, -6.999999999999950262 ) ) ;
#13900=EDGE_CURVE ( 'NONE', #11717, #17625, #19250, .T. ) ;
#13903=DIRECTION ( 'NONE',  ( -6.505213034913038160E-19, -3.903127820947822896E-18, -1.000000000000000000 ) ) ;
#13908=ORIENTED_EDGE ( 'NONE', *, *, #21649, .F. ) ;
#13910=ORIENTED_EDGE ( 'NONE', *, *, #4506, .F. ) ;
#13911=DIRECTION ( 'NONE',  ( -1.000000000000000000, 2.663326288974754901E-14, 0.000000000000000000 ) ) ;
#13915=CARTESIAN_POINT ( 'NONE',  ( 5.551115123125782702E-14, -1.387778780781445676E-13, -5.749999999999949374 ) ) ;
#13918=CARTESIAN_POINT ( 'NONE',  ( -34.64233806479151667, -10.34893680499436819, 2.932969818539049811 ) ) ;
#13920=EDGE_CURVE ( 'NONE', #14529, #10205, #8925, .T. ) ;
#13922=EDGE_CURVE ( 'NONE', #2563, #4860, #2052, .T. ) ;
#13925=VERTEX_POINT ( 'NONE', #19585 ) ;
#13926=CARTESIAN_POINT ( 'NONE',  ( -7.524443153164583897, 20.67323765728967899, 2.999999999999992450 ) ) ;
#13929=EDGE_CURVE ( 'NONE', #15217, #10145, #20352, .T. ) ;
#13931=ORIENTED_EDGE ( 'NONE', *, *, #8717, .F. ) ;
#13932=VERTEX_POINT ( 'NONE', #17527 ) ;
#13936=AXIS2_PLACEMENT_3D ( 'NONE', #22480, #4832, #18806 ) ;
#13942=VERTEX_POINT ( 'NONE', #1837 ) ;
#13945=DIRECTION ( 'NONE',  ( 1.000000000000000000, 1.208970125616065955E-17, 0.000000000000000000 ) ) ;
#13946=DIRECTION ( 'NONE',  ( -6.505213034913038160E-19, -3.903127820947822896E-18, -1.000000000000000000 ) ) ;
#13948=ORIENTED_EDGE ( 'NONE', *, *, #2028, .T. ) ;
#13949=EDGE_CURVE ( 'NONE', #12221, #2570, #1938, .T. ) ;
#13950=DIRECTION ( 'NONE',  ( 6.505213034913038160E-19, 3.903127820947822896E-18, 1.000000000000000000 ) ) ;
#13951=VECTOR ( 'NONE', #21558, 1000.000000000000000 ) ;
#13953=ORIENTED_EDGE ( 'NONE', *, *, #22437, .T. ) ;
#13955=CARTESIAN_POINT ( 'NONE',  ( 3.330669073875469621E-13, -1.110223024625156540E-13, -2.999999999999971578 ) ) ;
#13958=FACE_OUTER_BOUND ( 'NONE', #12176, .T. ) ;
#13960=ORIENTED_EDGE ( 'NONE', *, *, #20012, .F. ) ;
#13961=CARTESIAN_POINT ( 'NONE',  ( -36.76383501243539342, 2.727773753693014013E-14, -2.800654218530485018 ) ) ;
#13962=DIRECTION ( 'NONE',  ( -1.000000000000000000, 1.815202222194848473E-15, 0.000000000000000000 ) ) ;
#13964=CARTESIAN_POINT ( 'NONE',  ( 4.153516728483875653, -35.28654656445792170, 3.000000000000031974 ) ) ;
#13966=AXIS2_PLACEMENT_3D ( 'NONE', #8781, #15635, #13911 ) ;
#13973=ORIENTED_EDGE ( 'NONE', *, *, #4579, .T. ) ;
#13974=DIRECTION ( 'NONE',  ( -6.505213034913038160E-19, -3.903127820947822896E-18, -1.000000000000000000 ) ) ;
#13975=DIRECTION ( 'NONE',  ( -1.000000000000000000, 0.000000000000000000, 0.000000000000000000 ) ) ;
#13977=ORIENTED_EDGE ( 'NONE', *, *, #5661, .F. ) ;
#13978=VERTEX_POINT ( 'NONE', #100 ) ;
#13980=AXIS2_PLACEMENT_3D ( 'NONE', #14921, #21826, #20447 ) ;
#13986=ORIENTED_EDGE ( 'NONE', *, *, #15105, .T. ) ;
#13988=CARTESIAN_POINT ( 'NONE',  ( -30.33632613426172497, 11.35354668330676375, -2.999999999999988898 ) ) ;
#13989=ORIENTED_EDGE ( 'NONE', *, *, #17497, .T. ) ;
#13993=ORIENTED_EDGE ( 'NONE', *, *, #5497, .T. ) ;
#13995=EDGE_LOOP ( 'NONE', ( #21282, #3710, #13455, #4683, #13766, #4385 ) ) ;
#13996=DIRECTION ( 'NONE',  ( -6.505213034913038160E-19, -3.903127820947822896E-18, -1.000000000000000000 ) ) ;
#13997=CARTESIAN_POINT ( 'NONE',  ( 19.05255888325763181, 11.00000000000003730, -2.999999999999971578 ) ) ;
#14009=ORIENTED_EDGE ( 'NONE', *, *, #11948, .F. ) ;
#14012=LINE ( 'NONE', #6715, #14701 ) ;
#14020=EDGE_CURVE ( 'NONE', #12202, #1817, #8261, .T. ) ;
#14023=CARTESIAN_POINT ( 'NONE',  ( 33.51030287062373247, 15.12081897056669000, -2.800654218530485018 ) ) ;
#14028=DIRECTION ( 'NONE',  ( 6.505213034913038160E-19, 3.903127820947822896E-18, 1.000000000000000000 ) ) ;
#14029=CIRCLE ( 'NONE', #15501, 34.90673715956759082 ) ;
#14032=DIRECTION ( 'NONE',  ( -6.505213034913038160E-19, -3.903127820947822896E-18, -1.000000000000000000 ) ) ;
#14033=DIRECTION ( 'NONE',  ( -6.505213034913038160E-19, -3.903127820947822896E-18, -1.000000000000000000 ) ) ;
#14038=EDGE_CURVE ( 'NONE', #2882, #13818, #16996, .T. ) ;
#14039=ORIENTED_EDGE ( 'NONE', *, *, #1905, .F. ) ;
#14043=AXIS2_PLACEMENT_3D ( 'NONE', #17974, #2278, #11332 ) ;
#14055=DIRECTION ( 'NONE',  ( 6.505213034913038160E-19, 3.903127820947822896E-18, 1.000000000000000000 ) ) ;
#14058=AXIS2_PLACEMENT_3D ( 'NONE', #19005, #1128, #13582 ) ;
#14062=AXIS2_PLACEMENT_3D ( 'NONE', #20840, #3417, #19006 ) ;
#14063=ORIENTED_EDGE ( 'NONE', *, *, #1917, .F. ) ;
#14066=ORIENTED_EDGE ( 'NONE', *, *, #20183, .T. ) ;
#14068=CARTESIAN_POINT ( 'NONE',  ( -34.84300730320195072, 6.953913411054657878, 3.000000000000048850 ) ) ;
#14071=DIRECTION ( 'NONE',  ( 6.505213034913038160E-19, 3.903127820947822896E-18, 1.000000000000000000 ) ) ;
#14072=DIRECTION ( 'NONE',  ( 1.000000000000000000, 0.000000000000000000, 0.000000000000000000 ) ) ;
#14073=ORIENTED_EDGE ( 'NONE', *, *, #11966, .F. ) ;
#14074=DIRECTION ( 'NONE',  ( -1.000000000000000000, 0.000000000000000000, 0.000000000000000000 ) ) ;
#14075=DIRECTION ( 'NONE',  ( -6.505213034913038160E-19, -3.903127820947822896E-18, -1.000000000000000000 ) ) ;
#14081=LINE ( 'NONE', #3245, #16991 ) ;
#14086=DIRECTION ( 'NONE',  ( -1.000000000000000000, -1.208970125616081209E-17, 0.000000000000000000 ) ) ;
#14093=CIRCLE ( 'NONE', #20721, 0.9999999999999974465 ) ;
#14095=B_SPLINE_CURVE_WITH_KNOTS ( 'NONE', 3,
 ( #11683, #920, #16501, #7915 ),
 .UNSPECIFIED., .F., .F.,
 ( 4, 4 ),
 ( 0.001875451646902739260, 0.003761979286330971450 ),
 .UNSPECIFIED. ) ;
#14096=VERTEX_POINT ( 'NONE', #17865 ) ;
#14097=EDGE_CURVE ( 'NONE', #2692, #9285, #10766, .T. ) ;
#14101=CYLINDRICAL_SURFACE ( 'NONE', #3707, 1.000000000000000888 ) ;
#14107=AXIS2_PLACEMENT_3D ( 'NONE', #12303, #14225, #19419 ) ;
#14110=DIRECTION ( 'NONE',  ( 1.000000000000000000, 0.000000000000000000, 0.000000000000000000 ) ) ;
#14111=TOROIDAL_SURFACE ( 'NONE', #4265, 34.90673715956759082, 8.750000000000000000 ) ;
#14115=ADVANCED_FACE ( 'NONE', ( #5717 ), #19817, .T. ) ;
#14121=CYLINDRICAL_SURFACE ( 'NONE', #2675, 31.50000000000000000 ) ;
#14122=CARTESIAN_POINT ( 'NONE',  ( 2.220446049250313081E-13, 2.775557561562891351E-14, -2.800654218530485018 ) ) ;
#14124=EDGE_LOOP ( 'NONE', ( #15058, #10815, #15463, #14595 ) ) ;
#14126=EDGE_LOOP ( 'NONE', ( #19325, #1291, #16779, #5074 ) ) ;
#14130=DIRECTION ( 'NONE',  ( -1.000000000000000000, -1.815202222194848473E-15, 0.000000000000000000 ) ) ;
#14132=CARTESIAN_POINT ( 'NONE',  ( -12.31876324338254669, -30.07487443287981677, -6.999999999999950262 ) ) ;
#14134=CARTESIAN_POINT ( 'NONE',  ( 24.24871130596423185, 14.00000000000009592, 2.999999999999995559 ) ) ;
#14139=DIRECTION ( 'NONE',  ( -1.000000000000000000, 1.597512185334606831E-14, 0.000000000000000000 ) ) ;
#14145=EDGE_CURVE ( 'NONE', #13471, #3795, #12804, .T. ) ;
#14146=FACE_OUTER_BOUND ( 'NONE', #16388, .T. ) ;
#14149=DIRECTION ( 'NONE',  ( -1.000000000000000000, -1.208970125616060717E-17, 0.000000000000000000 ) ) ;
#14152=ADVANCED_FACE ( 'NONE', ( #12690 ), #16593, .F. ) ;
#14156=AXIS2_PLACEMENT_3D ( 'NONE', #7415, #21064, #5366 ) ;
#14157=ORIENTED_EDGE ( 'NONE', *, *, #975, .F. ) ;
#14159=DIRECTION ( 'NONE',  ( -6.505213034913038160E-19, -3.903127820947822896E-18, -1.000000000000000000 ) ) ;
#14161=ADVANCED_FACE ( 'NONE', ( #4120 ), #4018, .F. ) ;
#14163=CARTESIAN_POINT ( 'NONE',  ( 1.110223024625156540E-13, -5.551115123125782702E-14, -6.999999999999950262 ) ) ;
#14168=CYLINDRICAL_SURFACE ( 'NONE', #11954, 19.11328065563152379 ) ;
#14170=CARTESIAN_POINT ( 'NONE',  ( 36.75746821813308429, -0.6841746959067585010, 2.800654218530485018 ) ) ;
#14177=CARTESIAN_POINT ( 'NONE',  ( 5.551115123125782702E-14, -1.387778780781445676E-13, -5.749999999999949374 ) ) ;
#14178=DIRECTION ( 'NONE',  ( 6.505213034913038160E-19, 3.903127820947822896E-18, 1.000000000000000000 ) ) ;
#14182=AXIS2_PLACEMENT_3D ( 'NONE', #6363, #6479, #10017 ) ;
#14183=CIRCLE ( 'NONE', #20461, 1.000000000000001776 ) ;
#14184=VERTEX_POINT ( 'NONE', #21881 ) ;
#14186=CARTESIAN_POINT ( 'NONE',  ( 2.220446049250313081E-13, 2.775557561562891351E-14, -2.800654218530485018 ) ) ;
#14187=DIRECTION ( 'NONE',  ( -6.505213034913038160E-19, -3.903127820947822896E-18, -1.000000000000000000 ) ) ;
#14191=CARTESIAN_POINT ( 'NONE',  ( 11.85401191286899980, 32.83234229683715455, 2.999999999999995559 ) ) ;
#14194=DIRECTION ( 'NONE',  ( -6.505213034913038160E-19, -3.903127820947822896E-18, -1.000000000000000000 ) ) ;
#14201=CIRCLE ( 'NONE', #3776, 3.000000000000002665 ) ;
#14202=EDGE_CURVE ( 'NONE', #4210, #20847, #17371, .T. ) ;
#14206=ORIENTED_EDGE ( 'NONE', *, *, #7313, .F. ) ;
#14213=AXIS2_PLACEMENT_3D ( 'NONE', #14941, #7856, #6481 ) ;
#14215=ORIENTED_EDGE ( 'NONE', *, *, #19563, .T. ) ;
#14219=DIRECTION ( 'NONE',  ( -6.505213034913038160E-19, -3.903127820947822896E-18, -1.000000000000000000 ) ) ;
#14221=DIRECTION ( 'NONE',  ( -1.000000000000000000, -4.356485333267636965E-15, 0.000000000000000000 ) ) ;
#14222=DIRECTION ( 'NONE',  ( 6.505213034913038160E-19, 3.903127820947822896E-18, 1.000000000000000000 ) ) ;
#14224=CARTESIAN_POINT ( 'NONE',  ( 20.36304159388371815, 24.03323817228478276, -2.999999999999999112 ) ) ;
#14225=DIRECTION ( 'NONE',  ( -6.505213034913038160E-19, -3.903127820947822896E-18, -1.000000000000000000 ) ) ;
#14228=LINE ( 'NONE', #8865, #667 ) ;
#14229=VERTEX_POINT ( 'NONE', #1129 ) ;
#14230=CARTESIAN_POINT ( 'NONE',  ( -9.999999999999758415, -3.000000000000169198, -4.999999999999984013 ) ) ;
#14231=DIRECTION ( 'NONE',  ( 6.505213034913038160E-19, 3.903127820947822896E-18, 1.000000000000000000 ) ) ;
#14232=CARTESIAN_POINT ( 'NONE',  ( -8.485281374238429208, 2.999999999999808153, 5.000000000000018652 ) ) ;
#14239=EDGE_CURVE ( 'NONE', #21378, #2694, #8589, .T. ) ;
#14240=CARTESIAN_POINT ( 'NONE',  ( 28.14364593009904425, -21.69710536060321715, 3.000000000000048850 ) ) ;
#14246=ORIENTED_EDGE ( 'NONE', *, *, #13798, .T. ) ;
#14247=CARTESIAN_POINT ( 'NONE',  ( -24.79619811426189813, 21.00948735876859175, -2.999999999999999112 ) ) ;
#14252=CYLINDRICAL_SURFACE ( 'NONE', #8736, 1.000000000000000888 ) ;
#14257=CARTESIAN_POINT ( 'NONE',  ( 7.463862311151453710, 35.99819890246955367, 2.800654218530485018 ) ) ;
#14270=CARTESIAN_POINT ( 'NONE',  ( -6.953913411054715610, -34.84300730320209283, 3.000000000000044409 ) ) ;
#14272=DIRECTION ( 'NONE',  ( 1.000000000000000000, 1.208970125616063182E-17, 0.000000000000000000 ) ) ;
#14275=DIRECTION ( 'NONE',  ( 6.505213034913038160E-19, 3.903127820947822896E-18, 1.000000000000000000 ) ) ;
#14280=ADVANCED_FACE ( 'NONE', ( #20385 ), #17153, .T. ) ;
#14283=DIRECTION ( 'NONE',  ( -1.000000000000000000, -1.208970125616046080E-17, 6.505213034913038160E-19 ) ) ;
#14289=AXIS2_PLACEMENT_3D ( 'NONE', #8266, #22600, #20531 ) ;
#14290=B_SPLINE_CURVE_WITH_KNOTS ( 'NONE', 3,
 ( #271, #1999, #5142, #2226 ),
 .UNSPECIFIED., .F., .F.,
 ( 4, 4 ),
 ( 9.715086410652220024E-07, 0.001929643240672559339 ),
 .UNSPECIFIED. ) ;
#14291=CARTESIAN_POINT ( 'NONE',  ( 24.75236754129178607, 27.84804035626031649, -2.999999999999971578 ) ) ;
#14294=EDGE_CURVE ( 'NONE', #15936, #15170, #13583, .T. ) ;
#14296=VECTOR ( 'NONE', #13855, 1000.000000000000000 ) ;
#14303=VERTEX_POINT ( 'NONE', #18664 ) ;
#14307=CARTESIAN_POINT ( 'NONE',  ( 10.70799354677381920, -35.16985127952404611, -2.800654218530477912 ) ) ;
#14310=B_SPLINE_CURVE_WITH_KNOTS ( 'NONE', 3,
 ( #6058, #1130, #4578, #13026 ),
 .UNSPECIFIED., .F., .F.,
 ( 4, 4 ),
 ( 9.715086410669694314E-07, 0.001929643240672542425 ),
 .UNSPECIFIED. ) ;
#14319=CIRCLE ( 'NONE', #4468, 1.000000000000000888 ) ;
#14324=ORIENTED_EDGE ( 'NONE', *, *, #21627, .T. ) ;
#14329=DIRECTION ( 'NONE',  ( 6.505213034913038160E-19, 3.903127820947822896E-18, 1.000000000000000000 ) ) ;
#14330=DIRECTION ( 'NONE',  ( -6.505213034913038160E-19, -3.903127820947822896E-18, -1.000000000000000000 ) ) ;
#14335=DIRECTION ( 'NONE',  ( -1.000000000000000000, -1.208970125616027129E-17, 0.000000000000000000 ) ) ;
#14336=CYLINDRICAL_SURFACE ( 'NONE', #3211, 0.9999999999999974465 ) ;
#14337=ORIENTED_EDGE ( 'NONE', *, *, #9164, .T. ) ;
#14338=DIRECTION ( 'NONE',  ( -6.505213034913038160E-19, -3.903127820947822896E-18, -1.000000000000000000 ) ) ;
#14343=VERTEX_POINT ( 'NONE', #15872 ) ;
#14344=DIRECTION ( 'NONE',  ( -0.7071067811865524577, -1.130863789078082253E-17, -0.7071067811865426878 ) ) ;
#14347=CARTESIAN_POINT ( 'NONE',  ( -28.88846368933341324, -19.59430950039325836, -2.999999999999947153 ) ) ;
#14355=B_SPLINE_CURVE_WITH_KNOTS ( 'NONE', 3,
 ( #10199, #6321, #3005, #4735 ),
 .UNSPECIFIED., .F., .F.,
 ( 4, 4 ),
 ( 9.715086409635437439E-07, 0.001929643240672442245 ),
 .UNSPECIFIED. ) ;
#14356=CONICAL_SURFACE ( 'NONE', #11074, 20.00000000000002132, 0.7853981633974543852 ) ;
#14358=ORIENTED_EDGE ( 'NONE', *, *, #17374, .F. ) ;
#14360=ORIENTED_EDGE ( 'NONE', *, *, #7017, .T. ) ;
#14361=CARTESIAN_POINT ( 'NONE',  ( -32.10132595304119008, -5.074925817841968723, -2.999999999999971578 ) ) ;
#14364=ORIENTED_EDGE ( 'NONE', *, *, #2621, .F. ) ;
#14365=FACE_OUTER_BOUND ( 'NONE', #15207, .T. ) ;
#14366=CARTESIAN_POINT ( 'NONE',  ( 2.220446049250313081E-13, -8.326672684688674053E-14, 2.800654218530498785 ) ) ;
#14368=EDGE_CURVE ( 'NONE', #12073, #12156, #7861, .T. ) ;
#14370=AXIS2_PLACEMENT_3D ( 'NONE', #19438, #10480, #3293 ) ;
#14371=ORIENTED_EDGE ( 'NONE', *, *, #19990, .T. ) ;
#14372=CARTESIAN_POINT ( 'NONE',  ( 2.220446049250313081E-13, 2.775557561562891351E-14, -2.800654218530485018 ) ) ;
#14377=EDGE_CURVE ( 'NONE', #11652, #10901, #10274, .T. ) ;
#14378=CARTESIAN_POINT ( 'NONE',  ( 28.13960001536971234, -21.69517388068267039, -2.999999999999977796 ) ) ;
#14384=CIRCLE ( 'NONE', #19536, 19.11328065563151668 ) ;
#14385=ORIENTED_EDGE ( 'NONE', *, *, #4440, .F. ) ;
#14387=FACE_OUTER_BOUND ( 'NONE', #7469, .T. ) ;
#14388=EDGE_CURVE ( 'NONE', #18499, #5003, #20334, .T. ) ;
#14389=DIRECTION ( 'NONE',  ( -1.000000000000000000, -1.208970125616046080E-17, 6.505213034913038160E-19 ) ) ;
#14391=DIRECTION ( 'NONE',  ( 6.505213034913038160E-19, 3.903127820947822896E-18, 1.000000000000000000 ) ) ;
#14393=CARTESIAN_POINT ( 'NONE',  ( 1.423424233832626395, 32.35999952201593288, -6.999999999999999112 ) ) ;
#14394=CYLINDRICAL_SURFACE ( 'NONE', #2155, 1.000000000000000888 ) ;
#14395=DIRECTION ( 'NONE',  ( 1.000000000000000000, 0.000000000000000000, 0.000000000000000000 ) ) ;
#14402=DIRECTION ( 'NONE',  ( -1.000000000000000000, -2.677423277737400817E-15, 0.000000000000000000 ) ) ;
#14403=DIRECTION ( 'NONE',  ( 1.000000000000000000, 0.000000000000000000, 0.000000000000000000 ) ) ;
#14410=EDGE_CURVE ( 'NONE', #10013, #21090, #16659, .T. ) ;
#14412=ORIENTED_EDGE ( 'NONE', *, *, #18071, .F. ) ;
#14413=CARTESIAN_POINT ( 'NONE',  ( -10.00000000000000888, 2.999999999999836131, -4.999999999999948486 ) ) ;
#14429=CIRCLE ( 'NONE', #14058, 2.999999999999999112 ) ;
#14435=FACE_OUTER_BOUND ( 'NONE', #16888, .T. ) ;
#14436=EDGE_CURVE ( 'NONE', #6859, #2966, #20187, .T. ) ;
#14437=AXIS2_PLACEMENT_3D ( 'NONE', #11501, #16430, #743 ) ;
#14439=AXIS2_PLACEMENT_3D ( 'NONE', #18784, #9856, #1034 ) ;
#14440=EDGE_LOOP ( 'NONE', ( #7087, #14215, #749, #1602 ) ) ;
#14441=ORIENTED_EDGE ( 'NONE', *, *, #4842, .F. ) ;
#14442=VERTEX_POINT ( 'NONE', #17609 ) ;
#14443=DIRECTION ( 'NONE',  ( 1.000000000000000000, 0.000000000000000000, 0.000000000000000000 ) ) ;
#14447=CARTESIAN_POINT ( 'NONE',  ( 17.09029715894935819, -27.64365646977296009, 2.999999999999995559 ) ) ;
#14450=LINE ( 'NONE', #21461, #12701 ) ;
#14454=CARTESIAN_POINT ( 'NONE',  ( -32.14641817400173807, -18.83615802559818064, -6.999999999999992006 ) ) ;
#14456=VERTEX_POINT ( 'NONE', #6818 ) ;
#14464=ORIENTED_EDGE ( 'NONE', *, *, #20210, .T. ) ;
#14467=FACE_OUTER_BOUND ( 'NONE', #14901, .T. ) ;
#14468=AXIS2_PLACEMENT_3D ( 'NONE', #19865, #3721, #15834 ) ;
#14477=CIRCLE ( 'NONE', #15191, 34.90673715956759082 ) ;
#14486=DIRECTION ( 'NONE',  ( 6.505213034913038160E-19, 3.903127820947822896E-18, 1.000000000000000000 ) ) ;
#14489=ORIENTED_EDGE ( 'NONE', *, *, #14576, .F. ) ;
#14490=DIRECTION ( 'NONE',  ( -6.505213034913038160E-19, -3.903127820947822896E-18, -1.000000000000000000 ) ) ;
#14496=EDGE_CURVE ( 'NONE', #1823, #3953, #10871, .T. ) ;
#14497=CIRCLE ( 'NONE', #9011, 34.90673715956759082 ) ;
#14498=EDGE_CURVE ( 'NONE', #1368, #20409, #2936, .T. ) ;
#14500=CARTESIAN_POINT ( 'NONE',  ( 17.86915608785671949, -27.01645732367855146, -6.999999999999950262 ) ) ;
#14502=EDGE_LOOP ( 'NONE', ( #4229, #22607, #10610, #4384 ) ) ;
#14503=CIRCLE ( 'NONE', #12319, 0.9999999999999974465 ) ;
#14506=ORIENTED_EDGE ( 'NONE', *, *, #11650, .T. ) ;
#14509=VECTOR ( 'NONE', #21298, 1000.000000000000000 ) ;
#14514=CARTESIAN_POINT ( 'NONE',  ( -14.74639653023226948, 28.96193690644935259, 2.999999999999995559 ) ) ;
#14515=DIRECTION ( 'NONE',  ( 6.505213034913038160E-19, 3.903127820947822896E-18, 1.000000000000000000 ) ) ;
#14516=ORIENTED_EDGE ( 'NONE', *, *, #13798, .F. ) ;
#14517=LINE ( 'NONE', #21528, #9327 ) ;
#14518=CARTESIAN_POINT ( 'NONE',  ( 30.60042966911735718, 7.474202570535965151, 2.999999999999995559 ) ) ;
#14522=AXIS2_PLACEMENT_3D ( 'NONE', #12740, #14222, #9432 ) ;
#14523=CARTESIAN_POINT ( 'NONE',  ( -16.06969024216331476, -19.15111107797465451, 2.999999999999995559 ) ) ;
#14529=VERTEX_POINT ( 'NONE', #18709 ) ;
#14530=CYLINDRICAL_SURFACE ( 'NONE', #11500, 36.76383501243555685 ) ;
#14538=DIRECTION ( 'NONE',  ( -1.000000000000000000, -1.208970125616044077E-17, 0.000000000000000000 ) ) ;
#14541=ORIENTED_EDGE ( 'NONE', *, *, #2927, .T. ) ;
#14542=CARTESIAN_POINT ( 'NONE',  ( 11.93830856187213207, 33.47097213929420434, 3.000000000000055955 ) ) ;
#14546=CARTESIAN_POINT ( 'NONE',  ( -28.73837443790552371, 21.94460005644904754, -2.932164912090533981 ) ) ;
#14549=ORIENTED_EDGE ( 'NONE', *, *, #163, .T. ) ;
#14557=CARTESIAN_POINT ( 'NONE',  ( -22.98755168577401520, -22.97438720605754625, -2.999999999999971578 ) ) ;
#14560=AXIS2_PLACEMENT_3D ( 'NONE', #5985, #21924, #2559 ) ;
#14564=( NAMED_UNIT ( * ) SI_UNIT ( $, .STERADIAN. ) SOLID_ANGLE_UNIT ( ) );
#14565=EDGE_LOOP ( 'NONE', ( #10786, #17993, #2215, #7710 ) ) ;
#14567=DIRECTION ( 'NONE',  ( -1.000000000000000000, 0.000000000000000000, 0.000000000000000000 ) ) ;
#14568=DIRECTION ( 'NONE',  ( -6.505213034913038160E-19, -3.903127820947822896E-18, -1.000000000000000000 ) ) ;
#14573=CIRCLE ( 'NONE', #10189, 2.999999999999999112 ) ;
#14574=VERTEX_POINT ( 'NONE', #1284 ) ;
#14575=CARTESIAN_POINT ( 'NONE',  ( 20.06142356895430368, -29.33203831401597483, 3.000000000000046629 ) ) ;
#14576=EDGE_CURVE ( 'NONE', #10262, #22056, #22533, .T. ) ;
#14578=AXIS2_PLACEMENT_3D ( 'NONE', #21379, #17937, #11053 ) ;
#14583=ORIENTED_EDGE ( 'NONE', *, *, #9336, .T. ) ;
#14587=EDGE_CURVE ( 'NONE', #3870, #12877, #2766, .T. ) ;
#14591=DIRECTION ( 'NONE',  ( -6.505213034913038160E-19, -3.903127820947822896E-18, -1.000000000000000000 ) ) ;
#14595=ORIENTED_EDGE ( 'NONE', *, *, #15041, .F. ) ;
#14599=ORIENTED_EDGE ( 'NONE', *, *, #6654, .F. ) ;
#14600=DIRECTION ( 'NONE',  ( -1.000000000000000000, 0.000000000000000000, 0.000000000000000000 ) ) ;
#14602=CARTESIAN_POINT ( 'NONE',  ( -18.22261011550273224, -31.92986134326242365, -2.800654218530485018 ) ) ;
#14611=CARTESIAN_POINT ( 'NONE',  ( 5.093313992686365310, 32.09841355225995585, -2.999999999999971578 ) ) ;
#14612=LINE ( 'NONE', #12997, #8783 ) ;
#14619=ORIENTED_EDGE ( 'NONE', *, *, #19823, .F. ) ;
#14620=DIRECTION ( 'NONE',  ( 6.505213034913038160E-19, 3.903127820947822896E-18, 1.000000000000000000 ) ) ;
#14624=CIRCLE ( 'NONE', #4777, 19.11328065563151668 ) ;
#14635=CYLINDRICAL_SURFACE ( 'NONE', #21963, 19.11328065563152023 ) ;
#14639=DIRECTION ( 'NONE',  ( -1.209647751973867239E-17, -1.000000000000000000, 3.903127820947822896E-18 ) ) ;
#14642=DIRECTION ( 'NONE',  ( -6.505213034913038160E-19, -3.903127820947822896E-18, -1.000000000000000000 ) ) ;
#14644=EDGE_LOOP ( 'NONE', ( #8944, #10268, #3493, #20350 ) ) ;
#14647=ORIENTED_EDGE ( 'NONE', *, *, #9026, .F. ) ;
#14650=DIRECTION ( 'NONE',  ( 1.000000000000000000, 0.000000000000000000, 0.000000000000000000 ) ) ;
#14652=CARTESIAN_POINT ( 'NONE',  ( 1.110223024625156540E-13, -5.551115123125782702E-14, -6.999999999999950262 ) ) ;
#14656=CARTESIAN_POINT ( 'NONE',  ( -20.17230487860800636, -25.34312177887357365, -6.999999999999950262 ) ) ;
#14665=DIRECTION ( 'NONE',  ( -1.000000000000000000, -1.208970125616046080E-17, 6.505213034913038160E-19 ) ) ;
#14669=ADVANCED_FACE ( 'NONE', ( #1854 ), #21102, .T. ) ;
#14672=VERTEX_POINT ( 'NONE', #17649 ) ;
#14674=VERTEX_POINT ( 'NONE', #4109 ) ;
#14679=DIRECTION ( 'NONE',  ( 6.505213034913038160E-19, 3.903127820947822896E-18, 1.000000000000000000 ) ) ;
#14683=DIRECTION ( 'NONE',  ( 6.505213034913038160E-19, 3.903127820947822896E-18, 1.000000000000000000 ) ) ;
#14684=EDGE_LOOP ( 'NONE', ( #1086, #17977, #12960, #9540 ) ) ;
#14692=ORIENTED_EDGE ( 'NONE', *, *, #10938, .F. ) ;
#14695=ORIENTED_EDGE ( 'NONE', *, *, #8040, .T. ) ;
#14697=DIRECTION ( 'NONE',  ( 6.505213034913038160E-19, 3.903127820947822896E-18, 1.000000000000000000 ) ) ;
#14701=VECTOR ( 'NONE', #20695, 1000.000000000000000 ) ;
#14708=CARTESIAN_POINT ( 'NONE',  ( -14.67611967928926475, 31.67162468655990182, -2.999999999999971578 ) ) ;
#14717=CARTESIAN_POINT ( 'NONE',  ( -29.14949368109855143, 11.93972437435547640, -2.999999999999992450 ) ) ;
#14721=ORIENTED_EDGE ( 'NONE', *, *, #7964, .T. ) ;
#14726=AXIS2_PLACEMENT_3D ( 'NONE', #14132, #15751, #15636 ) ;
#14727=DIRECTION ( 'NONE',  ( -1.000000000000000000, 2.128324605523459973E-14, 0.000000000000000000 ) ) ;
#14730=CARTESIAN_POINT ( 'NONE',  ( 19.59430950039317665, -28.88846368933348074, -2.999999999999999112 ) ) ;
#14735=DIRECTION ( 'NONE',  ( -6.505213034913038160E-19, -3.903127820947822896E-18, -1.000000000000000000 ) ) ;
#14736=EDGE_CURVE ( 'NONE', #768, #13884, #17749, .T. ) ;
#14737=VERTEX_POINT ( 'NONE', #5077 ) ;
#14738=CARTESIAN_POINT ( 'NONE',  ( -19.99999999999969091, -2.554026978681552118E-14, -2.999999999999971578 ) ) ;
#14742=CIRCLE ( 'NONE', #129, 1.000000000000000888 ) ;
#14744=B_SPLINE_CURVE_WITH_KNOTS ( 'NONE', 3,
 ( #12673, #14068, #19692, #10965 ),
 .UNSPECIFIED., .F., .F.,
 ( 4, 4 ),
 ( 0.001875451646902760077, 0.003761979286331185689 ),
 .UNSPECIFIED. ) ;
#14745=DIRECTION ( 'NONE',  ( 6.505213034913038160E-19, 3.903127820947822896E-18, 1.000000000000000000 ) ) ;
#14747=CIRCLE ( 'NONE', #18425, 1.000000000000000888 ) ;
#14749=EDGE_CURVE ( 'NONE', #6570, #9329, #19234, .T. ) ;
#14750=AXIS2_PLACEMENT_3D ( 'NONE', #11794, #19030, #3099 ) ;
#14751=VERTEX_POINT ( 'NONE', #19048 ) ;
#14752=CARTESIAN_POINT ( 'NONE',  ( -17.79500259159599906, -31.47514467962714235, 2.932460736555821956 ) ) ;
#14753=AXIS2_PLACEMENT_3D ( 'NONE', #2145, #21168, #1697 ) ;
#14758=DIRECTION ( 'NONE',  ( -6.505213034913038160E-19, -3.903127820947822896E-18, -1.000000000000000000 ) ) ;
#14759=VECTOR ( 'NONE', #7672, 1000.000000000000000 ) ;
#14760=DIRECTION ( 'NONE',  ( 1.000000000000000000, 1.208970125616063490E-17, 0.000000000000000000 ) ) ;
#14764=DIRECTION ( 'NONE',  ( 1.000000000000000000, 1.208970125616053475E-17, 0.000000000000000000 ) ) ;
#14769=ORIENTED_EDGE ( 'NONE', *, *, #21359, .F. ) ;
#14771=DIRECTION ( 'NONE',  ( -6.505213034913038160E-19, -3.903127820947822896E-18, -1.000000000000000000 ) ) ;
#14777=DIRECTION ( 'NONE',  ( -1.000000000000000000, -1.208970125616081209E-17, 0.000000000000000000 ) ) ;
#14782=ADVANCED_FACE ( 'NONE', ( #7010 ), #12793, .F. ) ;
#14783=VERTEX_POINT ( 'NONE', #12161 ) ;
#14789=AXIS2_PLACEMENT_3D ( 'NONE', #17037, #15194, #10043 ) ;
#14791=EDGE_LOOP ( 'NONE', ( #18293, #3746, #5322, #20913 ) ) ;
#14793=DIRECTION ( 'NONE',  ( -6.505213034913038160E-19, -3.903127820947822896E-18, -1.000000000000000000 ) ) ;
#14805=CARTESIAN_POINT ( 'NONE',  ( -30.48934413892756368, 16.99647590252650886, -2.999999999999995559 ) ) ;
#14807=CARTESIAN_POINT ( 'NONE',  ( 27.62019382530525391, -4.341204441673157888, -2.999999999999999112 ) ) ;
#14808=AXIS2_PLACEMENT_3D ( 'NONE', #20945, #3755, #2023 ) ;
#14809=ORIENTED_EDGE ( 'NONE', *, *, #13920, .T. ) ;
#14812=ORIENTED_EDGE ( 'NONE', *, *, #15162, .F. ) ;
#14813=VERTEX_POINT ( 'NONE', #4451 ) ;
#14815=CARTESIAN_POINT ( 'NONE',  ( 2.220446049250313081E-13, -8.326672684688674053E-14, 2.800654218530498785 ) ) ;
#14817=ORIENTED_EDGE ( 'NONE', *, *, #5270, .T. ) ;
#14818=CARTESIAN_POINT ( 'NONE',  ( 2.220446049250313081E-13, -25.00000000000007816, -4.999999999999962697 ) ) ;
#14821=AXIS2_PLACEMENT_3D ( 'NONE', #9183, #17774, #2082 ) ;
#14826=DIRECTION ( 'NONE',  ( -6.505213034913038160E-19, -3.903127820947822896E-18, -1.000000000000000000 ) ) ;
#14827=CARTESIAN_POINT ( 'NONE',  ( 11.85401191286916678, 32.83234229683709771, -2.999999999999995559 ) ) ;
#14828=EDGE_CURVE ( 'NONE', #15027, #11046, #18512, .T. ) ;
#14829=CIRCLE ( 'NONE', #9725, 2.999999999999999112 ) ;
#14833=CIRCLE ( 'NONE', #4985, 22.00000000000000000 ) ;
#14834=VERTEX_POINT ( 'NONE', #11429 ) ;
#14835=ORIENTED_EDGE ( 'NONE', *, *, #10505, .F. ) ;
#14839=DIRECTION ( 'NONE',  ( -6.505213034913038160E-19, -3.903127820947822896E-18, -1.000000000000000000 ) ) ;
#14843=AXIS2_PLACEMENT_3D ( 'NONE', #4623, #13288, #20764 ) ;
#14845=DIRECTION ( 'NONE',  ( -1.000000000000000000, -1.208970125616081209E-17, 0.000000000000000000 ) ) ;
#14846=CIRCLE ( 'NONE', #2809, 19.11328065563152379 ) ;
#14847=DIRECTION ( 'NONE',  ( 6.505213034913038160E-19, 3.903127820947822896E-18, 1.000000000000000000 ) ) ;
#14850=ORIENTED_EDGE ( 'NONE', *, *, #11406, .T. ) ;
#14851=CARTESIAN_POINT ( 'NONE',  ( -35.99819890246949683, 7.463862311151203244, -2.800654218530485018 ) ) ;
#14853=CARTESIAN_POINT ( 'NONE',  ( 30.60042966911727547, 7.474202570536048640, -6.999999999999950262 ) ) ;
#14855=CIRCLE ( 'NONE', #1715, 19.11328065563151313 ) ;
#14856=EDGE_LOOP ( 'NONE', ( #5754, #14246, #21195, #10756, #16253, #4162 ) ) ;
#14857=FACE_OUTER_BOUND ( 'NONE', #7570, .T. ) ;
#14858=DIRECTION ( 'NONE',  ( 6.505213034913038160E-19, 3.903127820947822896E-18, 1.000000000000000000 ) ) ;
#14860=ORIENTED_EDGE ( 'NONE', *, *, #12408, .T. ) ;
#14861=AXIS2_PLACEMENT_3D ( 'NONE', #327, #7318, #14283 ) ;
#14862=DIRECTION ( 'NONE',  ( -1.000000000000000000, -1.208970125616044077E-17, 0.000000000000000000 ) ) ;
#14865=ORIENTED_EDGE ( 'NONE', *, *, #12096, .F. ) ;
#14867=CIRCLE ( 'NONE', #22594, 36.76383501243555685 ) ;
#14870=DIRECTION ( 'NONE',  ( -6.505213034913038160E-19, -3.903127820947822896E-18, -1.000000000000000000 ) ) ;
#14876=DIRECTION ( 'NONE',  ( 6.505213034913038160E-19, 3.903127820947822896E-18, 1.000000000000000000 ) ) ;
#14879=DIRECTION ( 'NONE',  ( 6.505213034913038160E-19, 3.903127820947822896E-18, 1.000000000000000000 ) ) ;
#14883=DIRECTION ( 'NONE',  ( -6.505213034913038160E-19, -3.903127820947822896E-18, -1.000000000000000000 ) ) ;
#14890=VERTEX_POINT ( 'NONE', #5931 ) ;
#14894=CYLINDRICAL_SURFACE ( 'NONE', #17240, 0.9999999999999974465 ) ;
#14900=CARTESIAN_POINT ( 'NONE',  ( 35.16985127952418111, 10.70799354677351367, -2.800654218530464146 ) ) ;
#14901=EDGE_LOOP ( 'NONE', ( #12769, #16053, #162, #18986 ) ) ;
#14904=DIRECTION ( 'NONE',  ( -1.000000000000000000, -1.208970125616060101E-17, 6.505213034913038160E-19 ) ) ;
#14907=EDGE_LOOP ( 'NONE', ( #13808, #20948, #13686, #1354 ) ) ;
#14908=CARTESIAN_POINT ( 'NONE',  ( 32.20238537491815123, 4.080045426412798548, 2.999999999999995559 ) ) ;
#14911=ORIENTED_EDGE ( 'NONE', *, *, #8775, .T. ) ;
#14916=AXIS2_PLACEMENT_3D ( 'NONE', #9517, #16497, #803 ) ;
#14918=CIRCLE ( 'NONE', #10528, 1.000000000000000888 ) ;
#14920=EDGE_CURVE ( 'NONE', #6602, #21037, #5698, .T. ) ;
#14921=CARTESIAN_POINT ( 'NONE',  ( -7.094908322883119567, 35.33352588067079125, -2.999999999999971578 ) ) ;
#14924=VERTEX_POINT ( 'NONE', #4340 ) ;
#14927=ORIENTED_EDGE ( 'NONE', *, *, #1518, .T. ) ;
#14933=DIRECTION ( 'NONE',  ( 1.000000000000000000, 0.000000000000000000, 0.000000000000000000 ) ) ;
#14941=CARTESIAN_POINT ( 'NONE',  ( 2.775557561562891351E-14, 2.775557561562891351E-14, 5.750000000000001776 ) ) ;
#14942=EDGE_CURVE ( 'NONE', #4779, #8231, #14829, .T. ) ;
#14946=CARTESIAN_POINT ( 'NONE',  ( 2.220446049250313081E-13, -2.498001805406602216E-13, -6.859353255829918616 ) ) ;
#14947=EDGE_CURVE ( 'NONE', #3371, #384, #10067, .T. ) ;
#14951=VERTEX_POINT ( 'NONE', #1224 ) ;
#14957=FACE_OUTER_BOUND ( 'NONE', #21060, .T. ) ;
#14958=CARTESIAN_POINT ( 'NONE',  ( 33.51030287062395274, 15.12081897056660651, 2.800654218530485018 ) ) ;
#14966=DIRECTION ( 'NONE',  ( -1.000000000000000000, 0.000000000000000000, 0.000000000000000000 ) ) ;
#14975=CARTESIAN_POINT ( 'NONE',  ( 16.56444186175109934, -26.79308242454903066, 3.000000000000023537 ) ) ;
#14977=ADVANCED_FACE ( 'NONE', ( #6848 ), #10151, .F. ) ;
#14981=EDGE_CURVE ( 'NONE', #5071, #2772, #5017, .T. ) ;
#14986=DIRECTION ( 'NONE',  ( 6.505213034913038160E-19, 3.903127820947822896E-18, 1.000000000000000000 ) ) ;
#14988=CARTESIAN_POINT ( 'NONE',  ( 31.92986134326236680, -18.22261011550291343, -2.800654218530485018 ) ) ;
#14989=EDGE_LOOP ( 'NONE', ( #13864, #10558, #11068, #1306 ) ) ;
#14992=LINE ( 'NONE', #7491, #9136 ) ;
#15000=CARTESIAN_POINT ( 'NONE',  ( 4.936596639065399472, 31.11077005834403408, 2.999999999999995559 ) ) ;
#15002=ORIENTED_EDGE ( 'NONE', *, *, #16145, .T. ) ;
#15012=CYLINDRICAL_SURFACE ( 'NONE', #9078, 1.000000000000000888 ) ;
#15016=VERTEX_POINT ( 'NONE', #13468 ) ;
#15021=ORIENTED_EDGE ( 'NONE', *, *, #9333, .F. ) ;
#15027=VERTEX_POINT ( 'NONE', #17256 ) ;
#15030=CARTESIAN_POINT ( 'NONE',  ( -21.97438720605733664, 22.98755168577401520, -2.999999999999971578 ) ) ;
#15036=ORIENTED_EDGE ( 'NONE', *, *, #2752, .F. ) ;
#15037=DIRECTION ( 'NONE',  ( -1.000000000000000000, -1.208970125616077665E-17, 0.000000000000000000 ) ) ;
#15040=CIRCLE ( 'NONE', #16133, 19.11328065563151668 ) ;
#15041=EDGE_CURVE ( 'NONE', #2190, #7646, #1343, .T. ) ;
#15043=CARTESIAN_POINT ( 'NONE',  ( -29.36548507648009831, -13.83143812983123055, 2.999999999999995559 ) ) ;
#15045=ORIENTED_EDGE ( 'NONE', *, *, #20076, .T. ) ;
#15046=LINE ( 'NONE', #15277, #16487 ) ;
#15048=ORIENTED_EDGE ( 'NONE', *, *, #20012, .T. ) ;
#15051=CARTESIAN_POINT ( 'NONE',  ( 2.775557561562891351E-14, -2.775557561562891351E-14, 2.999999999999999112 ) ) ;
#15056=DIRECTION ( 'NONE',  ( -1.000000000000000000, -1.815202222194849261E-15, 0.000000000000000000 ) ) ;
#15057=ORIENTED_EDGE ( 'NONE', *, *, #2741, .T. ) ;
#15058=ORIENTED_EDGE ( 'NONE', *, *, #1553, .T. ) ;
#15059=EDGE_CURVE ( 'NONE', #22419, #13252, #12996, .T. ) ;
#15062=DIRECTION ( 'NONE',  ( 1.266830946243004623E-16, -1.000000000000000000, -3.903127820947817503E-18 ) ) ;
#15063=DIRECTION ( 'NONE',  ( 1.000000000000000000, 0.000000000000000000, 0.000000000000000000 ) ) ;
#15069=CARTESIAN_POINT ( 'NONE',  ( 4.918774254216024211, -31.11359284679388182, 2.999999999999995559 ) ) ;
#15070=DIRECTION ( 'NONE',  ( -6.505213034913038160E-19, -3.903127820947822896E-18, -1.000000000000000000 ) ) ;
#15074=CARTESIAN_POINT ( 'NONE',  ( 3.330669073875469621E-13, -1.110223024625156540E-13, -2.999999999999971578 ) ) ;
#15082=EDGE_LOOP ( 'NONE', ( #17491, #5335, #12110, #17294, #1762, #10232 ) ) ;
#15084=CIRCLE ( 'NONE', #16195, 34.90673715956759082 ) ;
#15088=DIRECTION ( 'NONE',  ( 1.000000000000000000, 0.000000000000000000, 0.000000000000000000 ) ) ;
#15097=CARTESIAN_POINT ( 'NONE',  ( -35.99819890246936893, 7.463862311150981199, -1.999999999999984457 ) ) ;
#15098=VERTEX_POINT ( 'NONE', #1809 ) ;
#15105=EDGE_CURVE ( 'NONE', #8849, #312, #10807, .T. ) ;
#15106=VERTEX_POINT ( 'NONE', #3647 ) ;
#15108=CARTESIAN_POINT ( 'NONE',  ( -21.41958700883257904, -27.56232195404059837, -2.999999999999992450 ) ) ;
#15109=EDGE_CURVE ( 'NONE', #16547, #14672, #15763, .T. ) ;
#15112=EDGE_LOOP ( 'NONE', ( #12276, #5182, #10103, #22444 ) ) ;
#15117=ORIENTED_EDGE ( 'NONE', *, *, #9619, .F. ) ;
#15119=DIRECTION ( 'NONE',  ( -6.505213034913038160E-19, -3.903127820947822896E-18, -1.000000000000000000 ) ) ;
#15120=CARTESIAN_POINT ( 'NONE',  ( -27.56232195404058416, 21.41958700883256483, 2.999999999999995559 ) ) ;
#15127=CARTESIAN_POINT ( 'NONE',  ( 2.775557561562891351E-14, -2.775557561562891351E-14, 2.999999999999999112 ) ) ;
#15130=CIRCLE ( 'NONE', #5278, 36.76383501243555685 ) ;
#15135=DIRECTION ( 'NONE',  ( 6.505213034913038160E-19, 3.903127820947822896E-18, 1.000000000000000000 ) ) ;
#15140=CARTESIAN_POINT ( 'NONE',  ( -28.07080038625073115, -14.29266125237904639, -2.999999999999981792 ) ) ;
#15144=ORIENTED_EDGE ( 'NONE', *, *, #4213, .T. ) ;
#15148=EDGE_LOOP ( 'NONE', ( #16911, #11494, #21712, #1643, #9863, #11737 ) ) ;
#15151=DIRECTION ( 'NONE',  ( -1.000000000000000000, -9.002681209562840861E-16, 0.000000000000000000 ) ) ;
#15153=ORIENTED_EDGE ( 'NONE', *, *, #11296, .F. ) ;
#15155=CARTESIAN_POINT ( 'NONE',  ( 18.00000000000035882, -2.752196816394091375E-14, -4.999999999999997335 ) ) ;
#15158=CARTESIAN_POINT ( 'NONE',  ( 21.41958700883261812, 27.56232195404056995, -2.999999999999995559 ) ) ;
#15159=ORIENTED_EDGE ( 'NONE', *, *, #5747, .T. ) ;
#15161=CARTESIAN_POINT ( 'NONE',  ( -17.09029715894913437, 27.64365646977270785, 3.000000000000012879 ) ) ;
#15162=EDGE_CURVE ( 'NONE', #20565, #14456, #1266, .T. ) ;
#15163=CARTESIAN_POINT ( 'NONE',  ( 28.88846368933370456, 19.59430950039303809, -2.999999999999975131 ) ) ;
#15166=FACE_OUTER_BOUND ( 'NONE', #18381, .T. ) ;
#15167=ORIENTED_EDGE ( 'NONE', *, *, #12938, .T. ) ;
#15168=ORIENTED_EDGE ( 'NONE', *, *, #12349, .F. ) ;
#15170=VERTEX_POINT ( 'NONE', #10827 ) ;
#15172=FACE_OUTER_BOUND ( 'NONE', #21334, .T. ) ;
#15173=VECTOR ( 'NONE', #16844, 1000.000000000000000 ) ;
#15174=ADVANCED_FACE ( 'NONE', ( #299 ), #10444, .T. ) ;
#15176=CYLINDRICAL_SURFACE ( 'NONE', #5995, 0.9999999999999956701 ) ;
#15177=VECTOR ( 'NONE', #9882, 1000.000000000000000 ) ;
#15178=CYLINDRICAL_SURFACE ( 'NONE', #20359, 36.76383501243555685 ) ;
#15179=ORIENTED_EDGE ( 'NONE', *, *, #21113, .F. ) ;
#15183=CYLINDRICAL_SURFACE ( 'NONE', #16000, 19.11328065563150957 ) ;
#15191=AXIS2_PLACEMENT_3D ( 'NONE', #16559, #21848, #13325 ) ;
#15194=DIRECTION ( 'NONE',  ( -6.505213034913038160E-19, -3.903127820947822896E-18, -1.000000000000000000 ) ) ;
#15206=VECTOR ( 'NONE', #12385, 1000.000000000000000 ) ;
#15207=EDGE_LOOP ( 'NONE', ( #8637, #3512, #22540, #20586 ) ) ;
#15208=B_SPLINE_CURVE_WITH_KNOTS ( 'NONE', 3,
 ( #12392, #1415, #6793, #20657 ),
 .UNSPECIFIED., .F., .F.,
 ( 4, 4 ),
 ( 9.715086429499893182E-07, 0.001929643240674650765 ),
 .UNSPECIFIED. ) ;
#15209=AXIS2_PLACEMENT_3D ( 'NONE', #17739, #7092, #10292 ) ;
#15211=DIRECTION ( 'NONE',  ( -6.505213034913038160E-19, -3.903127820947822896E-18, -1.000000000000000000 ) ) ;
#15217=VERTEX_POINT ( 'NONE', #17942 ) ;
#15220=DIRECTION ( 'NONE',  ( -1.000000000000000000, 0.000000000000000000, 0.000000000000000000 ) ) ;
#15221=CARTESIAN_POINT ( 'NONE',  ( -35.92356703407480012, -4.104166344909336850, 2.932460736555823733 ) ) ;
#15224=EDGE_CURVE ( 'NONE', #21131, #5874, #18147, .T. ) ;
#15225=CARTESIAN_POINT ( 'NONE',  ( -34.74700806321090596, 12.00937115242645170, 2.800654218530481465 ) ) ;
#15227=AXIS2_PLACEMENT_3D ( 'NONE', #13496, #11686, #20511 ) ;
#15228=EDGE_CURVE ( 'NONE', #15404, #2168, #19246, .T. ) ;
#15230=AXIS2_PLACEMENT_3D ( 'NONE', #19114, #10381, #17379 ) ;
#15232=ORIENTED_EDGE ( 'NONE', *, *, #22535, .T. ) ;
#15235=CARTESIAN_POINT ( 'NONE',  ( 2.775557561562891351E-14, -2.775557561562891351E-14, 2.999999999999999112 ) ) ;
#15236=CARTESIAN_POINT ( 'NONE',  ( 22.26748298433281548, -22.28024240313505899, 2.999999999999995559 ) ) ;
#15238=AXIS2_PLACEMENT_3D ( 'NONE', #16527, #11371, #14904 ) ;
#15239=ORIENTED_EDGE ( 'NONE', *, *, #19588, .F. ) ;
#15244=AXIS2_PLACEMENT_3D ( 'NONE', #8559, #13815, #18026 ) ;
#15247=DIRECTION ( 'NONE',  ( -6.505213034913038160E-19, -3.903127820947822896E-18, -1.000000000000000000 ) ) ;
#15251=ORIENTED_EDGE ( 'NONE', *, *, #22148, .F. ) ;
#15252=DIRECTION ( 'NONE',  ( -1.000000000000000000, -1.208970125616046080E-17, 6.505213034913038160E-19 ) ) ;
#15254=ORIENTED_EDGE ( 'NONE', *, *, #6804, .T. ) ;
#15261=CIRCLE ( 'NONE', #8341, 27.99999999999999645 ) ;
#15262=CIRCLE ( 'NONE', #10882, 0.9999999999999974465 ) ;
#15264=ORIENTED_EDGE ( 'NONE', *, *, #6055, .T. ) ;
#15265=ORIENTED_EDGE ( 'NONE', *, *, #17589, .T. ) ;
#15267=EDGE_CURVE ( 'NONE', #13925, #5266, #22543, .T. ) ;
#15269=CARTESIAN_POINT ( 'NONE',  ( 21.41958700883261812, 27.56232195404056995, -2.999999999999995559 ) ) ;
#15270=DIRECTION ( 'NONE',  ( 1.000000000000000000, 0.000000000000000000, 0.000000000000000000 ) ) ;
#15273=ORIENTED_EDGE ( 'NONE', *, *, #1472, .F. ) ;
#15274=DIRECTION ( 'NONE',  ( -6.505213034913038160E-19, -3.903127820947822896E-18, -1.000000000000000000 ) ) ;
#15277=CARTESIAN_POINT ( 'NONE',  ( -2.347663744114242057, -31.41239365194231681, -6.999999999999950262 ) ) ;
#15279=ORIENTED_EDGE ( 'NONE', *, *, #11396, .F. ) ;
#15281=AXIS2_PLACEMENT_3D ( 'NONE', #15306, #20706, #20375 ) ;
#15282=CARTESIAN_POINT ( 'NONE',  ( 32.83234229683737482, -11.85401191286897316, -2.999999999999971578 ) ) ;
#15283=DIRECTION ( 'NONE',  ( -6.505213034913038160E-19, -3.903127820947822896E-18, -1.000000000000000000 ) ) ;
#15284=CARTESIAN_POINT ( 'NONE',  ( -36.54278193890295512, -4.025500340002762911, -2.800654218530457484 ) ) ;
#15287=TOROIDAL_SURFACE ( 'NONE', #22638, 34.90673715956759082, 8.750000000000000000 ) ;
#15288=VERTEX_POINT ( 'NONE', #20127 ) ;
#15289=TOROIDAL_SURFACE ( 'NONE', #18234, 34.90673715956759082, 8.750000000000000000 ) ;
#15290=ORIENTED_EDGE ( 'NONE', *, *, #13287, .T. ) ;
#15291=CIRCLE ( 'NONE', #17857, 31.50000000000001421 ) ;
#15293=EDGE_CURVE ( 'NONE', #2580, #16652, #17778, .T. ) ;
#15294=CIRCLE ( 'NONE', #6532, 34.90673715956759082 ) ;
#15297=CARTESIAN_POINT ( 'NONE',  ( 3.608224830031758756E-13, -2.775557561562891351E-14, -4.999999999999997335 ) ) ;
#15306=CARTESIAN_POINT ( 'NONE',  ( -22.97438720605751783, 22.98755168577401520, 3.000000000000023537 ) ) ;
#15307=CARTESIAN_POINT ( 'NONE',  ( -4.918774254215691144, 31.11359284679385340, -7.000000000000006217 ) ) ;
#15318=EDGE_CURVE ( 'NONE', #15629, #2277, #11525, .T. ) ;
#15322=DIRECTION ( 'NONE',  ( -6.505213034913038160E-19, -3.903127820947822896E-18, -1.000000000000000000 ) ) ;
#15324=FACE_OUTER_BOUND ( 'NONE', #7307, .T. ) ;
#15333=STYLED_ITEM('',(#22748),#18090);
#15334=ORIENTED_EDGE ( 'NONE', *, *, #20251, .F. ) ;
#15343=CIRCLE ( 'NONE', #3306, 36.76383501243555685 ) ;
#15344=EDGE_LOOP ( 'NONE', ( #10377, #14860 ) ) ;
#15350=DIRECTION ( 'NONE',  ( -1.000000000000000000, 7.725943281265459575E-14, 0.000000000000000000 ) ) ;
#15356=ORIENTED_EDGE ( 'NONE', *, *, #3537, .F. ) ;
#15364=DIRECTION ( 'NONE',  ( 6.505213034913038160E-19, 3.903127820947822896E-18, 1.000000000000000000 ) ) ;
#15365=VERTEX_POINT ( 'NONE', #7635 ) ;
#15368=VERTEX_POINT ( 'NONE', #16453 ) ;
#15369=DIRECTION ( 'NONE',  ( -1.000000000000000000, 0.000000000000000000, 0.000000000000000000 ) ) ;
#15370=CARTESIAN_POINT ( 'NONE',  ( -32.09841355225970005, 5.093313992686226754, 2.999999999999995559 ) ) ;
#15371=ORIENTED_EDGE ( 'NONE', *, *, #8448, .T. ) ;
#15377=CIRCLE ( 'NONE', #9158, 22.00000000000000000 ) ;
#15390=ORIENTED_EDGE ( 'NONE', *, *, #15990, .T. ) ;
#15391=CARTESIAN_POINT ( 'NONE',  ( 35.16985127952398926, 10.70799354677376414, -2.000000000000001776 ) ) ;
#15392=CARTESIAN_POINT ( 'NONE',  ( -26.50842683089750551, 24.41514043009179602, -7.000000000000006217 ) ) ;
#15398=CARTESIAN_POINT ( 'NONE',  ( -17.99999999999963762, -2.576882599977457532E-14, -4.999999999999997335 ) ) ;
#15399=EDGE_LOOP ( 'NONE', ( #12934, #13744, #3566, #13565, #19923 ) ) ;
#15400=EDGE_CURVE ( 'NONE', #2388, #1875, #1319, .T. ) ;
#15401=AXIS2_PLACEMENT_3D ( 'NONE', #6552, #4494, #9971 ) ;
#15404=VERTEX_POINT ( 'NONE', #15622 ) ;
#15409=B_SPLINE_CURVE_WITH_KNOTS ( 'NONE', 3,
 ( #10714, #1916, #8897, #15873 ),
 .UNSPECIFIED., .F., .F.,
 ( 4, 4 ),
 ( 0.001875451646902967593, 0.003761979286331313191 ),
 .UNSPECIFIED. ) ;
#15410=ORIENTED_EDGE ( 'NONE', *, *, #21649, .T. ) ;
#15414=DIRECTION ( 'NONE',  ( 1.000000000000000000, 1.208970125616045926E-17, 0.000000000000000000 ) ) ;
#15420=ORIENTED_EDGE ( 'NONE', *, *, #16979, .F. ) ;
#15433=EDGE_CURVE ( 'NONE', #21019, #15288, #19305, .T. ) ;
#15435=CARTESIAN_POINT ( 'NONE',  ( -30.07487443287951123, 12.31876324338268525, 3.000000000000023537 ) ) ;
#15439=ORIENTED_EDGE ( 'NONE', *, *, #20302, .T. ) ;
#15444=EDGE_CURVE ( 'NONE', #13122, #1817, #4807, .T. ) ;
#15446=CIRCLE ( 'NONE', #1562, 0.9999999999999974465 ) ;
#15450=CIRCLE ( 'NONE', #18393, 1.000000000000000888 ) ;
#15453=EDGE_CURVE ( 'NONE', #18082, #1931, #7163, .T. ) ;
#15455=ORIENTED_EDGE ( 'NONE', *, *, #20926, .F. ) ;
#15457=DIRECTION ( 'NONE',  ( 6.505213034913038160E-19, 3.903127820947822896E-18, 1.000000000000000000 ) ) ;
#15461=EDGE_CURVE ( 'NONE', #2202, #16547, #11551, .T. ) ;
#15463=ORIENTED_EDGE ( 'NONE', *, *, #6306, .T. ) ;
#15466=CARTESIAN_POINT ( 'NONE',  ( -1.423424233832598640, -32.35999952201590446, -2.999999999999971578 ) ) ;
#15473=VERTEX_POINT ( 'NONE', #4774 ) ;
#15477=EDGE_CURVE ( 'NONE', #12921, #14751, #1679, .T. ) ;
#15482=DIRECTION ( 'NONE',  ( -6.505213034913038160E-19, -3.903127820947822896E-18, -1.000000000000000000 ) ) ;
#15491=DIRECTION ( 'NONE',  ( 0.000000000000000000, 0.000000000000000000, 1.000000000000000000 ) ) ;
#15493=DIRECTION ( 'NONE',  ( 6.505213034913038160E-19, 3.903127820947822896E-18, 1.000000000000000000 ) ) ;
#15497=ORIENTED_EDGE ( 'NONE', *, *, #21239, .F. ) ;
#15501=AXIS2_PLACEMENT_3D ( 'NONE', #12894, #14839, #21396 ) ;
#15502=FACE_OUTER_BOUND ( 'NONE', #8216, .T. ) ;
#15505=CARTESIAN_POINT ( 'NONE',  ( 34.74700806321118307, -12.00937115242653519, -2.800654218530457484 ) ) ;
#15506=CARTESIAN_POINT ( 'NONE',  ( 30.13956425491259949, 21.05198877411795877, -2.800654218530485018 ) ) ;
#15509=LINE ( 'NONE', #8534, #19142 ) ;
#15511=CARTESIAN_POINT ( 'NONE',  ( 10.70799354677381920, -35.16985127952404611, -2.800654218530477912 ) ) ;
#15512=EDGE_LOOP ( 'NONE', ( #8569, #18021, #14039, #1885, #4071, #21147, #11328, #6741, #16461, #7928, #684, #20315, #18916, #16067, #6486, #12317, #6930, #8257, #13449, #11305, #18277, #20133, #16414, #3814, #7884, #4169, #17631, #8278, #16631, #15708, #20487, #2554, #16223, #16207, #21642, #17420, #20336, #2086, #7126, #22596, #9018, #8092, #10250, #19956, #20674, #11370, #9553, #3247, #12119, #15972, #3108, #12014, #10294, #15251, #3451, #4550, #12826, #18342, #12728, #22146, #21117, #8732, #18805, #8710, #4317, #18478, #4175, #21128, #3543, #6465, #21342, #17285, #15153, #11999, #2707, #17442, #6947, #13662, #11791, #13452, #1410, #7966, #5641, #7037, #20417, #14692, #618, #17782, #11860, #13600, #19771, #1229, #12201, #9998, #19850, #20538, #9138, #8352, #15905, #5727, #16946, #11147, #9175, #3777, #16658, #6781, #19207, #17375, #5123, #17519, #21459, #827, #2584, #20772, #13908, #2282, #16374, #21878, #15356, #21395, #21832, #13910, #19387, #9858, #19396, #5151, #14412, #9188, #795, #20442, #6346 ) ) ;
#15513=ORIENTED_EDGE ( 'NONE', *, *, #16230, .T. ) ;
#15514=ADVANCED_FACE ( 'NONE', ( #1547 ), #10440, .T. ) ;
#15516=CIRCLE ( 'NONE', #9685, 1.000000000000000888 ) ;
#15517=ORIENTED_EDGE ( 'NONE', *, *, #2163, .T. ) ;
#15519=CARTESIAN_POINT ( 'NONE',  ( -11.93772187171643040, -33.46652738560690921, -2.999999999999999112 ) ) ;
#15521=DIRECTION ( 'NONE',  ( -1.000000000000000000, 0.000000000000000000, 0.000000000000000000 ) ) ;
#15523=ORIENTED_EDGE ( 'NONE', *, *, #21829, .T. ) ;
#15524=TOROIDAL_SURFACE ( 'NONE', #8946, 34.90673715956759082, 8.750000000000000000 ) ;
#15532=CARTESIAN_POINT ( 'NONE',  ( 28.06260833510309993, -14.30873905802335067, 3.000000000000006217 ) ) ;
#15535=DIRECTION ( 'NONE',  ( 6.505213034913038160E-19, 3.903127820947822896E-18, 1.000000000000000000 ) ) ;
#15536=FACE_OUTER_BOUND ( 'NONE', #1158, .T. ) ;
#15537=DIRECTION ( 'NONE',  ( -6.505213034913038160E-19, -3.903127820947822896E-18, -1.000000000000000000 ) ) ;
#15540=ORIENTED_EDGE ( 'NONE', *, *, #21889, .T. ) ;
#15553=DIRECTION ( 'NONE',  ( 6.505213034913038160E-19, 3.903127820947822896E-18, 1.000000000000000000 ) ) ;
#15561=DIRECTION ( 'NONE',  ( -1.000000000000000000, -1.208970125616077665E-17, 0.000000000000000000 ) ) ;
#15564=DIRECTION ( 'NONE',  ( -6.505213034913038160E-19, -3.903127820947822896E-18, -1.000000000000000000 ) ) ;
#15566=EDGE_CURVE ( 'NONE', #104, #6092, #6069, .T. ) ;
#15568=AXIS2_PLACEMENT_3D ( 'NONE', #17578, #13996, #21025 ) ;
#15569=AXIS2_PLACEMENT_3D ( 'NONE', #17807, #16078, #19647 ) ;
#15570=B_SPLINE_CURVE_WITH_KNOTS ( 'NONE', 3,
 ( #18866, #61, #2009, #8543 ),
 .UNSPECIFIED., .F., .F.,
 ( 4, 4 ),
 ( 9.545285770191642639E-07, 0.001900595205834596261 ),
 .UNSPECIFIED. ) ;
#15573=ORIENTED_EDGE ( 'NONE', *, *, #14020, .F. ) ;
#15574=CARTESIAN_POINT ( 'NONE',  ( 6.742883674876798850, 34.24928931925766307, 2.999999999999999112 ) ) ;
#15576=CARTESIAN_POINT ( 'NONE',  ( 36.14854559161371128, -0.8615617109689401865, -2.932164912090503339 ) ) ;
#15577=CARTESIAN_POINT ( 'NONE',  ( -17.66631876130896117, 31.41173278719219653, 3.000000000000016431 ) ) ;
#15591=AXIS2_PLACEMENT_3D ( 'NONE', #13627, #6668, #1513 ) ;
#15592=AXIS2_PLACEMENT_3D ( 'NONE', #735, #7293, #14139 ) ;
#15595=DIRECTION ( 'NONE',  ( 6.505213034913038160E-19, 3.903127820947822896E-18, 1.000000000000000000 ) ) ;
#15596=CARTESIAN_POINT ( 'NONE',  ( -14.30873905802322632, -28.06260833510312835, 2.999999999999995559 ) ) ;
#15613=EDGE_LOOP ( 'NONE', ( #20549, #16881, #18320, #7782 ) ) ;
#15616=VERTEX_POINT ( 'NONE', #13997 ) ;
#15622=CARTESIAN_POINT ( 'NONE',  ( -16.99647590252643781, -30.48934413892778750, -2.999999999999992450 ) ) ;
#15626=CARTESIAN_POINT ( 'NONE',  ( 25.58633464742632313, 23.74488952252767859, -2.999999999999971578 ) ) ;
#15627=CIRCLE ( 'NONE', #3580, 18.00000000000000000 ) ;
#15629=VERTEX_POINT ( 'NONE', #21026 ) ;
#15633=ORIENTED_EDGE ( 'NONE', *, *, #17163, .T. ) ;
#15635=DIRECTION ( 'NONE',  ( 6.505213034913038160E-19, 3.903127820947822896E-18, 1.000000000000000000 ) ) ;
#15636=DIRECTION ( 'NONE',  ( 1.000000000000000000, 0.000000000000000000, 0.000000000000000000 ) ) ;
#15639=CIRCLE ( 'NONE', #1370, 31.50000000000000711 ) ;
#15641=DIRECTION ( 'NONE',  ( -1.000000000000000000, 0.000000000000000000, 0.000000000000000000 ) ) ;
#15644=ADVANCED_FACE ( 'NONE', ( #10799 ), #10464, .T. ) ;
#15646=ORIENTED_EDGE ( 'NONE', *, *, #12524, .F. ) ;
#15647=CARTESIAN_POINT ( 'NONE',  ( 30.07487443287978834, -12.31876324338301920, 3.000000000000023537 ) ) ;
#15650=DIRECTION ( 'NONE',  ( 1.208970125616062874E-17, -1.000000000000000000, 3.903127820947822896E-18 ) ) ;
#15651=CARTESIAN_POINT ( 'NONE',  ( 27.64365646977287483, 17.09029715894919121, -2.999999999999975131 ) ) ;
#15655=AXIS2_PLACEMENT_3D ( 'NONE', #19187, #41, #13657 ) ;
#15656=AXIS2_PLACEMENT_3D ( 'NONE', #10755, #21661, #5505 ) ;
#15661=CIRCLE ( 'NONE', #16775, 0.9999999999999991118 ) ;
#15663=ORIENTED_EDGE ( 'NONE', *, *, #20748, .F. ) ;
#15665=CARTESIAN_POINT ( 'NONE',  ( -6.742883674876437361, -34.24928931925796860, 3.000000000000002665 ) ) ;
#15681=CARTESIAN_POINT ( 'NONE',  ( -9.576564013118820995, 26.31139338200511091, 2.999999999999999112 ) ) ;
#15685=DIRECTION ( 'NONE',  ( 6.505213034913038160E-19, 3.903127820947822896E-18, 1.000000000000000000 ) ) ;
#15687=VECTOR ( 'NONE', #3689, 1000.000000000000000 ) ;
#15689=PRODUCT_DEFINITION_FORMATION_WITH_SPECIFIED_SOURCE ( 'ANY', '', #10941, .NOT_KNOWN. ) ;
#15701=EDGE_LOOP ( 'NONE', ( #898, #11183, #6221, #16977, #17577, #12204 ) ) ;
#15708=ORIENTED_EDGE ( 'NONE', *, *, #22073, .F. ) ;
#15710=DIRECTION ( 'NONE',  ( 6.505213034913038160E-19, 3.903127820947822896E-18, 1.000000000000000000 ) ) ;
#15714=ADVANCED_FACE ( 'NONE', ( #11496 ), #14111, .T. ) ;
#15715=CIRCLE ( 'NONE', #21596, 36.76383501243555685 ) ;
#15719=ORIENTED_EDGE ( 'NONE', *, *, #22469, .T. ) ;
#15721=CARTESIAN_POINT ( 'NONE',  ( 1.665334536937734811E-13, 2.999999999999780620, 5.000000000000022204 ) ) ;
#15729=CYLINDRICAL_SURFACE ( 'NONE', #6623, 31.50000000000000711 ) ;
#15734=EDGE_CURVE ( 'NONE', #22134, #2949, #1489, .T. ) ;
#15742=EDGE_CURVE ( 'NONE', #13563, #18413, #12646, .T. ) ;
#15745=CYLINDRICAL_SURFACE ( 'NONE', #8204, 19.11328065563151668 ) ;
#15747=VERTEX_POINT ( 'NONE', #1256 ) ;
#15749=ORIENTED_EDGE ( 'NONE', *, *, #10885, .F. ) ;
#15751=DIRECTION ( 'NONE',  ( 6.505213034913038160E-19, 3.903127820947822896E-18, 1.000000000000000000 ) ) ;
#15753=AXIS2_PLACEMENT_3D ( 'NONE', #14366, #4313, #10821 ) ;
#15756=B_SPLINE_CURVE_WITH_KNOTS ( 'NONE', 3,
 ( #19764, #3727, #4070, #3952 ),
 .UNSPECIFIED., .F., .F.,
 ( 4, 4 ),
 ( 9.545285771901622165E-07, 0.001900595205834791634 ),
 .UNSPECIFIED. ) ;
#15763=LINE ( 'NONE', #19674, #6060 ) ;
#15774=DIRECTION ( 'NONE',  ( -6.505213034913038160E-19, -3.903127820947822896E-18, -1.000000000000000000 ) ) ;
#15779=CARTESIAN_POINT ( 'NONE',  ( -35.99819890246953946, 7.463862311151231665, 2.800654218530509443 ) ) ;
#15788=DIRECTION ( 'NONE',  ( -6.505213034913038160E-19, -3.903127820947822896E-18, -1.000000000000000000 ) ) ;
#15789=CARTESIAN_POINT ( 'NONE',  ( 3.330669073875469621E-13, -1.110223024625156540E-13, -2.999999999999971578 ) ) ;
#15790=EDGE_CURVE ( 'NONE', #5071, #15629, #19619, .T. ) ;
#15792=EDGE_LOOP ( 'NONE', ( #7168, #14371, #15821, #13656 ) ) ;
#15798=DIRECTION ( 'NONE',  ( -1.000000000000000000, -1.208970125616060101E-17, 6.505213034913038160E-19 ) ) ;
#15801=CARTESIAN_POINT ( 'NONE',  ( 12.31876324338274031, 30.07487443287973505, -2.999999999999999112 ) ) ;
#15804=DIRECTION ( 'NONE',  ( -6.505213034913038160E-19, -3.903127820947822896E-18, -1.000000000000000000 ) ) ;
#15811=VERTEX_POINT ( 'NONE', #9861 ) ;
#15812=DIRECTION ( 'NONE',  ( 1.000000000000000000, 1.208970125616186904E-17, 0.000000000000000000 ) ) ;
#15818=ORIENTED_EDGE ( 'NONE', *, *, #1866, .T. ) ;
#15821=ORIENTED_EDGE ( 'NONE', *, *, #2716, .T. ) ;
#15826=DIRECTION ( 'NONE',  ( -1.000000000000000000, -1.208970125616060717E-17, 0.000000000000000000 ) ) ;
#15834=DIRECTION ( 'NONE',  ( -1.000000000000000000, 0.000000000000000000, 0.000000000000000000 ) ) ;
#15836=DIRECTION ( 'NONE',  ( 6.505213034913038160E-19, 3.903127820947822896E-18, 1.000000000000000000 ) ) ;
#15841=CIRCLE ( 'NONE', #18402, 27.99999999999999645 ) ;
#15848=AXIS2_PLACEMENT_3D ( 'NONE', #2601, #11178, #2370 ) ;
#15851=AXIS2_PLACEMENT_3D ( 'NONE', #5675, #7739, #859 ) ;
#15854=DIRECTION ( 'NONE',  ( -6.505213034913038160E-19, -3.903127820947822896E-18, -1.000000000000000000 ) ) ;
#15857=DIRECTION ( 'NONE',  ( -6.505213034913038160E-19, -3.903127820947822896E-18, -1.000000000000000000 ) ) ;
#15863=CARTESIAN_POINT ( 'NONE',  ( 2.347663744114520057, 31.41239365194192601, -6.999999999999950262 ) ) ;
#15870=AXIS2_PLACEMENT_3D ( 'NONE', #16003, #5152, #3660 ) ;
#15872=CARTESIAN_POINT ( 'NONE',  ( 22.15900668633799597, 29.33526866242094755, 2.800654218530481465 ) ) ;
#15873=CARTESIAN_POINT ( 'NONE',  ( -24.73600648735115115, 27.19760187735867518, 2.800654218530485018 ) ) ;
#15882=EDGE_CURVE ( 'NONE', #11599, #13122, #9382, .T. ) ;
#15885=VECTOR ( 'NONE', #22103, 1000.000000000000000 ) ;
#15886=DIRECTION ( 'NONE',  ( 1.000000000000000000, 1.208970125616063028E-17, 0.000000000000000000 ) ) ;
#15888=CARTESIAN_POINT ( 'NONE',  ( -33.51030287062373247, -15.12081897056669000, -2.800654218530457484 ) ) ;
#15891=VERTEX_POINT ( 'NONE', #20859 ) ;
#15894=EDGE_CURVE ( 'NONE', #5664, #22110, #21076, .T. ) ;
#15895=( NAMED_UNIT ( * ) SI_UNIT ( $, .STERADIAN. ) SOLID_ANGLE_UNIT ( ) );
#15901=DIRECTION ( 'NONE',  ( -1.000000000000000000, -1.208970125616081209E-17, 0.000000000000000000 ) ) ;
#15903=VERTEX_POINT ( 'NONE', #12357 ) ;
#15904=CIRCLE ( 'NONE', #12280, 18.00000000000000000 ) ;
#15905=ORIENTED_EDGE ( 'NONE', *, *, #12811, .F. ) ;
#15908=DIRECTION ( 'NONE',  ( 1.000000000000000000, 0.000000000000000000, 0.000000000000000000 ) ) ;
#15910=DIRECTION ( 'NONE',  ( 6.505213034913038160E-19, 3.903127820947822896E-18, 1.000000000000000000 ) ) ;
#15912=CARTESIAN_POINT ( 'NONE',  ( -21.65063509461084834, 12.49999999999965006, 3.000000000000023537 ) ) ;
#15917=DIRECTION ( 'NONE',  ( -1.000000000000000000, -1.208970125616060101E-17, 6.505213034913038160E-19 ) ) ;
#15921=FACE_OUTER_BOUND ( 'NONE', #2719, .T. ) ;
#15922=VERTEX_POINT ( 'NONE', #15681 ) ;
#15928=ADVANCED_FACE ( 'NONE', ( #5825 ), #9012, .T. ) ;
#15932=AXIS2_PLACEMENT_3D ( 'NONE', #6701, #6593, #10014 ) ;
#15936=VERTEX_POINT ( 'NONE', #20968 ) ;
#15945=ORIENTED_EDGE ( 'NONE', *, *, #10291, .T. ) ;
#15946=DIRECTION ( 'NONE',  ( -1.000000000000000000, -2.650195244404477958E-14, 0.000000000000000000 ) ) ;
#15948=EDGE_LOOP ( 'NONE', ( #1196, #1760, #20851, #17611 ) ) ;
#15950=CIRCLE ( 'NONE', #15592, 31.50000000000001421 ) ;
#15955=FACE_OUTER_BOUND ( 'NONE', #1942, .T. ) ;
#15961=VECTOR ( 'NONE', #21622, 1000.000000000000000 ) ;
#15965=DIRECTION ( 'NONE',  ( 6.505213034913038160E-19, 3.903127820947822896E-18, 1.000000000000000000 ) ) ;
#15967=AXIS2_PLACEMENT_3D ( 'NONE', #4595, #18907, #22122 ) ;
#15970=VERTEX_POINT ( 'NONE', #19813 ) ;
#15972=ORIENTED_EDGE ( 'NONE', *, *, #4022, .F. ) ;
#15975=AXIS2_PLACEMENT_3D ( 'NONE', #9381, #17964, #20992 ) ;
#15976=CARTESIAN_POINT ( 'NONE',  ( 2.775557561562891351E-14, -2.775557561562891351E-14, 2.999999999999995559 ) ) ;
#15978=DIRECTION ( 'NONE',  ( -6.505213034913038160E-19, -3.903127820947822896E-18, -1.000000000000000000 ) ) ;
#15979=DIRECTION ( 'NONE',  ( 6.505213034913038160E-19, 3.903127820947822896E-18, 1.000000000000000000 ) ) ;
#15984=CIRCLE ( 'NONE', #6126, 31.50000000000001421 ) ;
#15989=CARTESIAN_POINT ( 'NONE',  ( 2.347663744114436568, 31.41239365194195443, -2.999999999999971578 ) ) ;
#15990=EDGE_CURVE ( 'NONE', #16547, #14529, #21777, .T. ) ;
#15996=ADVANCED_FACE ( 'NONE', ( #17968 ), #19920, .F. ) ;
#15998=AXIS2_PLACEMENT_3D ( 'NONE', #10911, #14683, #10788 ) ;
#15999=ORIENTED_EDGE ( 'NONE', *, *, #10953, .T. ) ;
#16000=AXIS2_PLACEMENT_3D ( 'NONE', #13467, #20830, #22208 ) ;
#16001=CIRCLE ( 'NONE', #13446, 1.000000000000000888 ) ;
#16003=CARTESIAN_POINT ( 'NONE',  ( 5.551115123125782702E-14, -1.387778780781445676E-13, -5.749999999999949374 ) ) ;
#16005=CARTESIAN_POINT ( 'NONE',  ( 5.551115123125782702E-14, -1.387778780781445676E-13, -5.749999999999949374 ) ) ;
#16007=CYLINDRICAL_SURFACE ( 'NONE', #18532, 36.76383501243555685 ) ;
#16008=CARTESIAN_POINT ( 'NONE',  ( -19.59430950039320152, 28.88846368933331732, -2.999999999999999112 ) ) ;
#16010=CARTESIAN_POINT ( 'NONE',  ( 21.05198877411804048, -30.13956425491232238, 2.800654218530485018 ) ) ;
#16014=CARTESIAN_POINT ( 'NONE',  ( -23.74488952252751162, 25.58633464742629471, -2.999999999999971578 ) ) ;
#16023=CARTESIAN_POINT ( 'NONE',  ( -21.05198877411806890, 30.13956425491229396, 2.800654218530481465 ) ) ;
#16027=CIRCLE ( 'NONE', #12746, 31.50000000000000711 ) ;
#16032=DIRECTION ( 'NONE',  ( -1.000000000000000000, 0.000000000000000000, 0.000000000000000000 ) ) ;
#16034=CARTESIAN_POINT ( 'NONE',  ( -28.07080038625074536, -14.29266125237915830, -6.999999999999992006 ) ) ;
#16039=VERTEX_POINT ( 'NONE', #7662 ) ;
#16043=EDGE_CURVE ( 'NONE', #13884, #9581, #2628, .T. ) ;
#16045=VERTEX_POINT ( 'NONE', #4348 ) ;
#16053=ORIENTED_EDGE ( 'NONE', *, *, #17247, .T. ) ;
#16055=EDGE_CURVE ( 'NONE', #8182, #10164, #9753, .T. ) ;
#16056=ORIENTED_EDGE ( 'NONE', *, *, #7859, .F. ) ;
#16057=CIRCLE ( 'NONE', #2536, 0.9999999999999974465 ) ;
#16059=AXIS2_PLACEMENT_3D ( 'NONE', #11482, #21809, #8270 ) ;
#16060=( NAMED_UNIT ( * ) PLANE_ANGLE_UNIT ( ) SI_UNIT ( $, .RADIAN. ) );
#16061=ORIENTED_EDGE ( 'NONE', *, *, #6995, .T. ) ;
#16066=EDGE_CURVE ( 'NONE', #15217, #17930, #12977, .T. ) ;
#16067=ORIENTED_EDGE ( 'NONE', *, *, #20235, .F. ) ;
#16076=ORIENTED_EDGE ( 'NONE', *, *, #8746, .T. ) ;
#16077=CARTESIAN_POINT ( 'NONE',  ( 35.99819890246980236, -7.463862311151397755, -2.800654218530467698 ) ) ;
#16078=DIRECTION ( 'NONE',  ( -6.505213034913038160E-19, -3.903127820947822896E-18, -1.000000000000000000 ) ) ;
#16086=EDGE_CURVE ( 'NONE', #19434, #8181, #2273, .T. ) ;
#16093=DIRECTION ( 'NONE',  ( -1.000000000000000000, 0.000000000000000000, 0.000000000000000000 ) ) ;
#16094=VECTOR ( 'NONE', #11766, 1000.000000000000000 ) ;
#16104=AXIS2_PLACEMENT_3D ( 'NONE', #16005, #17512, #14389 ) ;
#16107=DIRECTION ( 'NONE',  ( 6.505213034913038160E-19, 3.903127820947822896E-18, 1.000000000000000000 ) ) ;
#16111=EDGE_LOOP ( 'NONE', ( #21302, #936, #16540, #3288 ) ) ;
#16114=DIRECTION ( 'NONE',  ( 6.505213034913038160E-19, 3.903127820947822896E-18, 1.000000000000000000 ) ) ;
#16115=CARTESIAN_POINT ( 'NONE',  ( 1.110223024625156540E-13, -5.551115123125782702E-14, -6.999999999999950262 ) ) ;
#16119=CARTESIAN_POINT ( 'NONE',  ( -10.01331137436150520, 34.09180625983466939, -3.000000000000018208 ) ) ;
#16124=CARTESIAN_POINT ( 'NONE',  ( 26.50842683089785368, -24.41514043009201984, -2.999999999999971578 ) ) ;
#16132=CARTESIAN_POINT ( 'NONE',  ( -18.22261011550271803, -31.92986134326270076, 2.800654218530509443 ) ) ;
#16133=AXIS2_PLACEMENT_3D ( 'NONE', #4833, #15457, #13856 ) ;
#16135=ORIENTED_EDGE ( 'NONE', *, *, #12378, .F. ) ;
#16137=CARTESIAN_POINT ( 'NONE',  ( -36.76383501243532947, -2.502178713904648213E-13, 2.800654218530498785 ) ) ;
#16143=EDGE_CURVE ( 'NONE', #943, #43, #2013, .T. ) ;
#16144=CARTESIAN_POINT ( 'NONE',  ( -12.00937115242646591, -34.74700806321101254, -1.999999999999977573 ) ) ;
#16145=EDGE_CURVE ( 'NONE', #22077, #8307, #8241, .T. ) ;
#16146=DIRECTION ( 'NONE',  ( -1.000000000000000000, -7.117517058857148288E-15, 0.000000000000000000 ) ) ;
#16147=LINE ( 'NONE', #7230, #5300 ) ;
#16155=ADVANCED_FACE ( 'NONE', ( #13238 ), #6507, .T. ) ;
#16156=CARTESIAN_POINT ( 'NONE',  ( 31.11359284679393511, 4.918774254215746211, -2.999999999999988898 ) ) ;
#16157=EDGE_CURVE ( 'NONE', #2785, #5375, #8593, .T. ) ;
#16158=ORIENTED_EDGE ( 'NONE', *, *, #14498, .T. ) ;
#16160=EDGE_CURVE ( 'NONE', #9803, #14096, #6411, .T. ) ;
#16161=ORIENTED_EDGE ( 'NONE', *, *, #4485, .T. ) ;
#16165=APPLICATION_CONTEXT ( 'automotive_design' ) ;
#16166=AXIS2_PLACEMENT_3D ( 'NONE', #14361, #16324, #14600 ) ;
#16168=CARTESIAN_POINT ( 'NONE',  ( 30.33632613426209801, -11.35354668330701422, -7.000000000000006217 ) ) ;
#16173=EDGE_CURVE ( 'NONE', #16276, #15473, #22098, .T. ) ;
#16181=ORIENTED_EDGE ( 'NONE', *, *, #1917, .T. ) ;
#16182=DIRECTION ( 'NONE',  ( 6.505213034913038160E-19, 3.903127820947822896E-18, 1.000000000000000000 ) ) ;
#16183=CARTESIAN_POINT ( 'NONE',  ( -34.13396246814577495, 14.93538271375399695, -2.999999999999999112 ) ) ;
#16185=DIRECTION ( 'NONE',  ( 6.505213034913038160E-19, 3.903127820947822896E-18, 1.000000000000000000 ) ) ;
#16190=DIRECTION ( 'NONE',  ( 6.505213034913038160E-19, 3.903127820947822896E-18, 1.000000000000000000 ) ) ;
#16192=AXIS2_PLACEMENT_3D ( 'NONE', #6409, #11679, #16609 ) ;
#16193=TOROIDAL_SURFACE ( 'NONE', #19138, 34.90673715956759082, 8.750000000000000000 ) ;
#16194=CYLINDRICAL_SURFACE ( 'NONE', #12958, 2.999999999999999112 ) ;
#16195=AXIS2_PLACEMENT_3D ( 'NONE', #9332, #5659, #4073 ) ;
#16205=CARTESIAN_POINT ( 'NONE',  ( -32.75570538720758407, 15.02862401740787135, -6.999999999999950262 ) ) ;
#16207=ORIENTED_EDGE ( 'NONE', *, *, #17163, .F. ) ;
#16214=AXIS2_PLACEMENT_3D ( 'NONE', #17320, #22391, #3478 ) ;
#16216=EDGE_CURVE ( 'NONE', #14343, #2308, #8057, .T. ) ;
#16223=ORIENTED_EDGE ( 'NONE', *, *, #15742, .F. ) ;
#16227=DIRECTION ( 'NONE',  ( 1.000000000000000000, 1.208970125616053475E-17, 0.000000000000000000 ) ) ;
#16228=DIRECTION ( 'NONE',  ( 6.505213034913038160E-19, 3.903127820947822896E-18, 1.000000000000000000 ) ) ;
#16230=EDGE_CURVE ( 'NONE', #19564, #9197, #2755, .T. ) ;
#16232=CIRCLE ( 'NONE', #13290, 19.11328065563151313 ) ;
#16238=EDGE_LOOP ( 'NONE', ( #20123, #3682, #17297, #14337, #7742, #1387 ) ) ;
#16239=DIRECTION ( 'NONE',  ( 1.000000000000000000, 1.208970125616053321E-17, 0.000000000000000000 ) ) ;
#16242=CARTESIAN_POINT ( 'NONE',  ( -24.03323817228457315, 20.36304159388344104, -6.999999999999957367 ) ) ;
#16244=AXIS2_PLACEMENT_3D ( 'NONE', #11577, #11350, #1255 ) ;
#16246=DIRECTION ( 'NONE',  ( -6.505213034913038160E-19, -3.903127820947822896E-18, -1.000000000000000000 ) ) ;
#16251=B_SPLINE_CURVE_WITH_KNOTS ( 'NONE', 3,
 ( #16077, #1886, #8867, #3950 ),
 .UNSPECIFIED., .F., .F.,
 ( 4, 4 ),
 ( 9.545285766871421717E-07, 0.001900595205834707284 ),
 .UNSPECIFIED. ) ;
#16253=ORIENTED_EDGE ( 'NONE', *, *, #20815, .T. ) ;
#16254=EDGE_CURVE ( 'NONE', #5408, #12877, #7515, .T. ) ;
#16261=LINE ( 'NONE', #16034, #8743 ) ;
#16270=ORIENTED_EDGE ( 'NONE', *, *, #21564, .T. ) ;
#16271=FACE_OUTER_BOUND ( 'NONE', #638, .T. ) ;
#16273=DIRECTION ( 'NONE',  ( 6.505213034913038160E-19, 3.903127820947822896E-18, 1.000000000000000000 ) ) ;
#16275=AXIS2_PLACEMENT_3D ( 'NONE', #2519, #2170, #559 ) ;
#16276=VERTEX_POINT ( 'NONE', #8071 ) ;
#16280=AXIS2_PLACEMENT_3D ( 'NONE', #13535, #16985, #1293 ) ;
#16282=ORIENTED_EDGE ( 'NONE', *, *, #13053, .F. ) ;
#16285=EDGE_LOOP ( 'NONE', ( #18201, #17151, #21125, #11809, #12755, #12087 ) ) ;
#16288=AXIS2_PLACEMENT_3D ( 'NONE', #3582, #119, #10541 ) ;
#16289=DIRECTION ( 'NONE',  ( 6.505213034913038160E-19, 3.903127820947822896E-18, 1.000000000000000000 ) ) ;
#16293=CARTESIAN_POINT ( 'NONE',  ( 7.094908322883203056, -35.33352588067112521, -2.999999999999999112 ) ) ;
#16294=DIRECTION ( 'NONE',  ( 1.000000000000000000, 0.000000000000000000, 0.000000000000000000 ) ) ;
#16297=DIRECTION ( 'NONE',  ( -6.505213034913038160E-19, -3.903127820947822896E-18, -1.000000000000000000 ) ) ;
#16303=TOROIDAL_SURFACE ( 'NONE', #5690, 34.90673715956759082, 8.750000000000000000 ) ;
#16309=EDGE_CURVE ( 'NONE', #18373, #8376, #3502, .T. ) ;
#16316=ORIENTED_EDGE ( 'NONE', *, *, #22433, .T. ) ;
#16318=VERTEX_POINT ( 'NONE', #6792 ) ;
#16319=VERTEX_POINT ( 'NONE', #15140 ) ;
#16320=CIRCLE ( 'NONE', #5355, 8.999999999999998224 ) ;
#16324=DIRECTION ( 'NONE',  ( -6.505213034913038160E-19, -3.903127820947822896E-18, -1.000000000000000000 ) ) ;
#16326=AXIS2_PLACEMENT_3D ( 'NONE', #16949, #16732, #22466 ) ;
#16330=FACE_OUTER_BOUND ( 'NONE', #17869, .T. ) ;
#16333=VERTEX_POINT ( 'NONE', #15596 ) ;
#16339=TOROIDAL_SURFACE ( 'NONE', #10832, 34.90673715956759082, 8.750000000000000000 ) ;
#16340=DIRECTION ( 'NONE',  ( -1.000000000000000000, -8.894490888754760711E-15, 0.000000000000000000 ) ) ;
#16341=PLANE ( 'NONE',  #15848 ) ;
#16344=CIRCLE ( 'NONE', #14468, 1.000000000000000888 ) ;
#16345=VERTEX_POINT ( 'NONE', #22500 ) ;
#16346=ADVANCED_FACE ( 'NONE', ( #20776 ), #22159, .F. ) ;
#16347=ORIENTED_EDGE ( 'NONE', *, *, #8075, .F. ) ;
#16351=TOROIDAL_SURFACE ( 'NONE', #14861, 34.90673715956759082, 8.750000000000000000 ) ;
#16359=LINE ( 'NONE', #7661, #2551 ) ;
#16363=AXIS2_PLACEMENT_3D ( 'NONE', #22145, #14793, #9977 ) ;
#16364=ORIENTED_EDGE ( 'NONE', *, *, #15400, .F. ) ;
#16366=CIRCLE ( 'NONE', #2835, 36.76383501243555685 ) ;
#16368=AXIS2_PLACEMENT_3D ( 'NONE', #2270, #9256, #16239 ) ;
#16370=DIRECTION ( 'NONE',  ( 6.505213034913038160E-19, 3.903127820947822896E-18, 1.000000000000000000 ) ) ;
#16373=CARTESIAN_POINT ( 'NONE',  ( 3.608224830031758756E-13, -2.775557561562891351E-14, -4.999999999999997335 ) ) ;
#16374=ORIENTED_EDGE ( 'NONE', *, *, #15293, .F. ) ;
#16376=AXIS2_PLACEMENT_3D ( 'NONE', #17514, #1827, #8810 ) ;
#16377=DIRECTION ( 'NONE',  ( 6.505213034913038160E-19, 3.903127820947822896E-18, 1.000000000000000000 ) ) ;
#16378=DIRECTION ( 'NONE',  ( 6.505213034913038160E-19, 3.903127820947822896E-18, 1.000000000000000000 ) ) ;
#16379=AXIS2_PLACEMENT_3D ( 'NONE', #22676, #17255, #18875 ) ;
#16387=CARTESIAN_POINT ( 'NONE',  ( 19.59430950039339692, -28.88846368933353759, 3.000000000000023537 ) ) ;
#16388=EDGE_LOOP ( 'NONE', ( #2065, #6925, #11206, #9496 ) ) ;
#16393=VERTEX_POINT ( 'NONE', #13639 ) ;
#16394=CIRCLE ( 'NONE', #3246, 19.11328065563151668 ) ;
#16398=VECTOR ( 'NONE', #12327, 1000.000000000000000 ) ;
#16400=AXIS2_PLACEMENT_3D ( 'NONE', #4557, #11990, #15521 ) ;
#16405=CARTESIAN_POINT ( 'NONE',  ( -10.70799354677373572, 35.16985127952371215, 2.800654218530492123 ) ) ;
#16414=ORIENTED_EDGE ( 'NONE', *, *, #17402, .F. ) ;
#16418=CARTESIAN_POINT ( 'NONE',  ( -35.51751788033345747, 1.011722470948090313, -3.000000000000000000 ) ) ;
#16425=CARTESIAN_POINT ( 'NONE',  ( 5.551115123125782702E-14, -1.387778780781445676E-13, -5.749999999999949374 ) ) ;
#16426=AXIS2_PLACEMENT_3D ( 'NONE', #19485, #15910, #14072 ) ;
#16427=CARTESIAN_POINT ( 'NONE',  ( -29.36548507648012318, -13.83143812983131404, -6.999999999999950262 ) ) ;
#16429=DIRECTION ( 'NONE',  ( -1.000000000000000000, -1.208970125616046080E-17, 6.505213034913038160E-19 ) ) ;
#16430=DIRECTION ( 'NONE',  ( -6.505213034913038160E-19, -3.903127820947822896E-18, -1.000000000000000000 ) ) ;
#16431=CARTESIAN_POINT ( 'NONE',  ( 32.75570538720806724, -15.02862401740834386, -6.999999999999957367 ) ) ;
#16433=DIRECTION ( 'NONE',  ( 1.000000000000000000, 1.208970125616063028E-17, 0.000000000000000000 ) ) ;
#16439=ORIENTED_EDGE ( 'NONE', *, *, #13692, .T. ) ;
#16442=PRODUCT_DEFINITION_SHAPE ( 'NONE', 'NONE',  #22019 ) ;
#16447=CARTESIAN_POINT ( 'NONE',  ( 2.220446049250313081E-13, 2.775557561562891351E-14, -2.800654218530485018 ) ) ;
#16453=CARTESIAN_POINT ( 'NONE',  ( 30.48934413892778750, -16.99647590252659057, 3.000000000000027089 ) ) ;
#16457=FACE_OUTER_BOUND ( 'NONE', #22357, .T. ) ;
#16460=ORIENTED_EDGE ( 'NONE', *, *, #6652, .T. ) ;
#16461=ORIENTED_EDGE ( 'NONE', *, *, #11650, .F. ) ;
#16462=CIRCLE ( 'NONE', #7676, 0.9999999999999974465 ) ;
#16463=EDGE_CURVE ( 'NONE', #15027, #16867, #3924, .T. ) ;
#16466=EDGE_CURVE ( 'NONE', #15922, #295, #22175, .T. ) ;
#16477=ORIENTED_EDGE ( 'NONE', *, *, #4917, .T. ) ;
#16479=DIRECTION ( 'NONE',  ( 6.505213034913038160E-19, 3.903127820947822896E-18, 1.000000000000000000 ) ) ;
#16482=EDGE_CURVE ( 'NONE', #4363, #18451, #18144, .T. ) ;
#16487=VECTOR ( 'NONE', #7974, 1000.000000000000000 ) ;
#16489=DIRECTION ( 'NONE',  ( 6.505213034913038160E-19, 3.903127820947822896E-18, 1.000000000000000000 ) ) ;
#16490=LINE ( 'NONE', #19013, #1356 ) ;
#16497=DIRECTION ( 'NONE',  ( 6.505213034913038160E-19, 3.903127820947822896E-18, 1.000000000000000000 ) ) ;
#16500=CIRCLE ( 'NONE', #19444, 34.90673715956759082 ) ;
#16501=CARTESIAN_POINT ( 'NONE',  ( 17.79500259159620512, 31.47514467962667695, 2.932460736555829506 ) ) ;
#16503=LINE ( 'NONE', #4139, #17070 ) ;
#16510=CARTESIAN_POINT ( 'NONE',  ( -32.83234229683724692, 11.85401191286869427, 3.000000000000002665 ) ) ;
#16514=ORIENTED_EDGE ( 'NONE', *, *, #15477, .F. ) ;
#16521=DIRECTION ( 'NONE',  ( 6.505213034913038160E-19, 3.903127820947822896E-18, 1.000000000000000000 ) ) ;
#16523=VERTEX_POINT ( 'NONE', #12171 ) ;
#16525=CARTESIAN_POINT ( 'NONE',  ( -32.10132595304125402, -5.074925817842023790, 3.000000000000006217 ) ) ;
#16527=CARTESIAN_POINT ( 'NONE',  ( 2.775557561562891351E-14, 2.775557561562891351E-14, 5.750000000000001776 ) ) ;
#16537=B_SPLINE_CURVE_WITH_KNOTS ( 'NONE', 3,
 ( #9198, #5990, #19418, #10669 ),
 .UNSPECIFIED., .F., .F.,
 ( 4, 4 ),
 ( 0.001893031756885520502, 0.003808480026563967110 ),
 .UNSPECIFIED. ) ;
#16540=ORIENTED_EDGE ( 'NONE', *, *, #17402, .T. ) ;
#16542=DIRECTION ( 'NONE',  ( -6.505213034913038160E-19, -3.903127820947822896E-18, -1.000000000000000000 ) ) ;
#16543=DIRECTION ( 'NONE',  ( -1.000000000000000000, 0.000000000000000000, 0.000000000000000000 ) ) ;
#16546=AXIS2_PLACEMENT_3D ( 'NONE', #8660, #6837, #18987 ) ;
#16547=VERTEX_POINT ( 'NONE', #127 ) ;
#16549=EDGE_CURVE ( 'NONE', #384, #6508, #21794, .T. ) ;
#16550=VERTEX_POINT ( 'NONE', #467 ) ;
#16551=CYLINDRICAL_SURFACE ( 'NONE', #19493, 19.11328065563152379 ) ;
#16554=CARTESIAN_POINT ( 'NONE',  ( -28.88846368933341324, -19.59430950039325836, -2.999999999999947153 ) ) ;
#16555=CARTESIAN_POINT ( 'NONE',  ( -13.83143812983095344, 29.36548507648009831, 2.999999999999995559 ) ) ;
#16557=EDGE_CURVE ( 'NONE', #19747, #2560, #15904, .T. ) ;
#16558=ORIENTED_EDGE ( 'NONE', *, *, #5324, .T. ) ;
#16559=CARTESIAN_POINT ( 'NONE',  ( 3.330669073875469621E-13, -1.110223024625156540E-13, -2.999999999999971578 ) ) ;
#16562=CARTESIAN_POINT ( 'NONE',  ( 2.775557561562891351E-14, 2.775557561562891351E-14, 5.750000000000001776 ) ) ;
#16563=AXIS2_PLACEMENT_3D ( 'NONE', #14652, #22116, #5956 ) ;
#16570=ADVANCED_FACE ( 'NONE', ( #3477 ), #7123, .T. ) ;
#16573=FACE_OUTER_BOUND ( 'NONE', #16111, .T. ) ;
#16575=B_SPLINE_CURVE_WITH_KNOTS ( 'NONE', 3,
 ( #8635, #22640, #12846, #5528 ),
 .UNSPECIFIED., .F., .F.,
 ( 4, 4 ),
 ( 0.001893031756885543487, 0.003808480026563717744 ),
 .UNSPECIFIED. ) ;
#16576=DIRECTION ( 'NONE',  ( -1.000000000000000000, 0.000000000000000000, 0.000000000000000000 ) ) ;
#16577=AXIS2_PLACEMENT_3D ( 'NONE', #12172, #10552, #13761 ) ;
#16578=DIRECTION ( 'NONE',  ( -6.505213034913038160E-19, -3.903127820947822896E-18, -1.000000000000000000 ) ) ;
#16582=FACE_OUTER_BOUND ( 'NONE', #11205, .T. ) ;
#16586=DIRECTION ( 'NONE',  ( 6.505213034913038160E-19, 3.903127820947822896E-18, 1.000000000000000000 ) ) ;
#16589=PLANE ( 'NONE',  #21164 ) ;
#16593=CYLINDRICAL_SURFACE ( 'NONE', #12252, 0.9999999999999995559 ) ;
#16595=AXIS2_PLACEMENT_3D ( 'NONE', #20969, #10293, #20515 ) ;
#16598=EDGE_CURVE ( 'NONE', #104, #384, #3869, .T. ) ;
#16600=EDGE_CURVE ( 'NONE', #15903, #20662, #4965, .T. ) ;
#16601=CARTESIAN_POINT ( 'NONE',  ( 31.21605069118085751, 8.646032897228927538, -6.999999999999950262 ) ) ;
#16606=DIRECTION ( 'NONE',  ( -1.000000000000000000, -9.076011110974242363E-16, 0.000000000000000000 ) ) ;
#16609=DIRECTION ( 'NONE',  ( 1.000000000000000000, 0.000000000000000000, 0.000000000000000000 ) ) ;
#16612=AXIS2_PLACEMENT_3D ( 'NONE', #7795, #13046, #6304 ) ;
#16616=DIRECTION ( 'NONE',  ( -1.000000000000000000, -1.208970125616044077E-17, 0.000000000000000000 ) ) ;
#16623=CARTESIAN_POINT ( 'NONE',  ( 27.19760187735870005, 24.73600648735113694, -1.999999999999977573 ) ) ;
#16625=VECTOR ( 'NONE', #15062, 1000.000000000000000 ) ;
#16630=ADVANCED_FACE ( 'NONE', ( #3593 ), #5411, .T. ) ;
#16631=ORIENTED_EDGE ( 'NONE', *, *, #10596, .F. ) ;
#16639=DIRECTION ( 'NONE',  ( -1.000000000000000000, 0.000000000000000000, 0.000000000000000000 ) ) ;
#16650=DIRECTION ( 'NONE',  ( -1.000000000000000000, -1.208970125616063644E-17, 0.000000000000000000 ) ) ;
#16652=VERTEX_POINT ( 'NONE', #11234 ) ;
#16656=VECTOR ( 'NONE', #10059, 1000.000000000000000 ) ;
#16658=ORIENTED_EDGE ( 'NONE', *, *, #7537, .F. ) ;
#16659=CIRCLE ( 'NONE', #3120, 36.76383501243555685 ) ;
#16662=VERTEX_POINT ( 'NONE', #21443 ) ;
#16663=ORIENTED_EDGE ( 'NONE', *, *, #2954, .T. ) ;
#16665=EDGE_LOOP ( 'NONE', ( #6313, #10902, #17472, #9565 ) ) ;
#16668=VERTEX_POINT ( 'NONE', #18231 ) ;
#16670=DIRECTION ( 'NONE',  ( 6.505213034913038160E-19, 3.903127820947822896E-18, 1.000000000000000000 ) ) ;
#16672=ORIENTED_EDGE ( 'NONE', *, *, #5558, .F. ) ;
#16673=LINE ( 'NONE', #2708, #13372 ) ;
#16674=CIRCLE ( 'NONE', #21432, 36.76383501243555685 ) ;
#16677=CARTESIAN_POINT ( 'NONE',  ( -35.29097153256766006, -4.153395668489732628, -2.999999999999994671 ) ) ;
#16680=DIRECTION ( 'NONE',  ( -1.000000000000000000, 0.000000000000000000, 0.000000000000000000 ) ) ;
#16682=CIRCLE ( 'NONE', #11564, 0.9999999999999995559 ) ;
#16683=ORIENTED_EDGE ( 'NONE', *, *, #10655, .T. ) ;
#16686=ADVANCED_FACE ( 'NONE', ( #21672 ), #5969, .T. ) ;
#16691=CARTESIAN_POINT ( 'NONE',  ( -23.65408649739099545, -22.22891329980544839, -6.999999999999950262 ) ) ;
#16692=CARTESIAN_POINT ( 'NONE',  ( 1.110223024625156540E-13, -5.551115123125782702E-14, -6.999999999999950262 ) ) ;
#16702=AXIS2_PLACEMENT_3D ( 'NONE', #2764, #9746, #15220 ) ;
#16707=EDGE_CURVE ( 'NONE', #22419, #4210, #8851, .T. ) ;
#16708=DIRECTION ( 'NONE',  ( -1.000000000000000000, -1.208970125616081209E-17, 0.000000000000000000 ) ) ;
#16710=ORIENTED_EDGE ( 'NONE', *, *, #13287, .F. ) ;
#16713=CARTESIAN_POINT ( 'NONE',  ( -12.31876324338271367, -30.07487443287973505, -2.999999999999995559 ) ) ;
#16715=CIRCLE ( 'NONE', #13028, 0.9999999999999974465 ) ;
#16721=ADVANCED_FACE ( 'NONE', ( #6542 ), #16303, .T. ) ;
#16729=CIRCLE ( 'NONE', #9784, 0.9999999999999974465 ) ;
#16730=DIRECTION ( 'NONE',  ( -1.000000000000000000, -1.208970125616044077E-17, 0.000000000000000000 ) ) ;
#16732=DIRECTION ( 'NONE',  ( -6.505213034913038160E-19, -3.903127820947822896E-18, -1.000000000000000000 ) ) ;
#16733=EDGE_CURVE ( 'NONE', #22498, #2692, #19983, .T. ) ;
#16735=AXIS2_PLACEMENT_3D ( 'NONE', #20279, #6064, #18552 ) ;
#16737=CARTESIAN_POINT ( 'NONE',  ( 2.775557561562891351E-14, -2.775557561562891351E-14, 2.999999999999995559 ) ) ;
#16738=VECTOR ( 'NONE', #15595, 1000.000000000000000 ) ;
#16740=ORIENTED_EDGE ( 'NONE', *, *, #16043, .T. ) ;
#16744=ADVANCED_FACE ( 'NONE', ( #8037 ), #20519, .F. ) ;
#16746=CIRCLE ( 'NONE', #1759, 19.11328065563151668 ) ;
#16754=ORIENTED_EDGE ( 'NONE', *, *, #18064, .T. ) ;
#16761=DIRECTION ( 'NONE',  ( -6.505213034913038160E-19, -3.903127820947822896E-18, -1.000000000000000000 ) ) ;
#16763=CARTESIAN_POINT ( 'NONE',  ( 34.88850421923977763, -1.128083539116253586, 3.000000000000023537 ) ) ;
#16767=DIRECTION ( 'NONE',  ( -6.505213034913038160E-19, -3.903127820947822896E-18, -1.000000000000000000 ) ) ;
#16769=EDGE_CURVE ( 'NONE', #7646, #16668, #2430, .T. ) ;
#16775=AXIS2_PLACEMENT_3D ( 'NONE', #3056, #18525, #10030 ) ;
#16779=ORIENTED_EDGE ( 'NONE', *, *, #4506, .T. ) ;
#16780=ORIENTED_EDGE ( 'NONE', *, *, #10469, .F. ) ;
#16781=CIRCLE ( 'NONE', #1044, 31.50000000000000000 ) ;
#16789=DIRECTION ( 'NONE',  ( 1.000000000000000000, 0.000000000000000000, 0.000000000000000000 ) ) ;
#16791=EDGE_LOOP ( 'NONE', ( #18980, #21261, #11290, #8901, #19414, #12039 ) ) ;
#16795=DIRECTION ( 'NONE',  ( -1.000000000000000000, -1.208970125616063644E-17, 0.000000000000000000 ) ) ;
#16800=ADVANCED_FACE ( 'NONE', ( #9864 ), #5054, .F. ) ;
#16805=EDGE_CURVE ( 'NONE', #8029, #1297, #19908, .T. ) ;
#16810=CYLINDRICAL_SURFACE ( 'NONE', #18222, 1.000000000000000888 ) ;
#16812=EDGE_CURVE ( 'NONE', #14951, #20662, #5565, .T. ) ;
#16813=LINE ( 'NONE', #13461, #21818 ) ;
#16814=ORIENTED_EDGE ( 'NONE', *, *, #8927, .F. ) ;
#16816=CARTESIAN_POINT ( 'NONE',  ( 2.220446049250313081E-13, -2.498001805406602216E-13, -6.859353255829918616 ) ) ;
#16819=FACE_OUTER_BOUND ( 'NONE', #21133, .T. ) ;
#16826=B_SPLINE_CURVE_WITH_KNOTS ( 'NONE', 3,
 ( #3819, #17788, #2093, #7476 ),
 .UNSPECIFIED., .F., .F.,
 ( 4, 4 ),
 ( 9.715086409102729949E-07, 0.001929643240672379145 ),
 .UNSPECIFIED. ) ;
#16827=VERTEX_POINT ( 'NONE', #21291 ) ;
#16828=CARTESIAN_POINT ( 'NONE',  ( 24.41514043009221524, 26.50842683089738117, 2.999999999999995559 ) ) ;
#16829=AXIS2_PLACEMENT_3D ( 'NONE', #5243, #19108, #3533 ) ;
#16832=ORIENTED_EDGE ( 'NONE', *, *, #15105, .F. ) ;
#16836=DIRECTION ( 'NONE',  ( -1.000000000000000000, 0.000000000000000000, 0.000000000000000000 ) ) ;
#16839=FACE_OUTER_BOUND ( 'NONE', #6562, .T. ) ;
#16840=AXIS2_PLACEMENT_3D ( 'NONE', #14447, #21579, #5761 ) ;
#16841=FACE_OUTER_BOUND ( 'NONE', #2003, .T. ) ;
#16844=DIRECTION ( 'NONE',  ( 6.505213034913038160E-19, 3.903127820947822896E-18, 1.000000000000000000 ) ) ;
#16852=ORIENTED_EDGE ( 'NONE', *, *, #1553, .F. ) ;
#16853=CIRCLE ( 'NONE', #6977, 36.76383501243555685 ) ;
#16854=DIRECTION ( 'NONE',  ( 1.000000000000000000, 0.000000000000000000, 0.000000000000000000 ) ) ;
#16856=ADVANCED_FACE ( 'NONE', ( #1219 ), #15178, .T. ) ;
#16858=ORIENTED_EDGE ( 'NONE', *, *, #4758, .T. ) ;
#16859=EDGE_CURVE ( 'NONE', #5003, #21713, #16813, .T. ) ;
#16862=DIRECTION ( 'NONE',  ( 6.505213034913038160E-19, 3.903127820947822896E-18, 1.000000000000000000 ) ) ;
#16863=AXIS2_PLACEMENT_3D ( 'NONE', #9537, #2669, #824 ) ;
#16867=VERTEX_POINT ( 'NONE', #20370 ) ;
#16869=FACE_OUTER_BOUND ( 'NONE', #7769, .T. ) ;
#16870=ORIENTED_EDGE ( 'NONE', *, *, #1179, .F. ) ;
#16872=CARTESIAN_POINT ( 'NONE',  ( 3.656418565264413445, 37.07861450834795392, -2.999999999999988898 ) ) ;
#16878=VERTEX_POINT ( 'NONE', #14958 ) ;
#16879=FACE_OUTER_BOUND ( 'NONE', #15948, .T. ) ;
#16881=ORIENTED_EDGE ( 'NONE', *, *, #7298, .T. ) ;
#16888=EDGE_LOOP ( 'NONE', ( #12323, #20826, #16061, #12748 ) ) ;
#16890=ADVANCED_FACE ( 'NONE', ( #22204 ), #13345, .F. ) ;
#16895=CARTESIAN_POINT ( 'NONE',  ( -30.13956425491234725, -21.05198877411829272, -2.800654218530471251 ) ) ;
#16897=ORIENTED_EDGE ( 'NONE', *, *, #7341, .F. ) ;
#16899=ADVANCED_FACE ( 'NONE', ( #9706 ), #20481, .T. ) ;
#16900=VERTEX_POINT ( 'NONE', #7998 ) ;
#16901=FACE_OUTER_BOUND ( 'NONE', #8562, .T. ) ;
#16911=ORIENTED_EDGE ( 'NONE', *, *, #17328, .T. ) ;
#16915=DIRECTION ( 'NONE',  ( 1.000000000000000000, 0.000000000000000000, 0.000000000000000000 ) ) ;
#16917=APPLICATION_CONTEXT ( 'automotive_design' ) ;
#16928=DIRECTION ( 'NONE',  ( -6.505213034913038160E-19, -3.903127820947822896E-18, -1.000000000000000000 ) ) ;
#16930=CARTESIAN_POINT ( 'NONE',  ( 2.775557561562891351E-14, -2.775557561562891351E-14, 2.999999999999999112 ) ) ;
#16934=CIRCLE ( 'NONE', #822, 1.000000000000000888 ) ;
#16935=AXIS2_PLACEMENT_3D ( 'NONE', #16986, #20553, #4410 ) ;
#16936=ORIENTED_EDGE ( 'NONE', *, *, #3680, .F. ) ;
#16941=DIRECTION ( 'NONE',  ( 1.000000000000000000, 1.208970125616053475E-17, 0.000000000000000000 ) ) ;
#16945=LINE ( 'NONE', #4593, #1536 ) ;
#16946=ORIENTED_EDGE ( 'NONE', *, *, #16733, .F. ) ;
#16949=CARTESIAN_POINT ( 'NONE',  ( 37.07861450834818129, -3.656418565264246467, 3.000000000000023537 ) ) ;
#16950=CARTESIAN_POINT ( 'NONE',  ( 23.65408649739122993, 22.22891329980541997, -2.999999999999971578 ) ) ;
#16951=VECTOR ( 'NONE', #6238, 1000.000000000000000 ) ;
#16952=EDGE_LOOP ( 'NONE', ( #115, #8388, #12708, #6734 ) ) ;
#16955=ADVANCED_FACE ( 'NONE', ( #7141 ), #8862, .T. ) ;
#16957=ORIENTED_EDGE ( 'NONE', *, *, #10802, .F. ) ;
#16958=AXIS2_PLACEMENT_3D ( 'NONE', #402, #2354, #16093 ) ;
#16962=EDGE_LOOP ( 'NONE', ( #12069, #12903, #4015, #12689 ) ) ;
#16963=CARTESIAN_POINT ( 'NONE',  ( -4.918774254215746211, 31.11359284679371484, -2.999999999999971578 ) ) ;
#16970=DIRECTION ( 'NONE',  ( -1.000000000000000000, -1.208970125616044077E-17, 0.000000000000000000 ) ) ;
#16971=EDGE_LOOP ( 'NONE', ( #4594, #19392, #11798, #17015, #13953, #12460 ) ) ;
#16972=CARTESIAN_POINT ( 'NONE',  ( -7.980461308159769729, 36.39375341857517299, 3.000000000000023537 ) ) ;
#16977=ORIENTED_EDGE ( 'NONE', *, *, #1714, .T. ) ;
#16979=EDGE_CURVE ( 'NONE', #6211, #14813, #7757, .T. ) ;
#16982=ORIENTED_EDGE ( 'NONE', *, *, #3449, .T. ) ;
#16983=CARTESIAN_POINT ( 'NONE',  ( 31.92986134326233838, -18.22261011550282817, 2.800654218530512551 ) ) ;
#16984=AXIS2_PLACEMENT_3D ( 'NONE', #19012, #6628, #21998 ) ;
#16985=DIRECTION ( 'NONE',  ( 6.505213034913038160E-19, 3.903127820947822896E-18, 1.000000000000000000 ) ) ;
#16986=CARTESIAN_POINT ( 'NONE',  ( 3.330669073875469621E-13, -1.110223024625156540E-13, -2.999999999999971578 ) ) ;
#16991=VECTOR ( 'NONE', #3470, 1000.000000000000000 ) ;
#16993=DIRECTION ( 'NONE',  ( 1.000000000000000000, 0.000000000000000000, 0.000000000000000000 ) ) ;
#16995=DIRECTION ( 'NONE',  ( 1.000000000000000000, 0.000000000000000000, 0.000000000000000000 ) ) ;
#16996=CIRCLE ( 'NONE', #19571, 31.50000000000001421 ) ;
#16997=CARTESIAN_POINT ( 'NONE',  ( 3.330669073875469621E-13, -1.110223024625156540E-13, -2.999999999999971578 ) ) ;
#17005=DIRECTION ( 'NONE',  ( 6.505213034913038160E-19, 3.903127820947822896E-18, 1.000000000000000000 ) ) ;
#17010=EDGE_CURVE ( 'NONE', #1089, #2580, #10914, .T. ) ;
#17011=ADVANCED_FACE ( 'NONE', ( #21020 ), #17913, .T. ) ;
#17015=ORIENTED_EDGE ( 'NONE', *, *, #794, .T. ) ;
#17018=AXIS2_PLACEMENT_3D ( 'NONE', #12906, #16586, #12571 ) ;
#17019=ORIENTED_EDGE ( 'NONE', *, *, #12037, .F. ) ;
#17021=DIRECTION ( 'NONE',  ( 1.000000000000000000, 1.208970125616053475E-17, 0.000000000000000000 ) ) ;
#17032=ORIENTED_EDGE ( 'NONE', *, *, #11411, .T. ) ;
#17034=AXIS2_PLACEMENT_3D ( 'NONE', #6424, #4824, #10070 ) ;
#17035=AXIS2_PLACEMENT_3D ( 'NONE', #14372, #11056, #9228 ) ;
#17037=CARTESIAN_POINT ( 'NONE',  ( 2.220446049250313081E-13, 2.775557561562891351E-14, -2.800654218530485018 ) ) ;
#17039=FACE_OUTER_BOUND ( 'NONE', #13292, .T. ) ;
#17045=EDGE_CURVE ( 'NONE', #9285, #10824, #9670, .T. ) ;
#17048=EDGE_CURVE ( 'NONE', #7486, #1875, #16320, .T. ) ;
#17059=AXIS2_PLACEMENT_3D ( 'NONE', #17949, #14033, #10496 ) ;
#17067=CARTESIAN_POINT ( 'NONE',  ( -5.074925817841608122, 32.10132595304110481, 3.000000000000016431 ) ) ;
#17068=CARTESIAN_POINT ( 'NONE',  ( 24.43568323314253021, -26.65040777864172838, 2.932460736555815739 ) ) ;
#17069=CARTESIAN_POINT ( 'NONE',  ( 27.56232195404068008, -21.41958700883258970, 2.999999999999995559 ) ) ;
#17070=VECTOR ( 'NONE', #14876, 1000.000000000000000 ) ;
#17072=ORIENTED_EDGE ( 'NONE', *, *, #11553, .T. ) ;
#17076=LINE ( 'NONE', #5286, #6270 ) ;
#17078=DIRECTION ( 'NONE',  ( -6.505213034913038160E-19, -3.903127820947822896E-18, -1.000000000000000000 ) ) ;
#17081=DIRECTION ( 'NONE',  ( 1.000000000000000000, 0.000000000000000000, 0.000000000000000000 ) ) ;
#17082=DIRECTION ( 'NONE',  ( 6.505213034913038160E-19, 3.903127820947822896E-18, 1.000000000000000000 ) ) ;
#17088=DIRECTION ( 'NONE',  ( 6.505213034913038160E-19, 3.903127820947822896E-18, 1.000000000000000000 ) ) ;
#17098=DIRECTION ( 'NONE',  ( 1.209647751973867239E-17, 1.000000000000000000, -3.903127820947822896E-18 ) ) ;
#17099=CARTESIAN_POINT ( 'NONE',  ( 24.73600648735124707, -27.19760187735892387, -2.800654218530457484 ) ) ;
#17102=CONICAL_SURFACE ( 'NONE', #9452, 20.00000000000002132, 0.7853981633974543852 ) ;
#17104=ORIENTED_EDGE ( 'NONE', *, *, #15162, .T. ) ;
#17122=CARTESIAN_POINT ( 'NONE',  ( 24.79619811426220366, -21.00948735876903584, -6.999999999999950262 ) ) ;
#17123=DIRECTION ( 'NONE',  ( -6.505213034913038160E-19, -3.903127820947822896E-18, -1.000000000000000000 ) ) ;
#17129=EDGE_LOOP ( 'NONE', ( #19645, #4186, #2059, #3235, #18733, #505 ) ) ;
#17130=ADVANCED_FACE ( 'NONE', ( #5884 ), #11141, .T. ) ;
#17132=CIRCLE ( 'NONE', #20077, 0.9999999999999956701 ) ;
#17133=VERTEX_POINT ( 'NONE', #21694 ) ;
#17134=CARTESIAN_POINT ( 'NONE',  ( -31.41239365194190114, 2.347663744114103501, -7.000000000000006217 ) ) ;
#17135=DIRECTION ( 'NONE',  ( 6.505213034913038160E-19, 3.903127820947822896E-18, 1.000000000000000000 ) ) ;
#17138=DIRECTION ( 'NONE',  ( 6.505213034913038160E-19, 3.903127820947822896E-18, 1.000000000000000000 ) ) ;
#17139=EDGE_CURVE ( 'NONE', #7962, #17550, #9375, .T. ) ;
#17149=LINE ( 'NONE', #1463, #13879 ) ;
#17151=ORIENTED_EDGE ( 'NONE', *, *, #13922, .T. ) ;
#17152=DIRECTION ( 'NONE',  ( -6.505213034913038160E-19, -3.903127820947822896E-18, -1.000000000000000000 ) ) ;
#17153=CYLINDRICAL_SURFACE ( 'NONE', #6031, 36.76383501243555685 ) ;
#17155=ADVANCED_FACE ( 'NONE', ( #3012 ), #20644, .T. ) ;
#17156=ORIENTED_EDGE ( 'NONE', *, *, #16598, .F. ) ;
#17157=EDGE_CURVE ( 'NONE', #18373, #8686, #17309, .T. ) ;
#17162=DIRECTION ( 'NONE',  ( 6.505213034913038160E-19, 3.903127820947822896E-18, 1.000000000000000000 ) ) ;
#17163=EDGE_CURVE ( 'NONE', #8686, #13563, #12300, .T. ) ;
#17164=ORIENTED_EDGE ( 'NONE', *, *, #13581, .T. ) ;
#17176=EDGE_CURVE ( 'NONE', #12190, #21043, #969, .T. ) ;
#17182=DIRECTION ( 'NONE',  ( 6.505213034913038160E-19, 3.903127820947822896E-18, 1.000000000000000000 ) ) ;
#17183=DIRECTION ( 'NONE',  ( -6.505213034913038160E-19, -3.903127820947822896E-18, -1.000000000000000000 ) ) ;
#17184=B_SPLINE_CURVE_WITH_KNOTS ( 'NONE', 3,
 ( #19274, #13964, #1512, #12157 ),
 .UNSPECIFIED., .F., .F.,
 ( 4, 4 ),
 ( 0.001875451646903196793, 0.003761979286331223853 ),
 .UNSPECIFIED. ) ;
#17188=ORIENTED_EDGE ( 'NONE', *, *, #5747, .F. ) ;
#17192=CARTESIAN_POINT ( 'NONE',  ( 15.62726112422616076, 28.45046755804878202, 2.999999999999995559 ) ) ;
#17199=ADVANCED_FACE ( 'NONE', ( #18932 ), #6445, .T. ) ;
#17200=CARTESIAN_POINT ( 'NONE',  ( -18.65063509461084479, 12.49999999999990052, 3.000000000000023537 ) ) ;
#17201=CARTESIAN_POINT ( 'NONE',  ( 35.79662727779919607, -4.171001175319821286, -2.999999999999971578 ) ) ;
#17207=CARTESIAN_POINT ( 'NONE',  ( -20.36304159388344104, -24.03323817228492132, -6.999999999999950262 ) ) ;
#17212=CARTESIAN_POINT ( 'NONE',  ( 32.20238537491837150, 4.080045426412631571, -2.999999999999975131 ) ) ;
#17214=EDGE_CURVE ( 'NONE', #13845, #2563, #4997, .T. ) ;
#17215=VERTEX_POINT ( 'NONE', #17200 ) ;
#17216=VECTOR ( 'NONE', #18347, 1000.000000000000000 ) ;
#17218=ORIENTED_EDGE ( 'NONE', *, *, #22366, .T. ) ;
#17221=CARTESIAN_POINT ( 'NONE',  ( -4.170748987303213084, 34.65667543218822999, 3.000000000000002665 ) ) ;
#17231=ORIENTED_EDGE ( 'NONE', *, *, #9302, .T. ) ;
#17235=AXIS2_PLACEMENT_3D ( 'NONE', #11593, #22026, #13279 ) ;
#17236=CARTESIAN_POINT ( 'NONE',  ( 9.708269511265410046, -33.52953626616050542, -2.999999999999971578 ) ) ;
#17240=AXIS2_PLACEMENT_3D ( 'NONE', #9872, #2666, #6214 ) ;
#17242=ORIENTED_EDGE ( 'NONE', *, *, #20748, .T. ) ;
#17243=ORIENTED_EDGE ( 'NONE', *, *, #1708, .T. ) ;
#17244=B_SPLINE_CURVE_WITH_KNOTS ( 'NONE', 3,
 ( #11176, #14378, #4204, #7745 ),
 .UNSPECIFIED., .F., .F.,
 ( 4, 4 ),
 ( 0.001893031756885613093, 0.003808480026563617130 ),
 .UNSPECIFIED. ) ;
#17247=EDGE_CURVE ( 'NONE', #2560, #19747, #12660, .T. ) ;
#17255=DIRECTION ( 'NONE',  ( -6.505213034913038160E-19, -3.903127820947822896E-18, -1.000000000000000000 ) ) ;
#17256=CARTESIAN_POINT ( 'NONE',  ( -17.99805307122272069, -21.44924440733175786, -2.999999999999971578 ) ) ;
#17259=ADVANCED_FACE ( 'NONE', ( #22491 ), #2054, .T. ) ;
#17263=DIRECTION ( 'NONE',  ( -1.000000000000000000, -1.208970125616046080E-17, 6.505213034913038160E-19 ) ) ;
#17270=CIRCLE ( 'NONE', #1923, 36.76383501243555685 ) ;
#17272=EDGE_LOOP ( 'NONE', ( #6672, #13882, #12444, #14063 ) ) ;
#17280=FACE_OUTER_BOUND ( 'NONE', #15112, .T. ) ;
#17283=CARTESIAN_POINT ( 'NONE',  ( 2.220446049250313081E-13, -8.326672684688674053E-14, 2.800654218530498785 ) ) ;
#17285=ORIENTED_EDGE ( 'NONE', *, *, #9735, .F. ) ;
#17287=CARTESIAN_POINT ( 'NONE',  ( -7.463862311151175710, -35.99819890246952525, -2.800654218530457484 ) ) ;
#17294=ORIENTED_EDGE ( 'NONE', *, *, #19808, .T. ) ;
#17297=ORIENTED_EDGE ( 'NONE', *, *, #18071, .T. ) ;
#17300=CIRCLE ( 'NONE', #109, 34.90673715956759082 ) ;
#17301=DIRECTION ( 'NONE',  ( 1.000000000000000000, 0.000000000000000000, 0.000000000000000000 ) ) ;
#17302=VERTEX_POINT ( 'NONE', #3693 ) ;
#17309=LINE ( 'NONE', #13524, #22558 ) ;
#17316=ORIENTED_EDGE ( 'NONE', *, *, #3376, .F. ) ;
#17318=CIRCLE ( 'NONE', #9273, 36.76383501243555685 ) ;
#17320=CARTESIAN_POINT ( 'NONE',  ( 32.40961249803578426, -2.422192751864227223, -2.999999999999981792 ) ) ;
#17322=CARTESIAN_POINT ( 'NONE',  ( 10.70799354677379256, -35.16985127952393242, 2.800654218530485018 ) ) ;
#17324=CIRCLE ( 'NONE', #1972, 31.50000000000000711 ) ;
#17327=B_SPLINE_CURVE_WITH_KNOTS ( 'NONE', 3,
 ( #21242, #9321, #5647, #19641 ),
 .UNSPECIFIED., .F., .F.,
 ( 4, 4 ),
 ( 0.001875451646902835971, 0.003761979286331349620 ),
 .UNSPECIFIED. ) ;
#17328=EDGE_CURVE ( 'NONE', #928, #12190, #9351, .T. ) ;
#17329=ORIENTED_EDGE ( 'NONE', *, *, #14202, .F. ) ;
#17333=CARTESIAN_POINT ( 'NONE',  ( 2.775557561562891351E-14, 2.775557561562891351E-14, 5.750000000000001776 ) ) ;
#17345=FACE_OUTER_BOUND ( 'NONE', #11265, .T. ) ;
#17347=CARTESIAN_POINT ( 'NONE',  ( -6.070730550690822902, -31.88709182564697286, -7.000000000000006217 ) ) ;
#17352=CARTESIAN_POINT ( 'NONE',  ( 7.980461308159936706, -36.39375341857525825, 3.000000000000023537 ) ) ;
#17365=CARTESIAN_POINT ( 'NONE',  ( -33.52953626616041305, -9.708269511265326557, -2.999999999999971578 ) ) ;
#17369=DIRECTION ( 'NONE',  ( -1.000000000000000000, 0.000000000000000000, 0.000000000000000000 ) ) ;
#17371=CIRCLE ( 'NONE', #4205, 19.11328065563150957 ) ;
#17373=CARTESIAN_POINT ( 'NONE',  ( 31.67162468656012209, 14.67611967928900185, 3.000000000000002665 ) ) ;
#17374=EDGE_CURVE ( 'NONE', #8029, #19756, #934, .T. ) ;
#17375=ORIENTED_EDGE ( 'NONE', *, *, #7753, .F. ) ;
#17376=EDGE_CURVE ( 'NONE', #15616, #12921, #12607, .T. ) ;
#17379=DIRECTION ( 'NONE',  ( -1.000000000000000000, 0.000000000000000000, 0.000000000000000000 ) ) ;
#17382=EDGE_LOOP ( 'NONE', ( #21953, #14073, #17879, #7236 ) ) ;
#17386=CARTESIAN_POINT ( 'NONE',  ( -24.79619811426202247, 21.00948735876864859, 3.000000000000023537 ) ) ;
#17387=ORIENTED_EDGE ( 'NONE', *, *, #5660, .F. ) ;
#17388=DIRECTION ( 'NONE',  ( 6.505213034913038160E-19, 3.903127820947822896E-18, 1.000000000000000000 ) ) ;
#17397=CYLINDRICAL_SURFACE ( 'NONE', #5018, 36.76383501243555685 ) ;
#17399=AXIS2_PLACEMENT_3D ( 'NONE', #14177, #15564, #10522 ) ;
#17402=EDGE_CURVE ( 'NONE', #2694, #66, #557, .T. ) ;
#17413=CARTESIAN_POINT ( 'NONE',  ( 35.51751788033374879, -1.011722470948249963, -2.999999999999986677 ) ) ;
#17417=ORIENTED_EDGE ( 'NONE', *, *, #9809, .F. ) ;
#17419=CARTESIAN_POINT ( 'NONE',  ( 3.330669073875469621E-13, -1.110223024625156540E-13, -2.999999999999971578 ) ) ;
#17420=ORIENTED_EDGE ( 'NONE', *, *, #21612, .F. ) ;
#17421=ADVANCED_FACE ( 'NONE', ( #21557 ), #21779, .T. ) ;
#17429=CARTESIAN_POINT ( 'NONE',  ( -30.60042966911713336, -7.474202570536353285, -6.999999999999992006 ) ) ;
#17437=CIRCLE ( 'NONE', #6476, 31.50000000000000711 ) ;
#17438=EDGE_CURVE ( 'NONE', #19421, #13519, #6533, .T. ) ;
#17441=EDGE_CURVE ( 'NONE', #6416, #22614, #2758, .T. ) ;
#17442=ORIENTED_EDGE ( 'NONE', *, *, #7634, .F. ) ;
#17450=ORIENTED_EDGE ( 'NONE', *, *, #10505, .T. ) ;
#17454=DIRECTION ( 'NONE',  ( 6.505213034913038160E-19, 3.903127820947822896E-18, 1.000000000000000000 ) ) ;
#17455=CARTESIAN_POINT ( 'NONE',  ( 21.94460005644907596, 28.73837443790550239, -2.932164912090539310 ) ) ;
#17457=DIRECTION ( 'NONE',  ( 1.266830946243004623E-16, -1.000000000000000000, -3.903127820947817503E-18 ) ) ;
#17458=EDGE_LOOP ( 'NONE', ( #9398, #1703, #20814, #8657, #7007, #603 ) ) ;
#17461=CARTESIAN_POINT ( 'NONE',  ( 36.75746821813321930, -0.6841746959067585010, -2.800654218530457484 ) ) ;
#17463=AXIS2_PLACEMENT_3D ( 'NONE', #9091, #377, #16294 ) ;
#17467=AXIS2_PLACEMENT_3D ( 'NONE', #13831, #4806, #11775 ) ;
#17472=ORIENTED_EDGE ( 'NONE', *, *, #4345, .T. ) ;
#17473=VECTOR ( 'NONE', #9004, 1000.000000000000000 ) ;
#17479=CIRCLE ( 'NONE', #7610, 0.9999999999999974465 ) ;
#17490=EDGE_CURVE ( 'NONE', #17574, #5266, #11782, .T. ) ;
#17491=ORIENTED_EDGE ( 'NONE', *, *, #20473, .T. ) ;
#17494=AXIS2_PLACEMENT_3D ( 'NONE', #16293, #11135, #15946 ) ;
#17497=EDGE_CURVE ( 'NONE', #11475, #13563, #22119, .T. ) ;
#17500=LINE ( 'NONE', #14500, #10108 ) ;
#17505=VERTEX_POINT ( 'NONE', #1483 ) ;
#17508=CARTESIAN_POINT ( 'NONE',  ( -31.67162468655987340, -14.67611967928944594, -2.999999999999971578 ) ) ;
#17510=VECTOR ( 'NONE', #10258, 1000.000000000000000 ) ;
#17512=DIRECTION ( 'NONE',  ( -6.505213034913038160E-19, -3.903127820947822896E-18, -1.000000000000000000 ) ) ;
#17513=CARTESIAN_POINT ( 'NONE',  ( 25.34312177887357365, -20.17230487860815913, -2.999999999999999112 ) ) ;
#17514=CARTESIAN_POINT ( 'NONE',  ( 17.66631876130919565, -31.41173278719250206, -2.999999999999999112 ) ) ;
#17519=ORIENTED_EDGE ( 'NONE', *, *, #3324, .F. ) ;
#17523=DIRECTION ( 'NONE',  ( -1.000000000000000000, 0.000000000000000000, 0.000000000000000000 ) ) ;
#17524=ORIENTED_EDGE ( 'NONE', *, *, #1644, .T. ) ;
#17527=CARTESIAN_POINT ( 'NONE',  ( 26.79308242454919764, 16.56444186175085065, 2.999999999999995559 ) ) ;
#17529=AXIS2_PLACEMENT_3D ( 'NONE', #11252, #20313, #4501 ) ;
#17538=FACE_OUTER_BOUND ( 'NONE', #13881, .T. ) ;
#17540=CARTESIAN_POINT ( 'NONE',  ( 2.220446049250313081E-13, -8.326672684688674053E-14, 2.800654218530498785 ) ) ;
#17545=CARTESIAN_POINT ( 'NONE',  ( 3.608224830031758756E-13, -2.775557561562891351E-14, -4.999999999999997335 ) ) ;
#17550=VERTEX_POINT ( 'NONE', #16010 ) ;
#17551=DIRECTION ( 'NONE',  ( 6.505213034913038160E-19, 3.903127820947822896E-18, 1.000000000000000000 ) ) ;
#17558=VERTEX_POINT ( 'NONE', #10511 ) ;
#17560=( LENGTH_UNIT ( ) NAMED_UNIT ( * ) SI_UNIT ( .MILLI., .METRE. ) );
#17561=VERTEX_POINT ( 'NONE', #10572 ) ;
#17562=LINE ( 'NONE', #15721, #12174 ) ;
#17566=DIRECTION ( 'NONE',  ( -6.505213034913038160E-19, -3.903127820947822896E-18, -1.000000000000000000 ) ) ;
#17570=ORIENTED_EDGE ( 'NONE', *, *, #650, .T. ) ;
#17574=VERTEX_POINT ( 'NONE', #12454 ) ;
#17577=ORIENTED_EDGE ( 'NONE', *, *, #12349, .T. ) ;
#17578=CARTESIAN_POINT ( 'NONE',  ( 2.775557561562891351E-14, 2.775557561562891351E-14, 5.750000000000001776 ) ) ;
#17583=DIRECTION ( 'NONE',  ( 6.505213034913038160E-19, 3.903127820947822896E-18, 1.000000000000000000 ) ) ;
#17589=EDGE_CURVE ( 'NONE', #5664, #22237, #8597, .T. ) ;
#17590=ORIENTED_EDGE ( 'NONE', *, *, #22688, .F. ) ;
#17591=ORIENTED_EDGE ( 'NONE', *, *, #612, .F. ) ;
#17593=DIRECTION ( 'NONE',  ( -6.505213034913038160E-19, -3.903127820947822896E-18, -1.000000000000000000 ) ) ;
#17596=AXIS2_PLACEMENT_3D ( 'NONE', #16205, #14486, #2133 ) ;
#17599=VECTOR ( 'NONE', #2318, 1000.000000000000000 ) ;
#17600=VERTEX_POINT ( 'NONE', #1591 ) ;
#17601=DIRECTION ( 'NONE',  ( -6.505213034913038160E-19, -3.903127820947822896E-18, -1.000000000000000000 ) ) ;
#17604=DIRECTION ( 'NONE',  ( -6.505213034913038160E-19, -3.903127820947822896E-18, -1.000000000000000000 ) ) ;
#17607=TOROIDAL_SURFACE ( 'NONE', #20551, 34.90673715956759082, 8.750000000000000000 ) ;
#17609=CARTESIAN_POINT ( 'NONE',  ( -2.347663744114242057, -31.41239365194214983, 2.999999999999995559 ) ) ;
#17610=CARTESIAN_POINT ( 'NONE',  ( -24.73600648735115115, 27.19760187735867518, 2.800654218530485018 ) ) ;
#17611=ORIENTED_EDGE ( 'NONE', *, *, #20260, .F. ) ;
#17618=AXIS2_PLACEMENT_3D ( 'NONE', #600, #7362, #10904 ) ;
#17619=CARTESIAN_POINT ( 'NONE',  ( 2.775557561562891351E-14, -2.775557561562891351E-14, 2.999999999999999112 ) ) ;
#17620=ADVANCED_FACE ( 'NONE', ( #5373 ), #1829, .F. ) ;
#17621=DIRECTION ( 'NONE',  ( 1.000000000000000000, 0.000000000000000000, 0.000000000000000000 ) ) ;
#17623=CARTESIAN_POINT ( 'NONE',  ( 30.48934413892814987, -16.99647590252656570, -2.999999999999971578 ) ) ;
#17625=VERTEX_POINT ( 'NONE', #3434 ) ;
#17631=ORIENTED_EDGE ( 'NONE', *, *, #16143, .F. ) ;
#17632=CARTESIAN_POINT ( 'NONE',  ( -24.41514043009185286, -26.50842683089776841, -2.999999999999971578 ) ) ;
#17633=CARTESIAN_POINT ( 'NONE',  ( 31.41173278719253048, 17.66631876130919565, -2.999999999999971578 ) ) ;
#17642=ORIENTED_EDGE ( 'NONE', *, *, #17497, .F. ) ;
#17646=CARTESIAN_POINT ( 'NONE',  ( -31.67162468655980589, -14.67611967928950101, 3.000000000000002665 ) ) ;
#17649=CARTESIAN_POINT ( 'NONE',  ( 4.177897941877526833, -34.13396246814587442, 3.000000000000023537 ) ) ;
#17650=CARTESIAN_POINT ( 'NONE',  ( 31.88709182564702971, -6.070730550690850436, -6.999999999999999112 ) ) ;
#17656=ORIENTED_EDGE ( 'NONE', *, *, #6421, .T. ) ;
#17667=DIRECTION ( 'NONE',  ( 6.505213034913038160E-19, 3.903127820947822896E-18, 1.000000000000000000 ) ) ;
#17668=DIRECTION ( 'NONE',  ( -1.000000000000000000, -1.208970125616027129E-17, 0.000000000000000000 ) ) ;
#17675=EDGE_LOOP ( 'NONE', ( #14157, #9756, #6692, #20578 ) ) ;
#17676=DIRECTION ( 'NONE',  ( -1.000000000000000000, 0.000000000000000000, 0.000000000000000000 ) ) ;
#17678=DIRECTION ( 'NONE',  ( 1.000000000000000000, 0.000000000000000000, 0.000000000000000000 ) ) ;
#17679=ORIENTED_EDGE ( 'NONE', *, *, #14436, .T. ) ;
#17686=CARTESIAN_POINT ( 'NONE',  ( 34.13396246814617996, -14.93538271375438597, -6.999999999999950262 ) ) ;
#17691=TOROIDAL_SURFACE ( 'NONE', #7807, 34.90673715956759082, 8.750000000000000000 ) ;
#17692=CARTESIAN_POINT ( 'NONE',  ( 28.73472116836727253, -21.94328778841628136, 2.932969818539057361 ) ) ;
#17694=AXIS2_PLACEMENT_3D ( 'NONE', #22076, #15965, #8873 ) ;
#17697=ORIENTED_EDGE ( 'NONE', *, *, #17742, .T. ) ;
#17701=DIRECTION ( 'NONE',  ( -1.000000000000000000, 0.000000000000000000, 0.000000000000000000 ) ) ;
#17703=CIRCLE ( 'NONE', #1971, 36.76383501243555685 ) ;
#17705=FACE_OUTER_BOUND ( 'NONE', #14502, .T. ) ;
#17712=ADVANCED_FACE ( 'NONE', ( #3887 ), #14394, .F. ) ;
#17720=EDGE_CURVE ( 'NONE', #16652, #16333, #6556, .T. ) ;
#17722=ORIENTED_EDGE ( 'NONE', *, *, #1206, .T. ) ;
#17729=CYLINDRICAL_SURFACE ( 'NONE', #14156, 36.76383501243555685 ) ;
#17732=DIRECTION ( 'NONE',  ( -6.505213034913038160E-19, -3.903127820947822896E-18, -1.000000000000000000 ) ) ;
#17737=FACE_OUTER_BOUND ( 'NONE', #8626, .T. ) ;
#17739=CARTESIAN_POINT ( 'NONE',  ( 3.330669073875469621E-13, -1.110223024625156540E-13, -2.999999999999971578 ) ) ;
#17740=VECTOR ( 'NONE', #7766, 1000.000000000000000 ) ;
#17742=EDGE_CURVE ( 'NONE', #10689, #2580, #16057, .T. ) ;
#17744=EDGE_CURVE ( 'NONE', #8376, #12666, #10929, .T. ) ;
#17749=CIRCLE ( 'NONE', #16288, 2.999999999999999112 ) ;
#17753=AXIS2_PLACEMENT_3D ( 'NONE', #3806, #10436, #361 ) ;
#17758=CARTESIAN_POINT ( 'NONE',  ( -28.95348479018550236, 14.76298474240492276, -6.999999999999950262 ) ) ;
#17764=DIRECTION ( 'NONE',  ( -6.505213034913038160E-19, -3.903127820947822896E-18, -1.000000000000000000 ) ) ;
#17767=DIRECTION ( 'NONE',  ( 6.505213034913038160E-19, 3.903127820947822896E-18, 1.000000000000000000 ) ) ;
#17768=EDGE_LOOP ( 'NONE', ( #9776, #132, #21412, #13435 ) ) ;
#17769=DIRECTION ( 'NONE',  ( -6.505213034913038160E-19, -3.903127820947822896E-18, -1.000000000000000000 ) ) ;
#17774=DIRECTION ( 'NONE',  ( 6.505213034913038160E-19, 3.903127820947822896E-18, 1.000000000000000000 ) ) ;
#17775=DIRECTION ( 'NONE',  ( -6.505213034913038160E-19, -3.903127820947822896E-18, -1.000000000000000000 ) ) ;
#17777=CIRCLE ( 'NONE', #9362, 19.11328065563152379 ) ;
#17778=CIRCLE ( 'NONE', #20716, 0.9999999999999974465 ) ;
#17779=ORIENTED_EDGE ( 'NONE', *, *, #19931, .T. ) ;
#17780=AXIS2_PLACEMENT_3D ( 'NONE', #9505, #14642, #22104 ) ;
#17781=VERTEX_POINT ( 'NONE', #7744 ) ;
#17782=ORIENTED_EDGE ( 'NONE', *, *, #1499, .F. ) ;
#17784=ORIENTED_EDGE ( 'NONE', *, *, #19552, .F. ) ;
#17785=CARTESIAN_POINT ( 'NONE',  ( 2.775557561562891351E-14, -2.775557561562891351E-14, 2.999999999999995559 ) ) ;
#17788=CARTESIAN_POINT ( 'NONE',  ( -29.74882400976398955, -20.54749497201925479, 2.932969818539056028 ) ) ;
#17791=CARTESIAN_POINT ( 'NONE',  ( 3.330669073875469621E-13, -1.110223024625156540E-13, -2.999999999999971578 ) ) ;
#17795=CIRCLE ( 'NONE', #9010, 34.90673715956759082 ) ;
#17801=LINE ( 'NONE', #2101, #10854 ) ;
#17804=VERTEX_POINT ( 'NONE', #15989 ) ;
#17805=CARTESIAN_POINT ( 'NONE',  ( -19.99999999999999289, -2.799736964075212609E-14, 2.999999999999995559 ) ) ;
#17807=CARTESIAN_POINT ( 'NONE',  ( 2.220446049250313081E-13, -2.498001805406602216E-13, -6.859353255829918616 ) ) ;
#17811=CARTESIAN_POINT ( 'NONE',  ( -16.06969024216325792, -19.15111107797470780, -4.999999999999969802 ) ) ;
#17812=CIRCLE ( 'NONE', #2824, 3.000000000000002665 ) ;
#17813=EDGE_LOOP ( 'NONE', ( #20524, #14358, #4912, #9105 ) ) ;
#17817=ORIENTED_EDGE ( 'NONE', *, *, #15453, .F. ) ;
#17823=CYLINDRICAL_SURFACE ( 'NONE', #17596, 19.11328065563151668 ) ;
#17827=AXIS2_PLACEMENT_3D ( 'NONE', #5737, #3796, #10757 ) ;
#17834=EDGE_CURVE ( 'NONE', #10145, #18993, #21948, .T. ) ;
#17835=TOROIDAL_SURFACE ( 'NONE', #21873, 34.90673715956759082, 8.750000000000000000 ) ;
#17845=CARTESIAN_POINT ( 'NONE',  ( 15.12081897056669000, -33.51030287062373247, -2.800654218530457484 ) ) ;
#17847=AXIS2_PLACEMENT_3D ( 'NONE', #20838, #19110, #1812 ) ;
#17853=CIRCLE ( 'NONE', #13099, 31.50000000000001421 ) ;
#17857=AXIS2_PLACEMENT_3D ( 'NONE', #15051, #4991, #18970 ) ;
#17862=AXIS2_PLACEMENT_3D ( 'NONE', #2781, #8157, #22142 ) ;
#17865=CARTESIAN_POINT ( 'NONE',  ( -9.708269511265271490, 33.52953626616022831, 2.999999999999999112 ) ) ;
#17869=EDGE_LOOP ( 'NONE', ( #20111, #15517, #1878, #188 ) ) ;
#17870=VECTOR ( 'NONE', #7287, 1000.000000000000000 ) ;
#17872=AXIS2_PLACEMENT_3D ( 'NONE', #13769, #3263, #8516 ) ;
#17877=DIRECTION ( 'NONE',  ( 6.505213034913038160E-19, 3.903127820947822896E-18, 1.000000000000000000 ) ) ;
#17878=ADVANCED_FACE ( 'NONE', ( #11855 ), #1439, .T. ) ;
#17879=ORIENTED_EDGE ( 'NONE', *, *, #12200, .T. ) ;
#17880=CARTESIAN_POINT ( 'NONE',  ( 7.094908322883425100, -35.33352588067118205, 2.999999999999995559 ) ) ;
#17890=FACE_OUTER_BOUND ( 'NONE', #8800, .T. ) ;
#17891=CIRCLE ( 'NONE', #683, 1.000000000000000888 ) ;
#17894=DIRECTION ( 'NONE',  ( -1.000000000000000000, 0.000000000000000000, 0.000000000000000000 ) ) ;
#17896=DIRECTION ( 'NONE',  ( 1.000000000000000000, 1.208970125616065955E-17, 0.000000000000000000 ) ) ;
#17900=AXIS2_PLACEMENT_3D ( 'NONE', #5833, #12797, #19812 ) ;
#17907=DIRECTION ( 'NONE',  ( -1.000000000000000000, -1.208970125616063644E-17, 0.000000000000000000 ) ) ;
#17913=CYLINDRICAL_SURFACE ( 'NONE', #14107, 36.76383501243555685 ) ;
#17916=DIRECTION ( 'NONE',  ( -6.505213034913038160E-19, -3.903127820947822896E-18, -1.000000000000000000 ) ) ;
#17918=ORIENTED_EDGE ( 'NONE', *, *, #19649, .T. ) ;
#17922=AXIS2_PLACEMENT_3D ( 'NONE', #20152, #2627, #2735 ) ;
#17924=FACE_OUTER_BOUND ( 'NONE', #9676, .T. ) ;
#17926=ORIENTED_EDGE ( 'NONE', *, *, #11607, .F. ) ;
#17927=ADVANCED_FACE ( 'NONE', ( #6367 ), #1453, .T. ) ;
#17930=VERTEX_POINT ( 'NONE', #14827 ) ;
#17931=ORIENTED_EDGE ( 'NONE', *, *, #3059, .T. ) ;
#17932=DIRECTION ( 'NONE',  ( 6.505213034913038160E-19, 3.903127820947822896E-18, 1.000000000000000000 ) ) ;
#17934=CARTESIAN_POINT ( 'NONE',  ( -15.00354810072192713, 32.89319786336240981, -2.933296326616371186 ) ) ;
#17937=DIRECTION ( 'NONE',  ( 6.505213034913038160E-19, 3.903127820947822896E-18, 1.000000000000000000 ) ) ;
#17938=CARTESIAN_POINT ( 'NONE',  ( -20.36304159388342683, -24.03323817228481118, -2.999999999999999112 ) ) ;
#17940=DIRECTION ( 'NONE',  ( 1.000000000000000000, 0.000000000000000000, 0.000000000000000000 ) ) ;
#17941=CARTESIAN_POINT ( 'NONE',  ( -18.65063509461084479, 12.49999999999990052, -2.999999999999988898 ) ) ;
#17942=CARTESIAN_POINT ( 'NONE',  ( 6.742883674876798850, 34.24928931925757780, -2.999999999999971578 ) ) ;
#17949=CARTESIAN_POINT ( 'NONE',  ( 2.775557561562891351E-14, -2.775557561562891351E-14, 2.999999999999999112 ) ) ;
#17951=EDGE_CURVE ( 'NONE', #16045, #104, #10412, .T. ) ;
#17952=VERTEX_POINT ( 'NONE', #18390 ) ;
#17953=B_SPLINE_CURVE_WITH_KNOTS ( 'NONE', 3,
 ( #8249, #3337, #15221, #1720 ),
 .UNSPECIFIED., .F., .F.,
 ( 4, 4 ),
 ( 0.001875451646902988193, 0.003761979286331204771 ),
 .UNSPECIFIED. ) ;
#17961=DIRECTION ( 'NONE',  ( -1.000000000000000000, 1.052817288873012122E-14, 0.000000000000000000 ) ) ;
#17964=DIRECTION ( 'NONE',  ( -6.505213034913038160E-19, -3.903127820947822896E-18, -1.000000000000000000 ) ) ;
#17968=FACE_OUTER_BOUND ( 'NONE', #12750, .T. ) ;
#17969=ADVANCED_FACE ( 'NONE', ( #4993 ), #12193, .F. ) ;
#17970=CARTESIAN_POINT ( 'NONE',  ( 29.14949368109903816, -11.93972437435564160, -2.999999999999971578 ) ) ;
#17971=ORIENTED_EDGE ( 'NONE', *, *, #20146, .T. ) ;
#17972=FACE_OUTER_BOUND ( 'NONE', #22066, .T. ) ;
#17973=ORIENTED_EDGE ( 'NONE', *, *, #12763, .T. ) ;
#17974=CARTESIAN_POINT ( 'NONE',  ( 24.62019382530525391, -4.341204441673157888, -5.000000000000004441 ) ) ;
#17977=ORIENTED_EDGE ( 'NONE', *, *, #11725, .T. ) ;
#17978=DIRECTION ( 'NONE',  ( 6.505213034913038160E-19, 3.903127820947822896E-18, 1.000000000000000000 ) ) ;
#17983=EDGE_CURVE ( 'NONE', #6403, #10477, #13859, .T. ) ;
#17985=ORIENTED_EDGE ( 'NONE', *, *, #13596, .F. ) ;
#17988=VERTEX_POINT ( 'NONE', #17461 ) ;
#17993=ORIENTED_EDGE ( 'NONE', *, *, #20926, .T. ) ;
#18004=ORIENTED_EDGE ( 'NONE', *, *, #20999, .T. ) ;
#18009=LINE ( 'NONE', #5760, #17599 ) ;
#18013=CYLINDRICAL_SURFACE ( 'NONE', #14522, 3.000000000000002665 ) ;
#18016=CARTESIAN_POINT ( 'NONE',  ( -32.27599279215743877, -14.85437171138610957, 3.000000000000055067 ) ) ;
#18020=DIRECTION ( 'NONE',  ( -6.505213034913038160E-19, -3.903127820947822896E-18, -1.000000000000000000 ) ) ;
#18021=ORIENTED_EDGE ( 'NONE', *, *, #20591, .F. ) ;
#18023=DIRECTION ( 'NONE',  ( -6.505213034913038160E-19, -3.903127820947822896E-18, -1.000000000000000000 ) ) ;
#18026=DIRECTION ( 'NONE',  ( -1.000000000000000000, 0.000000000000000000, 0.000000000000000000 ) ) ;
#18028=CYLINDRICAL_SURFACE ( 'NONE', #102, 19.11328065563151668 ) ;
#18033=VERTEX_POINT ( 'NONE', #14232 ) ;
#18034=ORIENTED_EDGE ( 'NONE', *, *, #17010, .F. ) ;
#18051=VECTOR ( 'NONE', #10895, 1000.000000000000000 ) ;
#18053=DIRECTION ( 'NONE',  ( -6.505213034913038160E-19, -3.903127820947822896E-18, -1.000000000000000000 ) ) ;
#18055=ORIENTED_EDGE ( 'NONE', *, *, #6484, .F. ) ;
#18061=DIRECTION ( 'NONE',  ( -1.000000000000000000, 0.000000000000000000, 0.000000000000000000 ) ) ;
#18064=EDGE_CURVE ( 'NONE', #19379, #16333, #14992, .T. ) ;
#18066=CARTESIAN_POINT ( 'NONE',  ( 3.608224830031758756E-13, -2.775557561562891351E-14, -4.999999999999997335 ) ) ;
#18067=DIRECTION ( 'NONE',  ( 6.505213034913038160E-19, 3.903127820947822896E-18, 1.000000000000000000 ) ) ;
#18069=DIRECTION ( 'NONE',  ( 1.000000000000000000, 0.000000000000000000, 0.000000000000000000 ) ) ;
#18071=EDGE_CURVE ( 'NONE', #14672, #11367, #1819, .T. ) ;
#18074=CARTESIAN_POINT ( 'NONE',  ( 3.656418565264357490, 37.07861450834798234, 2.999999999999995559 ) ) ;
#18076=FACE_OUTER_BOUND ( 'NONE', #20758, .T. ) ;
#18082=VERTEX_POINT ( 'NONE', #19528 ) ;
#18086=VECTOR ( 'NONE', #4849, 1000.000000000000000 ) ;
#18090=MANIFOLD_SOLID_BREP ( 'Cut-Extrude2', #905 ) ;
#18095=DIRECTION ( 'NONE',  ( 6.505213034913038160E-19, 3.903127820947822896E-18, 1.000000000000000000 ) ) ;
#18099=CYLINDRICAL_SURFACE ( 'NONE', #15656, 2.999999999999999112 ) ;
#18105=VERTEX_POINT ( 'NONE', #3440 ) ;
#18107=CIRCLE ( 'NONE', #5663, 34.90673715956759082 ) ;
#18108=CARTESIAN_POINT ( 'NONE',  ( 2.220446049250313081E-13, -2.498001805406602216E-13, -6.859353255829918616 ) ) ;
#18127=CARTESIAN_POINT ( 'NONE',  ( 3.330669073875469621E-13, -1.110223024625156540E-13, -2.999999999999971578 ) ) ;
#18132=CARTESIAN_POINT ( 'NONE',  ( 21.66577056626875475, -3.820259908672546167, 3.000000000000009770 ) ) ;
#18134=EDGE_LOOP ( 'NONE', ( #11611, #18543, #22078, #21370 ) ) ;
#18136=DIRECTION ( 'NONE',  ( -1.000000000000000000, -1.208970125616083366E-17, 0.000000000000000000 ) ) ;
#18137=CARTESIAN_POINT ( 'NONE',  ( 4.918774254215884767, -31.11359284679388182, -2.999999999999999112 ) ) ;
#18138=EDGE_LOOP ( 'NONE', ( #4208, #2051, #21235, #18934 ) ) ;
#18139=DIRECTION ( 'NONE',  ( -6.505213034913038160E-19, -3.903127820947822896E-18, -1.000000000000000000 ) ) ;
#18140=DIRECTION ( 'NONE',  ( -1.000000000000000000, -1.208970125616077665E-17, 0.000000000000000000 ) ) ;
#18141=ORIENTED_EDGE ( 'NONE', *, *, #3874, .F. ) ;
#18144=CIRCLE ( 'NONE', #14821, 19.11328065563151668 ) ;
#18145=LINE ( 'NONE', #16427, #11460 ) ;
#18146=VECTOR ( 'NONE', #7853, 1000.000000000000000 ) ;
#18147=CIRCLE ( 'NONE', #19596, 34.90673715956759082 ) ;
#18154=ADVANCED_FACE ( 'NONE', ( #18076 ), #14635, .T. ) ;
#18155=ORIENTED_EDGE ( 'NONE', *, *, #9326, .T. ) ;
#18158=VECTOR ( 'NONE', #13008, 1000.000000000000000 ) ;
#18161=VERTEX_POINT ( 'NONE', #12683 ) ;
#18168=EDGE_CURVE ( 'NONE', #2517, #928, #21354, .T. ) ;
#18170=ORIENTED_EDGE ( 'NONE', *, *, #17744, .T. ) ;
#18172=CARTESIAN_POINT ( 'NONE',  ( 32.83234229683737482, -11.85401191286897316, -2.999999999999971578 ) ) ;
#18175=CARTESIAN_POINT ( 'NONE',  ( 22.97438720605776652, -22.98755168577443087, 2.999999999999995559 ) ) ;
#18177=DIRECTION ( 'NONE',  ( -6.505213034913038160E-19, -3.903127820947822896E-18, -1.000000000000000000 ) ) ;
#18179=CIRCLE ( 'NONE', #9017, 31.50000000000001421 ) ;
#18180=VERTEX_POINT ( 'NONE', #14518 ) ;
#18183=AXIS2_PLACEMENT_3D ( 'NONE', #5293, #15804, #6563 ) ;
#18197=CARTESIAN_POINT ( 'NONE',  ( -35.43002037646303393, 7.196011215416572959, -2.933296326616368521 ) ) ;
#18198=DIRECTION ( 'NONE',  ( 1.000000000000000000, 0.000000000000000000, 0.000000000000000000 ) ) ;
#18201=ORIENTED_EDGE ( 'NONE', *, *, #17214, .T. ) ;
#18206=DIRECTION ( 'NONE',  ( -6.505213034913038160E-19, -3.903127820947822896E-18, -1.000000000000000000 ) ) ;
#18208=ADVANCED_FACE ( 'NONE', ( #7427 ), #19706, .T. ) ;
#18209=VERTEX_POINT ( 'NONE', #14738 ) ;
#18210=CARTESIAN_POINT ( 'NONE',  ( 27.84804035626042662, -24.75236754129164751, 3.000000000000023537 ) ) ;
#18212=AXIS2_PLACEMENT_3D ( 'NONE', #18127, #7702, #17668 ) ;
#18216=DIRECTION ( 'NONE',  ( 6.505213034913038160E-19, 3.903127820947822896E-18, 1.000000000000000000 ) ) ;
#18219=CARTESIAN_POINT ( 'NONE',  ( 2.775557561562891351E-14, -2.775557561562891351E-14, 2.999999999999995559 ) ) ;
#18220=DIRECTION ( 'NONE',  ( 1.000000000000000000, 0.000000000000000000, 0.000000000000000000 ) ) ;
#18221=FACE_OUTER_BOUND ( 'NONE', #20427, .T. ) ;
#18222=AXIS2_PLACEMENT_3D ( 'NONE', #10259, #1114, #15063 ) ;
#18226=CARTESIAN_POINT ( 'NONE',  ( 2.220446049250313081E-13, -2.498001805406602216E-13, -6.859353255829918616 ) ) ;
#18227=FACE_BOUND ( 'NONE', #8152, .T. ) ;
#18231=CARTESIAN_POINT ( 'NONE',  ( -4.074925817841607234, 32.10132595304121850, 3.000000000000016431 ) ) ;
#18234=AXIS2_PLACEMENT_3D ( 'NONE', #18845, #6697, #12185 ) ;
#18239=ADVANCED_FACE ( 'NONE', ( #9386 ), #7887, .F. ) ;
#18252=ORIENTED_EDGE ( 'NONE', *, *, #21735, .T. ) ;
#18257=CARTESIAN_POINT ( 'NONE',  ( -4.936596639065260916, -31.11077005834428277, -6.999999999999950262 ) ) ;
#18259=DIRECTION ( 'NONE',  ( 1.000000000000000000, 1.208970125616063182E-17, 0.000000000000000000 ) ) ;
#18266=EDGE_CURVE ( 'NONE', #11125, #19820, #16359, .T. ) ;
#18269=AXIS2_PLACEMENT_3D ( 'NONE', #5642, #12616, #19631 ) ;
#18272=ORIENTED_EDGE ( 'NONE', *, *, #5933, .T. ) ;
#18273=AXIS2_PLACEMENT_3D ( 'NONE', #1648, #15491, #16993 ) ;
#18275=CARTESIAN_POINT ( 'NONE',  ( -17.86915608785649567, 27.01645732367846620, -2.999999999999999112 ) ) ;
#18276=CYLINDRICAL_SURFACE ( 'NONE', #3421, 19.11328065563151668 ) ;
#18277=ORIENTED_EDGE ( 'NONE', *, *, #6377, .F. ) ;
#18279=VERTEX_POINT ( 'NONE', #11879 ) ;
#18283=CARTESIAN_POINT ( 'NONE',  ( -16.99647590252643781, -30.48934413892778750, -2.999999999999992450 ) ) ;
#18290=CARTESIAN_POINT ( 'NONE',  ( 5.551115123125782702E-14, -1.387778780781445676E-13, -5.749999999999949374 ) ) ;
#18293=ORIENTED_EDGE ( 'NONE', *, *, #2705, .T. ) ;
#18301=VECTOR ( 'NONE', #20462, 1000.000000000000000 ) ;
#18305=CARTESIAN_POINT ( 'NONE',  ( -16.06969024216335740, -19.15111107797456924, -2.999999999999995559 ) ) ;
#18310=DIRECTION ( 'NONE',  ( 6.505213034913038160E-19, 3.903127820947822896E-18, 1.000000000000000000 ) ) ;
#18312=ORIENTED_EDGE ( 'NONE', *, *, #19505, .F. ) ;
#18313=FACE_BOUND ( 'NONE', #13182, .T. ) ;
#18317=EDGE_CURVE ( 'NONE', #21371, #13393, #16462, .T. ) ;
#18318=AXIS2_PLACEMENT_3D ( 'NONE', #11626, #6357, #18734 ) ;
#18320=ORIENTED_EDGE ( 'NONE', *, *, #15041, .T. ) ;
#18321=DIRECTION ( 'NONE',  ( -6.505213034913038160E-19, -3.903127820947822896E-18, -1.000000000000000000 ) ) ;
#18322=EDGE_CURVE ( 'NONE', #13710, #16662, #4684, .T. ) ;
#18324=ORIENTED_EDGE ( 'NONE', *, *, #12470, .T. ) ;
#18327=CARTESIAN_POINT ( 'NONE',  ( 31.11077005834428277, -4.936596639065260916, -2.999999999999971578 ) ) ;
#18334=CARTESIAN_POINT ( 'NONE',  ( 7.196011215416979745, 35.43002037646296998, -2.933296326616370298 ) ) ;
#18337=ORIENTED_EDGE ( 'NONE', *, *, #15990, .F. ) ;
#18338=EDGE_CURVE ( 'NONE', #13199, #3604, #11546, .T. ) ;
#18339=DIRECTION ( 'NONE',  ( 6.505213034913038160E-19, 3.903127820947822896E-18, 1.000000000000000000 ) ) ;
#18340=CARTESIAN_POINT ( 'NONE',  ( -21.69517388068220853, -28.13960001536977629, -2.999999999999998224 ) ) ;
#18342=ORIENTED_EDGE ( 'NONE', *, *, #5667, .F. ) ;
#18343=ORIENTED_EDGE ( 'NONE', *, *, #18998, .T. ) ;
#18344=ORIENTED_EDGE ( 'NONE', *, *, #22440, .F. ) ;
#18347=DIRECTION ( 'NONE',  ( 6.505213034913038160E-19, 3.903127820947822896E-18, 1.000000000000000000 ) ) ;
#18355=EDGE_CURVE ( 'NONE', #16393, #21378, #10155, .T. ) ;
#18357=AXIS2_PLACEMENT_3D ( 'NONE', #21230, #4052, #14443 ) ;
#18373=VERTEX_POINT ( 'NONE', #2964 ) ;
#18376=EDGE_CURVE ( 'NONE', #11307, #4097, #17149, .T. ) ;
#18377=ORIENTED_EDGE ( 'NONE', *, *, #2889, .F. ) ;
#18378=ORIENTED_EDGE ( 'NONE', *, *, #3000, .T. ) ;
#18379=CARTESIAN_POINT ( 'NONE',  ( 26.10603996529656357, 24.10117729468382564, 3.000000000000030198 ) ) ;
#18380=DIRECTION ( 'NONE',  ( -1.000000000000000000, 0.000000000000000000, 0.000000000000000000 ) ) ;
#18381=EDGE_LOOP ( 'NONE', ( #3445, #4930, #7258, #9409 ) ) ;
#18382=CARTESIAN_POINT ( 'NONE',  ( -29.32895111104219410, -20.05817253550624812, -2.999999999999996447 ) ) ;
#18386=LINE ( 'NONE', #13439, #18301 ) ;
#18387=CARTESIAN_POINT ( 'NONE',  ( 32.20238537491839992, 4.080045426412798548, -6.999999999999950262 ) ) ;
#18390=CARTESIAN_POINT ( 'NONE',  ( 20.17230487860829768, 25.34312177887326811, -2.999999999999971578 ) ) ;
#18393=AXIS2_PLACEMENT_3D ( 'NONE', #10468, #20921, #18975 ) ;
#18394=LINE ( 'NONE', #2715, #9298 ) ;
#18397=ORIENTED_EDGE ( 'NONE', *, *, #3662, .F. ) ;
#18401=DIRECTION ( 'NONE',  ( 6.505213034913038160E-19, 3.903127820947822896E-18, 1.000000000000000000 ) ) ;
#18402=AXIS2_PLACEMENT_3D ( 'NONE', #15976, #11986, #12320 ) ;
#18403=VECTOR ( 'NONE', #16185, 1000.000000000000000 ) ;
#18408=CARTESIAN_POINT ( 'NONE',  ( -30.13956425491219449, -21.05198877411826430, 2.800654218530505890 ) ) ;
#18413=VERTEX_POINT ( 'NONE', #17373 ) ;
#18414=CARTESIAN_POINT ( 'NONE',  ( -8.485281374238484275, 2.999999999999780620, -4.999999999999997335 ) ) ;
#18415=EDGE_CURVE ( 'NONE', #17133, #5664, #20867, .T. ) ;
#18419=ADVANCED_FACE ( 'NONE', ( #302 ), #6967, .F. ) ;
#18424=CARTESIAN_POINT ( 'NONE',  ( 11.93972437435558653, 29.14949368109881433, -2.999999999999999112 ) ) ;
#18425=AXIS2_PLACEMENT_3D ( 'NONE', #21411, #332, #14403 ) ;
#18428=EDGE_CURVE ( 'NONE', #7580, #11124, #9148, .T. ) ;
#18433=CYLINDRICAL_SURFACE ( 'NONE', #16735, 0.9999999999999956701 ) ;
#18436=CYLINDRICAL_SURFACE ( 'NONE', #746, 19.11328065563150957 ) ;
#18438=CARTESIAN_POINT ( 'NONE',  ( 14.74639653023226948, -28.96193690644938101, 2.999999999999995559 ) ) ;
#18441=AXIS2_PLACEMENT_3D ( 'NONE', #13263, #6418, #8247 ) ;
#18443=CARTESIAN_POINT ( 'NONE',  ( 29.36548507648054240, 13.83143812983103693, -6.999999999999950262 ) ) ;
#18445=DIRECTION ( 'NONE',  ( -6.505213034913038160E-19, -3.903127820947822896E-18, -1.000000000000000000 ) ) ;
#18446=EDGE_LOOP ( 'NONE', ( #3029, #14927, #10235, #11984 ) ) ;
#18447=DIRECTION ( 'NONE',  ( -1.000000000000000000, 0.000000000000000000, 0.000000000000000000 ) ) ;
#18451=VERTEX_POINT ( 'NONE', #2022 ) ;
#18453=VECTOR ( 'NONE', #12480, 1000.000000000000000 ) ;
#18456=VECTOR ( 'NONE', #13754, 1000.000000000000000 ) ;
#18465=CIRCLE ( 'NONE', #173, 31.50000000000001421 ) ;
#18469=FACE_OUTER_BOUND ( 'NONE', #13268, .T. ) ;
#18474=B_SPLINE_CURVE_WITH_KNOTS ( 'NONE', 3,
 ( #3222, #6543, #17068, #10071 ),
 .UNSPECIFIED., .F., .F.,
 ( 4, 4 ),
 ( 0.001875451646902768750, 0.003761979286331133213 ),
 .UNSPECIFIED. ) ;
#18478=ORIENTED_EDGE ( 'NONE', *, *, #14749, .F. ) ;
#18480=CARTESIAN_POINT ( 'NONE',  ( -14.76298474240489433, -28.95348479018577947, -6.999999999999999112 ) ) ;
#18484=EDGE_CURVE ( 'NONE', #18822, #586, #363, .T. ) ;
#18485=CARTESIAN_POINT ( 'NONE',  ( 3.330669073875469621E-13, -1.110223024625156540E-13, -2.999999999999971578 ) ) ;
#18487=AXIS2_PLACEMENT_3D ( 'NONE', #4226, #2166, #14402 ) ;
#18490=EDGE_CURVE ( 'NONE', #12877, #18279, #17244, .T. ) ;
#18491=VERTEX_POINT ( 'NONE', #19894 ) ;
#18492=AXIS2_PLACEMENT_3D ( 'NONE', #17545, #19161, #20765 ) ;
#18493=ORIENTED_EDGE ( 'NONE', *, *, #14410, .T. ) ;
#18496=CARTESIAN_POINT ( 'NONE',  ( 2.220446049250313081E-13, -8.326672684688674053E-14, 2.800654218530498785 ) ) ;
#18499=VERTEX_POINT ( 'NONE', #14717 ) ;
#18500=CARTESIAN_POINT ( 'NONE',  ( 2.775557561562891351E-14, -2.775557561562891351E-14, 2.999999999999999112 ) ) ;
#18503=AXIS2_PLACEMENT_3D ( 'NONE', #2992, #1378, #13607 ) ;
#18504=CARTESIAN_POINT ( 'NONE',  ( -29.14949368109887118, 11.93972437435536449, -6.999999999999999112 ) ) ;
#18507=DIRECTION ( 'NONE',  ( -6.505213034913038160E-19, -3.903127820947822896E-18, -1.000000000000000000 ) ) ;
#18510=DIRECTION ( 'NONE',  ( 6.505213034913038160E-19, 3.903127820947822896E-18, 1.000000000000000000 ) ) ;
#18511=DIRECTION ( 'NONE',  ( -6.505213034913038160E-19, -3.903127820947822896E-18, -1.000000000000000000 ) ) ;
#18512=CIRCLE ( 'NONE', #11557, 28.00000000000001066 ) ;
#18520=ORIENTED_EDGE ( 'NONE', *, *, #20260, .T. ) ;
#18524=CARTESIAN_POINT ( 'NONE',  ( 1.110223024625156540E-13, -5.551115123125782702E-14, -6.999999999999950262 ) ) ;
#18525=DIRECTION ( 'NONE',  ( 6.505213034913038160E-19, 3.903127820947822896E-18, 1.000000000000000000 ) ) ;
#18528=ORIENTED_EDGE ( 'NONE', *, *, #11274, .F. ) ;
#18530=DIRECTION ( 'NONE',  ( 1.000000000000000000, 1.208970125616063182E-17, 0.000000000000000000 ) ) ;
#18531=CYLINDRICAL_SURFACE ( 'NONE', #1048, 31.50000000000000711 ) ;
#18532=AXIS2_PLACEMENT_3D ( 'NONE', #16816, #15070, #9827 ) ;
#18537=EDGE_LOOP ( 'NONE', ( #18377, #35, #5006, #8330 ) ) ;
#18538=FACE_OUTER_BOUND ( 'NONE', #14684, .T. ) ;
#18541=LINE ( 'NONE', #11327, #2343 ) ;
#18543=ORIENTED_EDGE ( 'NONE', *, *, #21013, .T. ) ;
#18546=DIRECTION ( 'NONE',  ( -1.000000000000000000, 0.000000000000000000, 0.000000000000000000 ) ) ;
#18551=FACE_OUTER_BOUND ( 'NONE', #3277, .T. ) ;
#18552=DIRECTION ( 'NONE',  ( 1.000000000000000000, 0.000000000000000000, 0.000000000000000000 ) ) ;
#18553=ORIENTED_EDGE ( 'NONE', *, *, #4266, .T. ) ;
#18564=DIRECTION ( 'NONE',  ( -1.000000000000000000, 0.000000000000000000, 0.000000000000000000 ) ) ;
#18569=AXIS2_PLACEMENT_3D ( 'NONE', #11891, #22113, #3203 ) ;
#18572=CARTESIAN_POINT ( 'NONE',  ( -4.170748987303213084, 34.65667543218822999, -2.999999999999971578 ) ) ;
#18573=EDGE_CURVE ( 'NONE', #3830, #4700, #763, .T. ) ;
#18575=EDGE_CURVE ( 'NONE', #7962, #15903, #14612, .T. ) ;
#18576=AXIS2_PLACEMENT_3D ( 'NONE', #5982, #16289, #2441 ) ;
#18579=AXIS2_PLACEMENT_3D ( 'NONE', #8054, #17082, #18593 ) ;
#18580=AXIS2_PLACEMENT_3D ( 'NONE', #20398, #19941, #14764 ) ;
#18581=EDGE_CURVE ( 'NONE', #15288, #13346, #1830, .T. ) ;
#18587=DIRECTION ( 'NONE',  ( -1.000000000000000000, -1.208970125616077665E-17, 0.000000000000000000 ) ) ;
#18588=LINE ( 'NONE', #19149, #406 ) ;
#18592=DIRECTION ( 'NONE',  ( -6.505213034913038160E-19, -3.903127820947822896E-18, -1.000000000000000000 ) ) ;
#18593=DIRECTION ( 'NONE',  ( 1.000000000000000000, 0.000000000000000000, 0.000000000000000000 ) ) ;
#18596=CARTESIAN_POINT ( 'NONE',  ( 28.96193690644979668, 14.74639653023213093, 2.999999999999995559 ) ) ;
#18601=DIRECTION ( 'NONE',  ( 6.505213034913038160E-19, 3.903127820947822896E-18, 1.000000000000000000 ) ) ;
#18602=TOROIDAL_SURFACE ( 'NONE', #1405, 34.90673715956759082, 8.750000000000000000 ) ;
#18612=AXIS2_PLACEMENT_3D ( 'NONE', #12321, #19096, #8664 ) ;
#18616=ADVANCED_FACE ( 'NONE', ( #9087 ), #5316, .F. ) ;
#18617=VERTEX_POINT ( 'NONE', #3608 ) ;
#18619=ORIENTED_EDGE ( 'NONE', *, *, #19548, .F. ) ;
#18624=AXIS2_PLACEMENT_3D ( 'NONE', #14163, #18067, #8911 ) ;
#18625=EDGE_CURVE ( 'NONE', #19349, #14184, #15715, .T. ) ;
#18630=VECTOR ( 'NONE', #5070, 1000.000000000000000 ) ;
#18634=CYLINDRICAL_SURFACE ( 'NONE', #5062, 19.11328065563152379 ) ;
#18635=CARTESIAN_POINT ( 'NONE',  ( -35.52192638951989068, 1.010906942018126697, 3.000000000000041744 ) ) ;
#18646=DIRECTION ( 'NONE',  ( 6.505213034913038160E-19, 3.903127820947822896E-18, 1.000000000000000000 ) ) ;
#18647=AXIS2_PLACEMENT_3D ( 'NONE', #16562, #18511, #11634 ) ;
#18660=DIRECTION ( 'NONE',  ( 6.505213034913038160E-19, 3.903127820947822896E-18, 1.000000000000000000 ) ) ;
#18662=ORIENTED_EDGE ( 'NONE', *, *, #21966, .T. ) ;
#18664=CARTESIAN_POINT ( 'NONE',  ( -0.6841746959065087008, -36.75746821813308429, -2.800654218530457484 ) ) ;
#18668=CYLINDRICAL_SURFACE ( 'NONE', #21375, 19.11328065563151668 ) ;
#18669=CIRCLE ( 'NONE', #8793, 19.11328065563152379 ) ;
#18672=ORIENTED_EDGE ( 'NONE', *, *, #13343, .T. ) ;
#18674=AXIS2_PLACEMENT_3D ( 'NONE', #481, #14568, #17907 ) ;
#18675=CARTESIAN_POINT ( 'NONE',  ( -2.347663744114047990, -31.41239365194231681, -2.999999999999995559 ) ) ;
#18677=EDGE_CURVE ( 'NONE', #8182, #5375, #19857, .T. ) ;
#18683=DIRECTION ( 'NONE',  ( -6.505213034913038160E-19, -3.903127820947822896E-18, -1.000000000000000000 ) ) ;
#18691=EDGE_CURVE ( 'NONE', #7599, #1088, #6969, .T. ) ;
#18694=ORIENTED_EDGE ( 'NONE', *, *, #12938, .F. ) ;
#18698=DIRECTION ( 'NONE',  ( 1.000000000000000000, 1.208970125616063490E-17, 0.000000000000000000 ) ) ;
#18700=CARTESIAN_POINT ( 'NONE',  ( 8.646032897229204650, -31.21605069118105291, -2.999999999999981792 ) ) ;
#18701=VERTEX_POINT ( 'NONE', #7705 ) ;
#18703=CARTESIAN_POINT ( 'NONE',  ( 34.64554704988886158, 10.35112103033863029, -2.932164912090505560 ) ) ;
#18709=CARTESIAN_POINT ( 'NONE',  ( 4.080045426412798548, -32.20238537491815123, -2.999999999999971578 ) ) ;
#18711=EDGE_LOOP ( 'NONE', ( #7797, #21734, #10794, #16158 ) ) ;
#18716=VERTEX_POINT ( 'NONE', #13065 ) ;
#18717=FACE_OUTER_BOUND ( 'NONE', #22133, .T. ) ;
#18719=EDGE_CURVE ( 'NONE', #18716, #6587, #10975, .T. ) ;
#18729=VECTOR ( 'NONE', #3345, 1000.000000000000000 ) ;
#18730=EDGE_LOOP ( 'NONE', ( #12081, #14721, #14364, #11105 ) ) ;
#18731=DIRECTION ( 'NONE',  ( 6.505213034913038160E-19, 3.903127820947822896E-18, 1.000000000000000000 ) ) ;
#18733=ORIENTED_EDGE ( 'NONE', *, *, #16157, .T. ) ;
#18734=DIRECTION ( 'NONE',  ( 1.000000000000000000, 0.000000000000000000, 0.000000000000000000 ) ) ;
#18737=DIRECTION ( 'NONE',  ( 6.505213034913038160E-19, 3.903127820947822896E-18, 1.000000000000000000 ) ) ;
#18738=DIRECTION ( 'NONE',  ( -1.000000000000000000, 0.000000000000000000, 0.000000000000000000 ) ) ;
#18741=EDGE_CURVE ( 'NONE', #9197, #12493, #1110, .T. ) ;
#18749=DIRECTION ( 'NONE',  ( -1.000000000000000000, -1.208970125616081209E-17, 0.000000000000000000 ) ) ;
#18750=B_SPLINE_CURVE_WITH_KNOTS ( 'NONE', 3,
 ( #19203, #7276, #5546, #278 ),
 .UNSPECIFIED., .F., .F.,
 ( 4, 4 ),
 ( 9.545285769565287186E-07, 0.001900595205834659795 ),
 .UNSPECIFIED. ) ;
#18753=CIRCLE ( 'NONE', #4859, 19.11328065563151668 ) ;
#18755=DIRECTION ( 'NONE',  ( 6.505213034913038160E-19, 3.903127820947822896E-18, 1.000000000000000000 ) ) ;
#18766=DIRECTION ( 'NONE',  ( -6.505213034913038160E-19, -3.903127820947822896E-18, -1.000000000000000000 ) ) ;
#18768=CARTESIAN_POINT ( 'NONE',  ( 2.220446049250313081E-13, -2.498001805406602216E-13, -6.859353255829918616 ) ) ;
#18771=AXIS2_PLACEMENT_3D ( 'NONE', #21205, #19487, #3792 ) ;
#18775=ORIENTED_EDGE ( 'NONE', *, *, #1179, .T. ) ;
#18777=CARTESIAN_POINT ( 'NONE',  ( -7.711478842616386942, 31.57187188083510065, -2.999999999999971578 ) ) ;
#18778=ORIENTED_EDGE ( 'NONE', *, *, #18490, .T. ) ;
#18784=CARTESIAN_POINT ( 'NONE',  ( 2.220446049250313081E-13, -8.326672684688674053E-14, 2.800654218530498785 ) ) ;
#18788=DIRECTION ( 'NONE',  ( -6.505213034913038160E-19, -3.903127820947822896E-18, -1.000000000000000000 ) ) ;
#18795=DIRECTION ( 'NONE',  ( 6.505213034913038160E-19, 3.903127820947822896E-18, 1.000000000000000000 ) ) ;
#18798=ADVANCED_FACE ( 'NONE', ( #8267 ), #22483, .T. ) ;
#18799=EDGE_LOOP ( 'NONE', ( #9133, #18520, #10504, #12568 ) ) ;
#18800=AXIS2_PLACEMENT_3D ( 'NONE', #1769, #22635, #1652 ) ;
#18802=VECTOR ( 'NONE', #13140, 1000.000000000000000 ) ;
#18805=ORIENTED_EDGE ( 'NONE', *, *, #16160, .F. ) ;
#18806=DIRECTION ( 'NONE',  ( -1.000000000000000000, 0.000000000000000000, 0.000000000000000000 ) ) ;
#18807=EDGE_CURVE ( 'NONE', #4282, #14096, #14355, .T. ) ;
#18812=VERTEX_POINT ( 'NONE', #17192 ) ;
#18813=CARTESIAN_POINT ( 'NONE',  ( 25.34312177887374062, -20.17230487860835453, -6.999999999999950262 ) ) ;
#18814=CYLINDRICAL_SURFACE ( 'NONE', #18579, 19.11328065563151668 ) ;
#18815=VERTEX_POINT ( 'NONE', #1391 ) ;
#18822=VERTEX_POINT ( 'NONE', #15236 ) ;
#18823=DIRECTION ( 'NONE',  ( -1.000000000000000000, 0.000000000000000000, 0.000000000000000000 ) ) ;
#18825=CARTESIAN_POINT ( 'NONE',  ( 5.074925817841801745, -32.10132595304126824, 3.000000000000023537 ) ) ;
#18835=ORIENTED_EDGE ( 'NONE', *, *, #18415, .F. ) ;
#18845=CARTESIAN_POINT ( 'NONE',  ( 5.551115123125782702E-14, -1.387778780781445676E-13, -5.749999999999949374 ) ) ;
#18847=EDGE_LOOP ( 'NONE', ( #1076, #19052, #16870, #13650 ) ) ;
#18851=DIRECTION ( 'NONE',  ( -1.000000000000000000, 0.000000000000000000, 0.000000000000000000 ) ) ;
#18852=VECTOR ( 'NONE', #7546, 1000.000000000000000 ) ;
#18862=AXIS2_PLACEMENT_3D ( 'NONE', #29, #21000, #5625 ) ;
#18866=CARTESIAN_POINT ( 'NONE',  ( -24.73600648735095575, 27.19760187735845136, -2.800654218530457484 ) ) ;
#18871=AXIS2_PLACEMENT_3D ( 'NONE', #411, #10488, #19338 ) ;
#18873=CARTESIAN_POINT ( 'NONE',  ( -34.09180625983476176, -10.01331137436164020, -3.000000000000002220 ) ) ;
#18874=CARTESIAN_POINT ( 'NONE',  ( 9.708269511265410046, -33.52953626616050542, -2.999999999999971578 ) ) ;
#18875=DIRECTION ( 'NONE',  ( -1.000000000000000000, -1.208970125616063644E-17, 0.000000000000000000 ) ) ;
#18877=EDGE_LOOP ( 'NONE', ( #4314, #346 ) ) ;
#18878=DIRECTION ( 'NONE',  ( 6.505213034913038160E-19, 3.903127820947822896E-18, 1.000000000000000000 ) ) ;
#18880=AXIS2_PLACEMENT_3D ( 'NONE', #7267, #19526, #19424 ) ;
#18881=ORIENTED_EDGE ( 'NONE', *, *, #9809, .T. ) ;
#18882=DIRECTION ( 'NONE',  ( -1.000000000000000000, -8.894490888754757555E-15, 0.000000000000000000 ) ) ;
#18887=VERTEX_POINT ( 'NONE', #8050 ) ;
#18892=FACE_OUTER_BOUND ( 'NONE', #17129, .T. ) ;
#18904=CIRCLE ( 'NONE', #11949, 0.9999999999999974465 ) ;
#18906=ORIENTED_EDGE ( 'NONE', *, *, #19425, .T. ) ;
#18907=DIRECTION ( 'NONE',  ( -6.505213034913038160E-19, -3.903127820947822896E-18, -1.000000000000000000 ) ) ;
#18914=CARTESIAN_POINT ( 'NONE',  ( -32.40961249803532240, 2.422192751863672111, -2.999999999999960920 ) ) ;
#18916=ORIENTED_EDGE ( 'NONE', *, *, #16230, .F. ) ;
#18917=TOROIDAL_SURFACE ( 'NONE', #7196, 34.90673715956759082, 8.750000000000000000 ) ;
#18919=ORIENTED_EDGE ( 'NONE', *, *, #2266, .F. ) ;
#18928=CARTESIAN_POINT ( 'NONE',  ( -25.58633464742622721, -23.74488952252778873, 3.000000000000002665 ) ) ;
#18929=ORIENTED_EDGE ( 'NONE', *, *, #14097, .T. ) ;
#18931=VECTOR ( 'NONE', #20965, 1000.000000000000000 ) ;
#18932=FACE_OUTER_BOUND ( 'NONE', #8831, .T. ) ;
#18934=ORIENTED_EDGE ( 'NONE', *, *, #9245, .F. ) ;
#18936=ORIENTED_EDGE ( 'NONE', *, *, #12017, .F. ) ;
#18938=DIRECTION ( 'NONE',  ( 6.505213034913038160E-19, 3.903127820947822896E-18, 1.000000000000000000 ) ) ;
#18941=DIRECTION ( 'NONE',  ( 6.505213034913038160E-19, 3.903127820947822896E-18, 1.000000000000000000 ) ) ;
#18949=CIRCLE ( 'NONE', #16379, 34.90673715956759082 ) ;
#18956=CARTESIAN_POINT ( 'NONE',  ( -11.93972437435537870, -29.14949368109895289, -6.999999999999992006 ) ) ;
#18960=SHAPE_REPRESENTATION ( 'GEAR', ( #18273 ), #12407 ) ;
#18963=DIRECTION ( 'NONE',  ( 6.505213034913038160E-19, 3.903127820947822896E-18, 1.000000000000000000 ) ) ;
#18965=CIRCLE ( 'NONE', #16376, 19.11328065563152023 ) ;
#18968=DIRECTION ( 'NONE',  ( -6.505213034913038160E-19, -3.903127820947822896E-18, -1.000000000000000000 ) ) ;
#18970=DIRECTION ( 'NONE',  ( 1.000000000000000000, 1.208970125616063028E-17, 0.000000000000000000 ) ) ;
#18973=CIRCLE ( 'NONE', #16400, 1.000000000000000888 ) ;
#18975=DIRECTION ( 'NONE',  ( -1.000000000000000000, 0.000000000000000000, 0.000000000000000000 ) ) ;
#18980=ORIENTED_EDGE ( 'NONE', *, *, #15566, .T. ) ;
#18986=ORIENTED_EDGE ( 'NONE', *, *, #12408, .F. ) ;
#18987=DIRECTION ( 'NONE',  ( -1.000000000000000000, -1.208970125616063644E-17, 0.000000000000000000 ) ) ;
#18988=CARTESIAN_POINT ( 'NONE',  ( 5.551115123125782702E-14, -1.387778780781445676E-13, -5.749999999999949374 ) ) ;
#18992=VECTOR ( 'NONE', #20704, 1000.000000000000000 ) ;
#18993=VERTEX_POINT ( 'NONE', #1734 ) ;
#18996=ADVANCED_FACE ( 'NONE', ( #13958 ), #17835, .T. ) ;
#18998=EDGE_CURVE ( 'NONE', #17558, #10689, #20979, .T. ) ;
#19001=EDGE_LOOP ( 'NONE', ( #11109, #15818, #20730, #21407 ) ) ;
#19004=ORIENTED_EDGE ( 'NONE', *, *, #3594, .T. ) ;
#19005=CARTESIAN_POINT ( 'NONE',  ( -16.06969024216335740, -19.15111107797456924, -2.999999999999995559 ) ) ;
#19006=DIRECTION ( 'NONE',  ( -1.000000000000000000, 0.000000000000000000, 0.000000000000000000 ) ) ;
#19012=CARTESIAN_POINT ( 'NONE',  ( 2.220446049250313081E-13, -2.498001805406602216E-13, -6.859353255829918616 ) ) ;
#19013=CARTESIAN_POINT ( 'NONE',  ( 23.65408649739131164, 22.22891329980528141, -6.999999999999950262 ) ) ;
#19020=AXIS2_PLACEMENT_3D ( 'NONE', #19763, #18023, #4069 ) ;
#19021=ORIENTED_EDGE ( 'NONE', *, *, #18575, .T. ) ;
#19025=CARTESIAN_POINT ( 'NONE',  ( 7.463862311151453710, 35.99819890246955367, 2.800654218530485018 ) ) ;
#19028=ADVANCED_FACE ( 'NONE', ( #9330 ), #6133, .T. ) ;
#19029=DIRECTION ( 'NONE',  ( 6.505213034913038160E-19, 3.903127820947822896E-18, 1.000000000000000000 ) ) ;
#19030=DIRECTION ( 'NONE',  ( -6.505213034913038160E-19, -3.903127820947822896E-18, -1.000000000000000000 ) ) ;
#19034=ORIENTED_EDGE ( 'NONE', *, *, #8808, .T. ) ;
#19035=VECTOR ( 'NONE', #5805, 1000.000000000000000 ) ;
#19040=CARTESIAN_POINT ( 'NONE',  ( 14.29266125237896290, -28.07080038625095497, -2.999999999999971578 ) ) ;
#19044=DIRECTION ( 'NONE',  ( 6.505213034913038160E-19, 3.903127820947822896E-18, 1.000000000000000000 ) ) ;
#19047=DIRECTION ( 'NONE',  ( 6.505213034913038160E-19, 3.903127820947822896E-18, 1.000000000000000000 ) ) ;
#19048=CARTESIAN_POINT ( 'NONE',  ( -9.576564013118654017, 26.31139338200516420, -2.999999999999978240 ) ) ;
#19049=VECTOR ( 'NONE', #16670, 1000.000000000000000 ) ;
#19050=DIRECTION ( 'NONE',  ( -6.505213034913038160E-19, -3.903127820947822896E-18, -1.000000000000000000 ) ) ;
#19052=ORIENTED_EDGE ( 'NONE', *, *, #11440, .F. ) ;
#19056=CARTESIAN_POINT ( 'NONE',  ( -6.742883674876437361, -34.24928931925796860, 3.000000000000002665 ) ) ;
#19060=ORIENTED_EDGE ( 'NONE', *, *, #13408, .F. ) ;
#19071=ORIENTED_EDGE ( 'NONE', *, *, #11796, .T. ) ;
#19075=EDGE_CURVE ( 'NONE', #3715, #66, #12861, .T. ) ;
#19078=ORIENTED_EDGE ( 'NONE', *, *, #22598, .T. ) ;
#19080=CARTESIAN_POINT ( 'NONE',  ( -8.485281374238567764, -3.000000000000002665, -6.859353255829953255 ) ) ;
#19082=CARTESIAN_POINT ( 'NONE',  ( 34.13396246814587442, -14.93538271375421900, 3.000000000000023537 ) ) ;
#19087=AXIS2_PLACEMENT_3D ( 'NONE', #17785, #14329, #5635 ) ;
#19091=EDGE_CURVE ( 'NONE', #15368, #8029, #4563, .T. ) ;
#19096=DIRECTION ( 'NONE',  ( 6.505213034913038160E-19, 3.903127820947822896E-18, 1.000000000000000000 ) ) ;
#19098=ADVANCED_FACE ( 'NONE', ( #20773 ), #5192, .T. ) ;
#19102=FACE_OUTER_BOUND ( 'NONE', #16791, .T. ) ;
#19103=CARTESIAN_POINT ( 'NONE',  ( 1.110223024625156540E-13, -27.99999999999996803, -4.999999999999948486 ) ) ;
#19107=FACE_OUTER_BOUND ( 'NONE', #13995, .T. ) ;
#19108=DIRECTION ( 'NONE',  ( -6.505213034913038160E-19, -3.903127820947822896E-18, -1.000000000000000000 ) ) ;
#19110=DIRECTION ( 'NONE',  ( 6.505213034913038160E-19, 3.903127820947822896E-18, 1.000000000000000000 ) ) ;
#19114=CARTESIAN_POINT ( 'NONE',  ( 28.95348479018588961, -14.76298474240531000, -2.999999999999999112 ) ) ;
#19123=DIRECTION ( 'NONE',  ( 6.505213034913038160E-19, 3.903127820947822896E-18, 1.000000000000000000 ) ) ;
#19129=ORIENTED_EDGE ( 'NONE', *, *, #19091, .T. ) ;
#19137=ORIENTED_EDGE ( 'NONE', *, *, #9026, .T. ) ;
#19138=AXIS2_PLACEMENT_3D ( 'NONE', #13652, #1534, #20788 ) ;
#19139=EDGE_CURVE ( 'NONE', #1737, #260, #3591, .T. ) ;
#19141=DIRECTION ( 'NONE',  ( -6.505213034913038160E-19, -3.903127820947822896E-18, -1.000000000000000000 ) ) ;
#19142=VECTOR ( 'NONE', #17583, 1000.000000000000000 ) ;
#19143=ORIENTED_EDGE ( 'NONE', *, *, #20577, .T. ) ;
#19149=CARTESIAN_POINT ( 'NONE',  ( -7.474202570535936729, 30.60042966911702322, -7.000000000000006217 ) ) ;
#19150=ADVANCED_FACE ( 'NONE', ( #18717 ), #22499, .F. ) ;
#19154=VERTEX_POINT ( 'NONE', #19056 ) ;
#19155=DIRECTION ( 'NONE',  ( -1.000000000000000000, 0.000000000000000000, 0.000000000000000000 ) ) ;
#19161=DIRECTION ( 'NONE',  ( 6.505213034913038160E-19, 3.903127820947822896E-18, 1.000000000000000000 ) ) ;
#19166=CARTESIAN_POINT ( 'NONE',  ( -21.00948735876881202, -24.79619811426206510, -2.999999999999995559 ) ) ;
#19170=DIRECTION ( 'NONE',  ( -6.505213034913038160E-19, -3.903127820947822896E-18, -1.000000000000000000 ) ) ;
#19174=CIRCLE ( 'NONE', #13275, 20.00000000000002132 ) ;
#19176=ORIENTED_EDGE ( 'NONE', *, *, #11948, .T. ) ;
#19180=ORIENTED_EDGE ( 'NONE', *, *, #15433, .T. ) ;
#19187=CARTESIAN_POINT ( 'NONE',  ( 3.330669073875469621E-13, -1.110223024625156540E-13, -2.999999999999971578 ) ) ;
#19189=ORIENTED_EDGE ( 'NONE', *, *, #21612, .T. ) ;
#19195=ORIENTED_EDGE ( 'NONE', *, *, #13226, .T. ) ;
#19203=CARTESIAN_POINT ( 'NONE',  ( -27.19760187735867518, -24.73600648735113694, -2.800654218530429507 ) ) ;
#19207=ORIENTED_EDGE ( 'NONE', *, *, #2962, .F. ) ;
#19211=LINE ( 'NONE', #17134, #12521 ) ;
#19212=DIRECTION ( 'NONE',  ( -1.000000000000000000, -5.332156527697367955E-15, 0.000000000000000000 ) ) ;
#19220=CARTESIAN_POINT ( 'NONE',  ( 33.51030287062373247, 15.12081897056669000, -2.800654218530485018 ) ) ;
#19222=ORIENTED_EDGE ( 'NONE', *, *, #8808, .F. ) ;
#19224=EDGE_CURVE ( 'NONE', #15616, #20003, #5515, .T. ) ;
#19233=ORIENTED_EDGE ( 'NONE', *, *, #19563, .F. ) ;
#19234=CIRCLE ( 'NONE', #22165, 0.9999999999999956701 ) ;
#19236=CARTESIAN_POINT ( 'NONE',  ( -33.51030287062373247, -15.12081897056669000, -2.800654218530457484 ) ) ;
#19237=ORIENTED_EDGE ( 'NONE', *, *, #19406, .T. ) ;
#19241=DIRECTION ( 'NONE',  ( 6.505213034913038160E-19, 3.903127820947822896E-18, 1.000000000000000000 ) ) ;
#19242=AXIS2_PLACEMENT_3D ( 'NONE', #12942, #20181, #4487 ) ;
#19246=CIRCLE ( 'NONE', #3888, 34.90673715956759082 ) ;
#19249=DIRECTION ( 'NONE',  ( 1.000000000000000000, 1.208970125616063028E-17, 0.000000000000000000 ) ) ;
#19250=CIRCLE ( 'NONE', #4249, 19.11328065563151668 ) ;
#19252=EDGE_CURVE ( 'NONE', #13545, #2882, #11637, .T. ) ;
#19257=CARTESIAN_POINT ( 'NONE',  ( 22.22891329980558695, -23.65408649739134006, -6.999999999999999112 ) ) ;
#19260=AXIS2_PLACEMENT_3D ( 'NONE', #7603, #16767, #16650 ) ;
#19269=DIRECTION ( 'NONE',  ( 6.505213034913038160E-19, 3.903127820947822896E-18, 1.000000000000000000 ) ) ;
#19273=ORIENTED_EDGE ( 'NONE', *, *, #8080, .F. ) ;
#19274=CARTESIAN_POINT ( 'NONE',  ( 4.170748987303435129, -34.65667543218869895, 2.999999999999999112 ) ) ;
#19280=DIRECTION ( 'NONE',  ( -6.505213034913038160E-19, -3.903127820947822896E-18, -1.000000000000000000 ) ) ;
#19293=VERTEX_POINT ( 'NONE', #4484 ) ;
#19296=DIRECTION ( 'NONE',  ( -1.000000000000000000, -1.208970125616062874E-17, 0.000000000000000000 ) ) ;
#19297=CYLINDRICAL_SURFACE ( 'NONE', #18800, 36.76383501243555685 ) ;
#19299=DIRECTION ( 'NONE',  ( 1.000000000000000000, 0.000000000000000000, 0.000000000000000000 ) ) ;
#19305=B_SPLINE_CURVE_WITH_KNOTS ( 'NONE', 3,
 ( #13558, #10018, #18635, #2940 ),
 .UNSPECIFIED., .F., .F.,
 ( 4, 4 ),
 ( 9.715086428218796083E-07, 0.001929643240674198870 ),
 .UNSPECIFIED. ) ;
#19314=CIRCLE ( 'NONE', #10862, 34.90673715956759082 ) ;
#19316=LINE ( 'NONE', #3506, #7062 ) ;
#19323=EDGE_CURVE ( 'NONE', #6092, #5279, #8252, .T. ) ;
#19324=CIRCLE ( 'NONE', #6280, 36.76383501243555685 ) ;
#19325=ORIENTED_EDGE ( 'NONE', *, *, #12490, .T. ) ;
#19330=CIRCLE ( 'NONE', #12355, 31.50000000000000711 ) ;
#19331=LINE ( 'NONE', #3638, #17510 ) ;
#19332=DIRECTION ( 'NONE',  ( -6.505213034913038160E-19, -3.903127820947822896E-18, -1.000000000000000000 ) ) ;
#19336=CARTESIAN_POINT ( 'NONE',  ( 22.26748298433264850, -22.28024240313505899, -2.999999999999971578 ) ) ;
#19338=DIRECTION ( 'NONE',  ( -1.000000000000000000, -1.208970125616060101E-17, 6.505213034913038160E-19 ) ) ;
#19341=CIRCLE ( 'NONE', #8349, 36.76383501243555685 ) ;
#19349=VERTEX_POINT ( 'NONE', #4118 ) ;
#19350=ORIENTED_EDGE ( 'NONE', *, *, #16805, .F. ) ;
#19352=CARTESIAN_POINT ( 'NONE',  ( 31.67162468656012209, 14.67611967928900185, -2.999999999999971578 ) ) ;
#19367=LINE ( 'NONE', #6987, #18931 ) ;
#19373=DIRECTION ( 'NONE',  ( -1.000000000000000000, -2.486827044406942538E-14, 0.000000000000000000 ) ) ;
#19376=ADVANCED_FACE ( 'NONE', ( #4460 ), #556, .F. ) ;
#19379=VERTEX_POINT ( 'NONE', #4352 ) ;
#19382=( GEOMETRIC_REPRESENTATION_CONTEXT ( 3 ) GLOBAL_UNCERTAINTY_ASSIGNED_CONTEXT ( ( #8069 ) ) GLOBAL_UNIT_ASSIGNED_CONTEXT ( ( #3672, #9035, #15895 ) ) REPRESENTATION_CONTEXT ( 'NONE', 'WORKASPACE' ) );
#19387=ORIENTED_EDGE ( 'NONE', *, *, #19534, .F. ) ;
#19390=DIRECTION ( 'NONE',  ( 6.505213034913038160E-19, 3.903127820947822896E-18, 1.000000000000000000 ) ) ;
#19391=DIRECTION ( 'NONE',  ( -1.000000000000000000, 4.350865286404990634E-14, 0.000000000000000000 ) ) ;
#19392=ORIENTED_EDGE ( 'NONE', *, *, #2889, .T. ) ;
#19394=CARTESIAN_POINT ( 'NONE',  ( 33.46652738560686657, -11.93772187171692245, -2.999999999999998224 ) ) ;
#19396=ORIENTED_EDGE ( 'NONE', *, *, #4758, .F. ) ;
#19400=ADVANCED_FACE ( 'NONE', ( #17972, #11329, #7666, #18313, #2632 ), #16589, .T. ) ;
#19404=VERTEX_POINT ( 'NONE', #899 ) ;
#19405=EDGE_CURVE ( 'NONE', #14751, #14834, #13094, .T. ) ;
#19406=EDGE_CURVE ( 'NONE', #31, #14783, #19341, .T. ) ;
#19408=VERTEX_POINT ( 'NONE', #13697 ) ;
#19414=ORIENTED_EDGE ( 'NONE', *, *, #19588, .T. ) ;
#19418=CARTESIAN_POINT ( 'NONE',  ( 0.8615617109688762376, 36.14854559161343417, -2.932164912090547748 ) ) ;
#19419=DIRECTION ( 'NONE',  ( -1.000000000000000000, -1.208970125616044077E-17, 0.000000000000000000 ) ) ;
#19421=VERTEX_POINT ( 'NONE', #22439 ) ;
#19424=DIRECTION ( 'NONE',  ( -1.000000000000000000, -1.208970125616046080E-17, 6.505213034913038160E-19 ) ) ;
#19425=EDGE_CURVE ( 'NONE', #22614, #3371, #22216, .T. ) ;
#19430=AXIS2_PLACEMENT_3D ( 'NONE', #21179, #7418, #5480 ) ;
#19431=DIRECTION ( 'NONE',  ( 1.000000000000000000, 0.000000000000000000, 0.000000000000000000 ) ) ;
#19432=EDGE_CURVE ( 'NONE', #12412, #12073, #16394, .T. ) ;
#19434=VERTEX_POINT ( 'NONE', #20715 ) ;
#19435=VERTEX_POINT ( 'NONE', #1349 ) ;
#19438=CARTESIAN_POINT ( 'NONE',  ( 2.775557561562891351E-14, -2.775557561562891351E-14, 2.999999999999999112 ) ) ;
#19441=CARTESIAN_POINT ( 'NONE',  ( -26.64365646977254087, -17.09029715894938661, 3.000000000000012879 ) ) ;
#19443=ADVANCED_FACE ( 'NONE', ( #3191 ), #18602, .T. ) ;
#19444=AXIS2_PLACEMENT_3D ( 'NONE', #21684, #2778, #13400 ) ;
#19446=VERTEX_POINT ( 'NONE', #13819 ) ;
#19448=CARTESIAN_POINT ( 'NONE',  ( 0.6841746959068695233, 36.75746821813305587, 2.800654218530485018 ) ) ;
#19451=ADVANCED_FACE ( 'NONE', ( #3312 ), #10493, .F. ) ;
#19458=B_SPLINE_CURVE_WITH_KNOTS ( 'NONE', 3,
 ( #4679, #13010, #11542, #20374 ),
 .UNSPECIFIED., .F., .F.,
 ( 4, 4 ),
 ( 0.001875451646902865028, 0.003761979286331341814 ),
 .UNSPECIFIED. ) ;
#19459=ORIENTED_EDGE ( 'NONE', *, *, #21113, .T. ) ;
#19462=DIRECTION ( 'NONE',  ( -1.000000000000000000, -1.208970125616060101E-17, 6.505213034913038160E-19 ) ) ;
#19466=CARTESIAN_POINT ( 'NONE',  ( -27.64365646977265456, -17.09029715894952517, -2.999999999999981792 ) ) ;
#19467=ADVANCED_BREP_SHAPE_REPRESENTATION ( '', ( #18090, #18273 ), #12407 ) ;
#19468=ORIENTED_EDGE ( 'NONE', *, *, #12096, .T. ) ;
#19474=CARTESIAN_POINT ( 'NONE',  ( -13.83143812983099430, 29.36548507648012318, -7.000000000000006217 ) ) ;
#19476=ADVANCED_FACE ( 'NONE', ( #14146 ), #22682, .F. ) ;
#19478=AXIS2_PLACEMENT_3D ( 'NONE', #12318, #10590, #3636 ) ;
#19479=ORIENTED_EDGE ( 'NONE', *, *, #7341, .T. ) ;
#19481=ORIENTED_EDGE ( 'NONE', *, *, #13504, .T. ) ;
#19483=CARTESIAN_POINT ( 'NONE',  ( 15.02862401740831544, 32.75570538720759828, 2.999999999999995559 ) ) ;
#19485=CARTESIAN_POINT ( 'NONE',  ( 14.74639653023232455, -28.96193690644940943, -6.999999999999944045 ) ) ;
#19487=DIRECTION ( 'NONE',  ( -6.505213034913038160E-19, -3.903127820947822896E-18, -1.000000000000000000 ) ) ;
#19489=ORIENTED_EDGE ( 'NONE', *, *, #8536, .T. ) ;
#19493=AXIS2_PLACEMENT_3D ( 'NONE', #2811, #11732, #1303 ) ;
#19495=ORIENTED_EDGE ( 'NONE', *, *, #14587, .F. ) ;
#19499=TOROIDAL_SURFACE ( 'NONE', #8163, 34.90673715956759082, 8.750000000000000000 ) ;
#19500=ORIENTED_EDGE ( 'NONE', *, *, #8740, .F. ) ;
#19505=EDGE_CURVE ( 'NONE', #12184, #15016, #19697, .T. ) ;
#19507=ORIENTED_EDGE ( 'NONE', *, *, #15267, .T. ) ;
#19511=LINE ( 'NONE', #5524, #6651 ) ;
#19513=DIRECTION ( 'NONE',  ( -6.505213034913038160E-19, -3.903127820947822896E-18, -1.000000000000000000 ) ) ;
#19515=ORIENTED_EDGE ( 'NONE', *, *, #16066, .T. ) ;
#19517=DIRECTION ( 'NONE',  ( 6.505213034913038160E-19, 3.903127820947822896E-18, 1.000000000000000000 ) ) ;
#19519=CARTESIAN_POINT ( 'NONE',  ( -14.14132741310376851, -16.85297774861785314, -4.999999999999955591 ) ) ;
#19523=ADVANCED_FACE ( 'NONE', ( #16457 ), #15287, .T. ) ;
#19526=DIRECTION ( 'NONE',  ( -6.505213034913038160E-19, -3.903127820947822896E-18, -1.000000000000000000 ) ) ;
#19528=CARTESIAN_POINT ( 'NONE',  ( -25.34312177887334983, 20.17230487860824439, -2.999999999999971578 ) ) ;
#19529=FACE_OUTER_BOUND ( 'NONE', #10302, .T. ) ;
#19530=DIRECTION ( 'NONE',  ( 6.505213034913038160E-19, 3.903127820947822896E-18, 1.000000000000000000 ) ) ;
#19533=DIRECTION ( 'NONE',  ( 1.000000000000000000, 1.208970125616053784E-17, 0.000000000000000000 ) ) ;
#19534=EDGE_CURVE ( 'NONE', #14442, #817, #12720, .T. ) ;
#19536=AXIS2_PLACEMENT_3D ( 'NONE', #8707, #13950, #2 ) ;
#19537=CARTESIAN_POINT ( 'NONE',  ( -16.99647590252638452, -30.48934413892778750, 2.999999999999999112 ) ) ;
#19543=B_SPLINE_CURVE_WITH_KNOTS ( 'NONE', 3,
 ( #2450, #5645, #14575, #12742 ),
 .UNSPECIFIED., .F., .F.,
 ( 4, 4 ),
 ( 9.715086412473486974E-07, 0.001929643240672463496 ),
 .UNSPECIFIED. ) ;
#19548=EDGE_CURVE ( 'NONE', #5940, #15936, #9456, .T. ) ;
#19549=CARTESIAN_POINT ( 'NONE',  ( -22.22891329980540576, 23.65408649739122993, -7.000000000000006217 ) ) ;
#19552=EDGE_CURVE ( 'NONE', #8421, #4768, #8708, .T. ) ;
#19562=DIRECTION ( 'NONE',  ( -1.000000000000000000, -1.208970125616062874E-17, 0.000000000000000000 ) ) ;
#19563=EDGE_CURVE ( 'NONE', #13710, #15616, #13462, .T. ) ;
#19564=VERTEX_POINT ( 'NONE', #17069 ) ;
#19567=ORIENTED_EDGE ( 'NONE', *, *, #16086, .T. ) ;
#19571=AXIS2_PLACEMENT_3D ( 'NONE', #9265, #20157, #21764 ) ;
#19572=DIRECTION ( 'NONE',  ( -6.505213034913038160E-19, -3.903127820947822896E-18, -1.000000000000000000 ) ) ;
#19577=DIRECTION ( 'NONE',  ( 1.000000000000000000, 1.208970125616063182E-17, 0.000000000000000000 ) ) ;
#19584=AXIS2_PLACEMENT_3D ( 'NONE', #11004, #5856, #20170 ) ;
#19585=CARTESIAN_POINT ( 'NONE',  ( 20.36304159388385671, 24.03323817228478276, 3.000000000000023537 ) ) ;
#19587=B_SPLINE_CURVE_WITH_KNOTS ( 'NONE', 3,
 ( #6324, #13068, #6104, #11597 ),
 .UNSPECIFIED., .F., .F.,
 ( 4, 4 ),
 ( 0.001875451646902612842, 0.003761979286330821397 ),
 .UNSPECIFIED. ) ;
#19588=EDGE_CURVE ( 'NONE', #6416, #16045, #20521, .T. ) ;
#19592=EDGE_CURVE ( 'NONE', #13346, #11018, #3627, .T. ) ;
#19596=AXIS2_PLACEMENT_3D ( 'NONE', #13216, #21616, #6258 ) ;
#19598=CARTESIAN_POINT ( 'NONE',  ( 11.85401191286916678, 32.83234229683709771, -2.999999999999995559 ) ) ;
#19604=VECTOR ( 'NONE', #2452, 1000.000000000000000 ) ;
#19605=CARTESIAN_POINT ( 'NONE',  ( -28.13960001536965194, 21.69517388068233998, -2.999999999999999112 ) ) ;
#19610=CARTESIAN_POINT ( 'NONE',  ( 3.330669073875469621E-13, -1.110223024625156540E-13, -2.999999999999971578 ) ) ;
#19615=CARTESIAN_POINT ( 'NONE',  ( 1.942890293094023946E-13, -8.326672684688674053E-14, 4.999999999999993783 ) ) ;
#19616=DIRECTION ( 'NONE',  ( 6.505213034913038160E-19, 3.903127820947822896E-18, 1.000000000000000000 ) ) ;
#19617=AXIS2_PLACEMENT_3D ( 'NONE', #13746, #19047, #3241 ) ;
#19618=AXIS2_PLACEMENT_3D ( 'NONE', #2820, #9804, #16795 ) ;
#19619=CIRCLE ( 'NONE', #16702, 3.000000000000000888 ) ;
#19623=EDGE_LOOP ( 'NONE', ( #5028, #3428, #7023, #7660 ) ) ;
#19630=ORIENTED_EDGE ( 'NONE', *, *, #4579, .F. ) ;
#19631=DIRECTION ( 'NONE',  ( -1.000000000000000000, -1.208970125616081209E-17, 0.000000000000000000 ) ) ;
#19634=AXIS2_PLACEMENT_3D ( 'NONE', #16872, #20540, #1170 ) ;
#19640=AXIS2_PLACEMENT_3D ( 'NONE', #6052, #18310, #18198 ) ;
#19641=CARTESIAN_POINT ( 'NONE',  ( 36.54278193890331039, 4.025500340002458266, 2.800654218530485018 ) ) ;
#19642=ORIENTED_EDGE ( 'NONE', *, *, #11663, .T. ) ;
#19643=B_SPLINE_CURVE_WITH_KNOTS ( 'NONE', 3,
 ( #12130, #22347, #8358, #10285 ),
 .UNSPECIFIED., .F., .F.,
 ( 4, 4 ),
 ( 9.715086409868104685E-07, 0.001929643240672413622 ),
 .UNSPECIFIED. ) ;
#19645=ORIENTED_EDGE ( 'NONE', *, *, #16055, .T. ) ;
#19647=DIRECTION ( 'NONE',  ( -1.000000000000000000, -1.208970125616044077E-17, 0.000000000000000000 ) ) ;
#19648=CARTESIAN_POINT ( 'NONE',  ( -15.62726112422577174, -28.45046755804897387, -6.999999999999971578 ) ) ;
#19649=EDGE_CURVE ( 'NONE', #1729, #8443, #13727, .T. ) ;
#19659=ORIENTED_EDGE ( 'NONE', *, *, #9372, .F. ) ;
#19660=VERTEX_POINT ( 'NONE', #9668 ) ;
#19663=DIRECTION ( 'NONE',  ( 6.505213034913038160E-19, 3.903127820947822896E-18, 1.000000000000000000 ) ) ;
#19669=EDGE_LOOP ( 'NONE', ( #10320, #4302, #22164, #14865 ) ) ;
#19674=CARTESIAN_POINT ( 'NONE',  ( 4.177897941877333210, -34.13396246814587442, -6.999999999999950262 ) ) ;
#19675=CIRCLE ( 'NONE', #9785, 19.11328065563151668 ) ;
#19681=CARTESIAN_POINT ( 'NONE',  ( 2.775557561562891351E-13, 3.000000000000002665, -5.000000000000004441 ) ) ;
#19683=CIRCLE ( 'NONE', #15998, 1.000000000000000888 ) ;
#19687=CIRCLE ( 'NONE', #21139, 1.000000000000000888 ) ;
#19689=ORIENTED_EDGE ( 'NONE', *, *, #14942, .T. ) ;
#19691=FACE_OUTER_BOUND ( 'NONE', #21061, .T. ) ;
#19692=CARTESIAN_POINT ( 'NONE',  ( -35.43359966464135624, 7.197698565811587734, 2.932460736555813963 ) ) ;
#19693=EDGE_CURVE ( 'NONE', #11286, #5560, #21538, .T. ) ;
#19694=EDGE_CURVE ( 'NONE', #20280, #12118, #4677, .T. ) ;
#19697=CIRCLE ( 'NONE', #9811, 19.11328065563150957 ) ;
#19702=ORIENTED_EDGE ( 'NONE', *, *, #13343, .F. ) ;
#19703=CARTESIAN_POINT ( 'NONE',  ( -19.05255888325766023, 10.99999999999970512, -5.000000000000004441 ) ) ;
#19704=VECTOR ( 'NONE', #7401, 1000.000000000000000 ) ;
#19706=CYLINDRICAL_SURFACE ( 'NONE', #17922, 19.11328065563152023 ) ;
#19713=DIRECTION ( 'NONE',  ( 1.000000000000000000, 0.000000000000000000, 0.000000000000000000 ) ) ;
#19719=LINE ( 'NONE', #2283, #9301 ) ;
#19720=AXIS2_PLACEMENT_3D ( 'NONE', #9099, #17916, #18140 ) ;
#19724=CARTESIAN_POINT ( 'NONE',  ( -28.45046755804882110, 15.62726112422596714, 2.999999999999995559 ) ) ;
#19726=EDGE_LOOP ( 'NONE', ( #19748, #22042, #1659, #13799 ) ) ;
#19728=LINE ( 'NONE', #2291, #2492 ) ;
#19730=CARTESIAN_POINT ( 'NONE',  ( -21.94328778841581595, -28.73472116836736134, 2.932969818539080009 ) ) ;
#19737=DIRECTION ( 'NONE',  ( -1.000000000000000000, -1.208970125616081209E-17, 0.000000000000000000 ) ) ;
#19738=CARTESIAN_POINT ( 'NONE',  ( -0.6841746959065087008, -36.75746821813308429, -2.800654218530457484 ) ) ;
#19747=VERTEX_POINT ( 'NONE', #2293 ) ;
#19748=ORIENTED_EDGE ( 'NONE', *, *, #22592, .F. ) ;
#19752=DIRECTION ( 'NONE',  ( -1.000000000000000000, 0.000000000000000000, 0.000000000000000000 ) ) ;
#19753=VERTEX_POINT ( 'NONE', #18408 ) ;
#19756=VERTEX_POINT ( 'NONE', #2185 ) ;
#19758=CYLINDRICAL_SURFACE ( 'NONE', #20699, 3.000000000000002665 ) ;
#19759=VERTEX_POINT ( 'NONE', #15069 ) ;
#19760=CARTESIAN_POINT ( 'NONE',  ( 2.775557561562891351E-14, -2.775557561562891351E-14, 2.999999999999999112 ) ) ;
#19761=EDGE_LOOP ( 'NONE', ( #12868, #18672, #2315, #7576 ) ) ;
#19763=CARTESIAN_POINT ( 'NONE',  ( -14.93538271375398274, -34.13396246814581758, 3.000000000000023537 ) ) ;
#19764=CARTESIAN_POINT ( 'NONE',  ( 15.12081897056669000, -33.51030287062373247, -2.800654218530457484 ) ) ;
#19765=ORIENTED_EDGE ( 'NONE', *, *, #20258, .F. ) ;
#19766=AXIS2_PLACEMENT_3D ( 'NONE', #7299, #21165, #5569 ) ;
#19768=DIRECTION ( 'NONE',  ( 6.505213034913038160E-19, 3.903127820947822896E-18, 1.000000000000000000 ) ) ;
#19771=ORIENTED_EDGE ( 'NONE', *, *, #7017, .F. ) ;
#19772=AXIS2_PLACEMENT_3D ( 'NONE', #15577, #9972, #6896 ) ;
#19773=VERTEX_POINT ( 'NONE', #14307 ) ;
#19774=ORIENTED_EDGE ( 'NONE', *, *, #4440, .T. ) ;
#19782=CARTESIAN_POINT ( 'NONE',  ( 7.474202570536131240, -30.60042966911724704, -2.999999999999999112 ) ) ;
#19786=LINE ( 'NONE', #13112, #1028 ) ;
#19789=EDGE_CURVE ( 'NONE', #15811, #19434, #16781, .T. ) ;
#19792=CARTESIAN_POINT ( 'NONE',  ( 22.98755168577434915, 22.97438720605740770, 2.999999999999999112 ) ) ;
#19801=DIRECTION ( 'NONE',  ( 1.000000000000000000, 0.000000000000000000, 0.000000000000000000 ) ) ;
#19804=DIRECTION ( 'NONE',  ( 6.505213034913038160E-19, 3.903127820947822896E-18, 1.000000000000000000 ) ) ;
#19806=CARTESIAN_POINT ( 'NONE',  ( 24.62019382530525391, -4.341204441673157888, -5.000000000000004441 ) ) ;
#19807=CARTESIAN_POINT ( 'NONE',  ( 14.30873905802343415, 28.06260833510301822, -2.999999999999971578 ) ) ;
#19808=EDGE_CURVE ( 'NONE', #18161, #1737, #2613, .T. ) ;
#19812=DIRECTION ( 'NONE',  ( 1.000000000000000000, 0.000000000000000000, 0.000000000000000000 ) ) ;
#19813=CARTESIAN_POINT ( 'NONE',  ( -22.22891329980515707, 23.65408649739117308, -2.999999999999992450 ) ) ;
#19815=VERTEX_POINT ( 'NONE', #5736 ) ;
#19817=CYLINDRICAL_SURFACE ( 'NONE', #16275, 19.11328065563152379 ) ;
#19820=VERTEX_POINT ( 'NONE', #5236 ) ;
#19822=AXIS2_PLACEMENT_3D ( 'NONE', #20634, #20870, #10303 ) ;
#19823=EDGE_CURVE ( 'NONE', #15170, #4760, #9421, .T. ) ;
#19827=CARTESIAN_POINT ( 'NONE',  ( 35.79662727779894738, -4.171001175319904775, -7.000000000000006217 ) ) ;
#19829=ORIENTED_EDGE ( 'NONE', *, *, #13148, .T. ) ;
#19833=VERTEX_POINT ( 'NONE', #6961 ) ;
#19834=CARTESIAN_POINT ( 'NONE',  ( -31.11077005834410159, 4.936596639065010450, -6.999999999999978684 ) ) ;
#19849=ORIENTED_EDGE ( 'NONE', *, *, #13301, .F. ) ;
#19850=ORIENTED_EDGE ( 'NONE', *, *, #16145, .F. ) ;
#19852=ORIENTED_EDGE ( 'NONE', *, *, #5467, .F. ) ;
#19853=DIRECTION ( 'NONE',  ( 6.505213034913038160E-19, 3.903127820947822896E-18, 1.000000000000000000 ) ) ;
#19855=AXIS2_PLACEMENT_3D ( 'NONE', #5260, #10284, #22346 ) ;
#19856=DIRECTION ( 'NONE',  ( 6.505213034913038160E-19, 3.903127820947822896E-18, 1.000000000000000000 ) ) ;
#19857=LINE ( 'NONE', #16168, #12794 ) ;
#19860=CARTESIAN_POINT ( 'NONE',  ( 7.474202570536158774, -30.60042966911724704, -7.000000000000006217 ) ) ;
#19864=CARTESIAN_POINT ( 'NONE',  ( 3.608224830031758756E-13, -2.775557561562891351E-14, -4.999999999999997335 ) ) ;
#19865=CARTESIAN_POINT ( 'NONE',  ( -21.00948735876881202, -24.79619811426206510, -2.999999999999995559 ) ) ;
#19872=CARTESIAN_POINT ( 'NONE',  ( 21.94328778841601491, 28.73472116836732582, 2.932969818539045814 ) ) ;
#19875=EDGE_LOOP ( 'NONE', ( #8778, #14850, #10876, #17679, #3349, #9465 ) ) ;
#19877=ORIENTED_EDGE ( 'NONE', *, *, #20384, .T. ) ;
#19880=CARTESIAN_POINT ( 'NONE',  ( 4.104665049622683526, -35.91964150878182238, -2.933296326616347205 ) ) ;
#19882=ADVANCED_FACE ( 'NONE', ( #3182 ), #8218, .T. ) ;
#19885=DIRECTION ( 'NONE',  ( -6.505213034913038160E-19, -3.903127820947822896E-18, -1.000000000000000000 ) ) ;
#19887=EDGE_LOOP ( 'NONE', ( #7618, #9098, #11015, #11892 ) ) ;
#19893=EDGE_CURVE ( 'NONE', #5375, #4097, #11651, .T. ) ;
#19894=CARTESIAN_POINT ( 'NONE',  ( -29.36548507648019424, -13.83143812983114707, -2.999999999999995559 ) ) ;
#19902=CIRCLE ( 'NONE', #6006, 34.90673715956759082 ) ;
#19904=ORIENTED_EDGE ( 'NONE', *, *, #17441, .F. ) ;
#19908=LINE ( 'NONE', #11075, #18158 ) ;
#19912=DIRECTION ( 'NONE',  ( -6.505213034913038160E-19, -3.903127820947822896E-18, -1.000000000000000000 ) ) ;
#19918=DIRECTION ( 'NONE',  ( -1.000000000000000000, 1.775147869274630931E-14, 0.000000000000000000 ) ) ;
#19920=CYLINDRICAL_SURFACE ( 'NONE', #19640, 1.000000000000000888 ) ;
#19921=CARTESIAN_POINT ( 'NONE',  ( 24.75236754129181449, 27.84804035626023477, 2.999999999999995559 ) ) ;
#19923=ORIENTED_EDGE ( 'NONE', *, *, #14736, .F. ) ;
#19928=ORIENTED_EDGE ( 'NONE', *, *, #69, .T. ) ;
#19931=EDGE_CURVE ( 'NONE', #17625, #15936, #111, .T. ) ;
#19932=DIRECTION ( 'NONE',  ( -1.000000000000000000, -1.208970125616048853E-17, 0.000000000000000000 ) ) ;
#19940=EDGE_CURVE ( 'NONE', #728, #16668, #10034, .T. ) ;
#19941=DIRECTION ( 'NONE',  ( 6.505213034913038160E-19, 3.903127820947822896E-18, 1.000000000000000000 ) ) ;
#19948=CARTESIAN_POINT ( 'NONE',  ( -22.15900668633755188, -29.33526866242114295, -2.800654218530433059 ) ) ;
#19950=ORIENTED_EDGE ( 'NONE', *, *, #7114, .F. ) ;
#19956=ORIENTED_EDGE ( 'NONE', *, *, #9336, .F. ) ;
#19963=AXIS2_PLACEMENT_3D ( 'NONE', #781, #7762, #14845 ) ;
#19970=CARTESIAN_POINT ( 'NONE',  ( 30.60042966911749573, 7.474202570535909196, -2.999999999999988898 ) ) ;
#19973=EDGE_CURVE ( 'NONE', #17133, #12599, #13573, .T. ) ;
#19981=ORIENTED_EDGE ( 'NONE', *, *, #19893, .T. ) ;
#19983=CIRCLE ( 'NONE', #18503, 0.9999999999999974465 ) ;
#19987=AXIS2_PLACEMENT_3D ( 'NONE', #11744, #15283, #18738 ) ;
#19990=EDGE_CURVE ( 'NONE', #17804, #20782, #10825, .T. ) ;
#19991=CARTESIAN_POINT ( 'NONE',  ( -31.21605069118063724, -8.646032897229371628, -2.999999999999971578 ) ) ;
#19997=AXIS2_PLACEMENT_3D ( 'NONE', #7311, #17732, #5822 ) ;
#20003=VERTEX_POINT ( 'NONE', #2136 ) ;
#20004=CYLINDRICAL_SURFACE ( 'NONE', #1047, 1.000000000000000888 ) ;
#20005=FACE_OUTER_BOUND ( 'NONE', #16971, .T. ) ;
#20006=ORIENTED_EDGE ( 'NONE', *, *, #16812, .F. ) ;
#20008=EDGE_LOOP ( 'NONE', ( #5668, #4232 ) ) ;
#20009=CYLINDRICAL_SURFACE ( 'NONE', #5705, 36.76383501243555685 ) ;
#20012=EDGE_CURVE ( 'NONE', #18491, #16319, #20085, .T. ) ;
#20016=DIRECTION ( 'NONE',  ( -1.000000000000000000, -1.208970125616046080E-17, 6.505213034913038160E-19 ) ) ;
#20020=ORIENTED_EDGE ( 'NONE', *, *, #12288, .T. ) ;
#20025=VECTOR ( 'NONE', #5075, 1000.000000000000000 ) ;
#20029=ADVANCED_FACE ( 'NONE', ( #10706 ), #2017, .T. ) ;
#20030=CARTESIAN_POINT ( 'NONE',  ( 21.05198877411829272, -30.13956425491240410, -2.800654218530457484 ) ) ;
#20031=CYLINDRICAL_SURFACE ( 'NONE', #21836, 28.00000000000001066 ) ;
#20032=CARTESIAN_POINT ( 'NONE',  ( 1.110223024625156540E-13, -5.551115123125782702E-14, -6.999999999999950262 ) ) ;
#20037=DIRECTION ( 'NONE',  ( -1.000000000000000000, -3.376276133282418451E-14, 0.000000000000000000 ) ) ;
#20040=CARTESIAN_POINT ( 'NONE',  ( -28.45046755804880689, 15.62726112422596714, -7.000000000000006217 ) ) ;
#20046=CARTESIAN_POINT ( 'NONE',  ( -32.83234229683724692, 11.85401191286869427, 3.000000000000002665 ) ) ;
#20048=EDGE_LOOP ( 'NONE', ( #12812, #5697, #22228, #7916, #7507, #16710 ) ) ;
#20053=VERTEX_POINT ( 'NONE', #7169 ) ;
#20057=CARTESIAN_POINT ( 'NONE',  ( 32.75570538720779012, -15.02862401740828702, -2.999999999999964473 ) ) ;
#20062=DIRECTION ( 'NONE',  ( -6.505213034913038160E-19, -3.903127820947822896E-18, -1.000000000000000000 ) ) ;
#20064=ORIENTED_EDGE ( 'NONE', *, *, #2621, .T. ) ;
#20072=CARTESIAN_POINT ( 'NONE',  ( -22.22891329980529562, 23.65408649739109137, 2.999999999999995559 ) ) ;
#20073=AXIS2_PLACEMENT_3D ( 'NONE', #14818, #2932, #16789 ) ;
#20076=EDGE_CURVE ( 'NONE', #18701, #8987, #21821, .T. ) ;
#20077=AXIS2_PLACEMENT_3D ( 'NONE', #3687, #17877, #7219 ) ;
#20083=LINE ( 'NONE', #8049, #17216 ) ;
#20085=CIRCLE ( 'NONE', #22289, 0.9999999999999974465 ) ;
#20089=DIRECTION ( 'NONE',  ( 6.505213034913038160E-19, 3.903127820947822896E-18, 1.000000000000000000 ) ) ;
#20097=EDGE_LOOP ( 'NONE', ( #21308, #18906, #22260, #15239 ) ) ;
#20103=EDGE_CURVE ( 'NONE', #19660, #21037, #17777, .T. ) ;
#20109=EDGE_LOOP ( 'NONE', ( #204, #14817, #22244, #21795, #20558, #835 ) ) ;
#20111=ORIENTED_EDGE ( 'NONE', *, *, #12534, .T. ) ;
#20119=FACE_OUTER_BOUND ( 'NONE', #6771, .T. ) ;
#20120=ORIENTED_EDGE ( 'NONE', *, *, #5252, .T. ) ;
#20123=ORIENTED_EDGE ( 'NONE', *, *, #15461, .T. ) ;
#20124=CARTESIAN_POINT ( 'NONE',  ( 36.75746821813311271, -0.6841746959068695233, -1.999999999999994893 ) ) ;
#20125=EDGE_CURVE ( 'NONE', #2949, #2277, #14833, .T. ) ;
#20127=CARTESIAN_POINT ( 'NONE',  ( -34.88850421923980605, 1.128083539116031542, 2.999999999999995559 ) ) ;
#20129=EDGE_CURVE ( 'NONE', #12073, #943, #21157, .T. ) ;
#20132=CARTESIAN_POINT ( 'NONE',  ( -12.00937115242649256, -34.74700806321106938, -2.800654218530485018 ) ) ;
#20133=ORIENTED_EDGE ( 'NONE', *, *, #21533, .F. ) ;
#20139=CYLINDRICAL_SURFACE ( 'NONE', #892, 31.50000000000000711 ) ;
#20146=EDGE_CURVE ( 'NONE', #12403, #15891, #14477, .T. ) ;
#20150=VERTEX_POINT ( 'NONE', #6361 ) ;
#20151=DIRECTION ( 'NONE',  ( -1.000000000000000000, -1.208970125616046080E-17, 6.505213034913038160E-19 ) ) ;
#20152=CARTESIAN_POINT ( 'NONE',  ( 4.171001175319571708, 35.79662727779881237, -6.999999999999950262 ) ) ;
#20156=DIRECTION ( 'NONE',  ( 1.000000000000000000, 0.000000000000000000, 0.000000000000000000 ) ) ;
#20157=DIRECTION ( 'NONE',  ( -6.505213034913038160E-19, -3.903127820947822896E-18, -1.000000000000000000 ) ) ;
#20159=AXIS2_PLACEMENT_3D ( 'NONE', #10905, #19513, #15826 ) ;
#20164=EDGE_LOOP ( 'NONE', ( #15048, #15232, #2088, #16957 ) ) ;
#20166=DIRECTION ( 'NONE',  ( 6.505213034913038160E-19, 3.903127820947822896E-18, 1.000000000000000000 ) ) ;
#20167=CYLINDRICAL_SURFACE ( 'NONE', #16192, 0.9999999999999974465 ) ;
#20169=CYLINDRICAL_SURFACE ( 'NONE', #18580, 31.50000000000000711 ) ;
#20170=DIRECTION ( 'NONE',  ( 1.000000000000000000, 0.000000000000000000, 0.000000000000000000 ) ) ;
#20171=CIRCLE ( 'NONE', #17235, 3.000000000000002665 ) ;
#20178=ADVANCED_FACE ( 'NONE', ( #6142 ), #6429, .T. ) ;
#20179=ORIENTED_EDGE ( 'NONE', *, *, #1066, .T. ) ;
#20181=DIRECTION ( 'NONE',  ( 6.505213034913038160E-19, 3.903127820947822896E-18, 1.000000000000000000 ) ) ;
#20182=LINE ( 'NONE', #16623, #4895 ) ;
#20183=EDGE_CURVE ( 'NONE', #17988, #10690, #4428, .T. ) ;
#20184=CIRCLE ( 'NONE', #17618, 1.000000000000000888 ) ;
#20187=B_SPLINE_CURVE_WITH_KNOTS ( 'NONE', 3,
 ( #5470, #1915, #21169, #3315 ),
 .UNSPECIFIED., .F., .F.,
 ( 4, 4 ),
 ( 0.001875451646903046523, 0.003761979286331322732 ),
 .UNSPECIFIED. ) ;
#20192=DIRECTION ( 'NONE',  ( 1.000000000000000000, 0.000000000000000000, 0.000000000000000000 ) ) ;
#20198=CARTESIAN_POINT ( 'NONE',  ( 34.09180625983512414, 10.01331137436145013, -2.999999999999984901 ) ) ;
#20207=FACE_OUTER_BOUND ( 'NONE', #21112, .T. ) ;
#20210=EDGE_CURVE ( 'NONE', #10262, #9329, #16673, .T. ) ;
#20214=UNCERTAINTY_MEASURE_WITH_UNIT (LENGTH_MEASURE( 1.000000000000000082E-05 ), #17560, 'distance_accuracy_value', 'NONE');
#20226=ADVANCED_FACE ( 'NONE', ( #6255 ), #20009, .T. ) ;
#20228=DIRECTION ( 'NONE',  ( 1.000000000000000000, 1.208970125616063182E-17, 0.000000000000000000 ) ) ;
#20235=EDGE_CURVE ( 'NONE', #15368, #19564, #591, .T. ) ;
#20236=DIRECTION ( 'NONE',  ( 1.000000000000000000, 1.208970125616063182E-17, 0.000000000000000000 ) ) ;
#20247=ORIENTED_EDGE ( 'NONE', *, *, #11764, .T. ) ;
#20249=CARTESIAN_POINT ( 'NONE',  ( -10.00000000000000888, 3.000000000000002665, 5.000000000000000888 ) ) ;
#20251=EDGE_CURVE ( 'NONE', #7580, #15404, #10223, .T. ) ;
#20254=CIRCLE ( 'NONE', #6707, 1.000000000000000888 ) ;
#20258=EDGE_CURVE ( 'NONE', #21090, #5871, #21723, .T. ) ;
#20260=EDGE_CURVE ( 'NONE', #14751, #15922, #1435, .T. ) ;
#20262=ADVANCED_FACE ( 'NONE', ( #16901 ), #8422, .T. ) ;
#20272=CARTESIAN_POINT ( 'NONE',  ( 32.40961249803553557, -2.422192751864171711, 2.999999999999995559 ) ) ;
#20273=CARTESIAN_POINT ( 'NONE',  ( 30.07487443287981677, -12.31876324338301920, -2.999999999999999112 ) ) ;
#20274=EDGE_CURVE ( 'NONE', #20847, #4626, #10242, .T. ) ;
#20276=B_SPLINE_CURVE_WITH_KNOTS ( 'NONE', 3,
 ( #15665, #14270, #12343, #8687 ),
 .UNSPECIFIED., .F., .F.,
 ( 4, 4 ),
 ( 0.001875451646903004022, 0.003761979286331056885 ),
 .UNSPECIFIED. ) ;
#20279=CARTESIAN_POINT ( 'NONE',  ( -14.74639653023204744, 28.96193690644924246, -7.000000000000006217 ) ) ;
#20280=VERTEX_POINT ( 'NONE', #8529 ) ;
#20282=DIRECTION ( 'NONE',  ( 1.000000000000000000, 0.000000000000000000, 0.000000000000000000 ) ) ;
#20283=CIRCLE ( 'NONE', #10378, 19.11328065563151668 ) ;
#20284=DIRECTION ( 'NONE',  ( -6.505213034913038160E-19, -3.903127820947822896E-18, -1.000000000000000000 ) ) ;
#20287=AXIS2_PLACEMENT_3D ( 'NONE', #11687, #18683, #2988 ) ;
#20288=CARTESIAN_POINT ( 'NONE',  ( 22.28024240313505899, 22.26748298433242468, -7.000000000000006217 ) ) ;
#20291=CARTESIAN_POINT ( 'NONE',  ( 35.16985127952418111, 10.70799354677351367, -2.800654218530464146 ) ) ;
#20298=AXIS2_PLACEMENT_3D ( 'NONE', #21934, #2791, #13293 ) ;
#20300=CARTESIAN_POINT ( 'NONE',  ( -34.10919265018073077, 11.98978967046168265, 2.932969818539067575 ) ) ;
#20302=EDGE_CURVE ( 'NONE', #3679, #5453, #16682, .T. ) ;
#20304=ORIENTED_EDGE ( 'NONE', *, *, #13669, .T. ) ;
#20308=CARTESIAN_POINT ( 'NONE',  ( -5.093313992686310243, -32.09841355226006243, 2.999999999999995559 ) ) ;
#20309=FACE_BOUND ( 'NONE', #18711, .T. ) ;
#20312=ORIENTED_EDGE ( 'NONE', *, *, #4150, .F. ) ;
#20313=DIRECTION ( 'NONE',  ( 6.505213034913038160E-19, 3.903127820947822896E-18, 1.000000000000000000 ) ) ;
#20314=FACE_OUTER_BOUND ( 'NONE', #10924, .T. ) ;
#20315=ORIENTED_EDGE ( 'NONE', *, *, #18741, .F. ) ;
#20316=CARTESIAN_POINT ( 'NONE',  ( 21.00948735876911755, 24.79619811426203668, 3.000000000000006217 ) ) ;
#20333=EDGE_LOOP ( 'NONE', ( #9521, #7266, #5863, #6112 ) ) ;
#20334=CIRCLE ( 'NONE', #14062, 0.9999999999999974465 ) ;
#20336=ORIENTED_EDGE ( 'NONE', *, *, #8361, .F. ) ;
#20338=ORIENTED_EDGE ( 'NONE', *, *, #5785, .T. ) ;
#20339=CARTESIAN_POINT ( 'NONE',  ( 27.19760187735889545, 24.73600648735091312, 2.800654218530485018 ) ) ;
#20345=VERTEX_POINT ( 'NONE', #12512 ) ;
#20350=ORIENTED_EDGE ( 'NONE', *, *, #12946, .F. ) ;
#20352=CIRCLE ( 'NONE', #22183, 19.11328065563150957 ) ;
#20354=DIRECTION ( 'NONE',  ( 6.505213034913038160E-19, 3.903127820947822896E-18, 1.000000000000000000 ) ) ;
#20357=LINE ( 'NONE', #15398, #20685 ) ;
#20359=AXIS2_PLACEMENT_3D ( 'NONE', #1336, #2838, #8329 ) ;
#20366=AXIS2_PLACEMENT_3D ( 'NONE', #4691, #12914, #6288 ) ;
#20367=DIRECTION ( 'NONE',  ( -6.505213034913038160E-19, -3.903127820947822896E-18, -1.000000000000000000 ) ) ;
#20369=CARTESIAN_POINT ( 'NONE',  ( -28.06260833510287966, 14.30873905802324053, 2.999999999999995559 ) ) ;
#20370=CARTESIAN_POINT ( 'NONE',  ( -17.99805307122279174, -21.44924440733175786, 3.000000000000023537 ) ) ;
#20372=CARTESIAN_POINT ( 'NONE',  ( -31.57187188083528184, -7.711478842616553919, 3.000000000000023537 ) ) ;
#20374=CARTESIAN_POINT ( 'NONE',  ( 33.51030287062395274, 15.12081897056660651, 2.800654218530485018 ) ) ;
#20375=DIRECTION ( 'NONE',  ( 1.000000000000000000, 0.000000000000000000, 0.000000000000000000 ) ) ;
#20377=CIRCLE ( 'NONE', #5000, 0.9999999999999956701 ) ;
#20384=EDGE_CURVE ( 'NONE', #1842, #20949, #6066, .T. ) ;
#20385=FACE_OUTER_BOUND ( 'NONE', #8642, .T. ) ;
#20387=ORIENTED_EDGE ( 'NONE', *, *, #10758, .T. ) ;
#20388=ADVANCED_FACE ( 'NONE', ( #3725 ), #9729, .T. ) ;
#20395=ADVANCED_FACE ( 'NONE', ( #5652 ), #8992, .T. ) ;
#20396=CARTESIAN_POINT ( 'NONE',  ( -14.74639653023206165, 28.96193690644924246, -2.999999999999968026 ) ) ;
#20397=CARTESIAN_POINT ( 'NONE',  ( 7.711478842616581453, -31.57187188083526763, -2.999999999999995559 ) ) ;
#20398=CARTESIAN_POINT ( 'NONE',  ( 1.110223024625156540E-13, -5.551115123125782702E-14, -6.999999999999950262 ) ) ;
#20400=CIRCLE ( 'NONE', #21493, 36.76383501243555685 ) ;
#20408=CIRCLE ( 'NONE', #21864, 1.000000000000000888 ) ;
#20409=VERTEX_POINT ( 'NONE', #14230 ) ;
#20410=DIRECTION ( 'NONE',  ( -6.505213034913038160E-19, -3.903127820947822896E-18, -1.000000000000000000 ) ) ;
#20411=DIRECTION ( 'NONE',  ( -1.000000000000000000, -1.208970125616077665E-17, 0.000000000000000000 ) ) ;
#20414=ORIENTED_EDGE ( 'NONE', *, *, #320, .F. ) ;
#20417=ORIENTED_EDGE ( 'NONE', *, *, #251, .F. ) ;
#20424=EDGE_CURVE ( 'NONE', #19747, #6187, #5326, .T. ) ;
#20427=EDGE_LOOP ( 'NONE', ( #18881, #16181, #7338, #20501 ) ) ;
#20429=CARTESIAN_POINT ( 'NONE',  ( -8.646032897229066094, 31.21605069118044185, 2.999999999999995559 ) ) ;
#20442=ORIENTED_EDGE ( 'NONE', *, *, #21685, .F. ) ;
#20447=DIRECTION ( 'NONE',  ( -1.000000000000000000, 2.033026488858229532E-14, 0.000000000000000000 ) ) ;
#20454=CARTESIAN_POINT ( 'NONE',  ( -21.41958700883256483, -27.56232195404059837, 2.999999999999995559 ) ) ;
#20457=ORIENTED_EDGE ( 'NONE', *, *, #16309, .F. ) ;
#20461=AXIS2_PLACEMENT_3D ( 'NONE', #12262, #19269, #17301 ) ;
#20462=DIRECTION ( 'NONE',  ( 6.505213034913038160E-19, 3.903127820947822896E-18, 1.000000000000000000 ) ) ;
#20466=CARTESIAN_POINT ( 'NONE',  ( -14.93538271375420479, -34.13396246814581758, -2.999999999999999112 ) ) ;
#20468=AXIS2_PLACEMENT_3D ( 'NONE', #17791, #2096, #14335 ) ;
#20469=EDGE_CURVE ( 'NONE', #15106, #12184, #16251, .T. ) ;
#20473=EDGE_CURVE ( 'NONE', #573, #2168, #21837, .T. ) ;
#20480=CARTESIAN_POINT ( 'NONE',  ( -14.74639653023204744, 28.96193690644924246, -7.000000000000006217 ) ) ;
#20481=CYLINDRICAL_SURFACE ( 'NONE', #10813, 31.50000000000001421 ) ;
#20483=DIRECTION ( 'NONE',  ( -1.000000000000000000, 0.000000000000000000, 0.000000000000000000 ) ) ;
#20487=ORIENTED_EDGE ( 'NONE', *, *, #103, .F. ) ;
#20491=DIRECTION ( 'NONE',  ( -6.505213034913038160E-19, -3.903127820947822896E-18, -1.000000000000000000 ) ) ;
#20501=ORIENTED_EDGE ( 'NONE', *, *, #18064, .F. ) ;
#20504=AXIS2_PLACEMENT_3D ( 'NONE', #2558, #16521, #19752 ) ;
#20506=CARTESIAN_POINT ( 'NONE',  ( -5.074925817841608122, 32.10132595304110481, 3.000000000000016431 ) ) ;
#20511=DIRECTION ( 'NONE',  ( 1.000000000000000000, 0.000000000000000000, 0.000000000000000000 ) ) ;
#20514=EDGE_CURVE ( 'NONE', #6211, #2785, #22191, .T. ) ;
#20515=DIRECTION ( 'NONE',  ( -1.000000000000000000, -1.208970125616048853E-17, 0.000000000000000000 ) ) ;
#20517=CARTESIAN_POINT ( 'NONE',  ( -32.20238537491806596, -4.080045426413075660, -6.999999999999964473 ) ) ;
#20519=CYLINDRICAL_SURFACE ( 'NONE', #17034, 0.9999999999999995559 ) ;
#20521=LINE ( 'NONE', #1496, #21907 ) ;
#20523=ORIENTED_EDGE ( 'NONE', *, *, #2948, .F. ) ;
#20524=ORIENTED_EDGE ( 'NONE', *, *, #561, .F. ) ;
#20529=FACE_OUTER_BOUND ( 'NONE', #20689, .T. ) ;
#20531=DIRECTION ( 'NONE',  ( -1.000000000000000000, -1.208970125616063644E-17, 0.000000000000000000 ) ) ;
#20536=CARTESIAN_POINT ( 'NONE',  ( -7.980461308159631173, 36.39375341857503798, -7.000000000000006217 ) ) ;
#20537=CARTESIAN_POINT ( 'NONE',  ( -4.936596639065177428, -31.11077005834450659, -2.999999999999964473 ) ) ;
#20538=ORIENTED_EDGE ( 'NONE', *, *, #21962, .F. ) ;
#20540=DIRECTION ( 'NONE',  ( 6.505213034913038160E-19, 3.903127820947822896E-18, 1.000000000000000000 ) ) ;
#20543=ORIENTED_EDGE ( 'NONE', *, *, #16482, .T. ) ;
#20546=DIRECTION ( 'NONE',  ( -6.505213034913038160E-19, -3.903127820947822896E-18, -1.000000000000000000 ) ) ;
#20549=ORIENTED_EDGE ( 'NONE', *, *, #19940, .F. ) ;
#20551=AXIS2_PLACEMENT_3D ( 'NONE', #22087, #20583, #10031 ) ;
#20553=DIRECTION ( 'NONE',  ( 6.505213034913038160E-19, 3.903127820947822896E-18, 1.000000000000000000 ) ) ;
#20556=ORIENTED_EDGE ( 'NONE', *, *, #21441, .T. ) ;
#20558=ORIENTED_EDGE ( 'NONE', *, *, #103, .T. ) ;
#20563=ORIENTED_EDGE ( 'NONE', *, *, #7537, .T. ) ;
#20564=DIRECTION ( 'NONE',  ( 6.505213034913038160E-19, 3.903127820947822896E-18, 1.000000000000000000 ) ) ;
#20565=VERTEX_POINT ( 'NONE', #22386 ) ;
#20566=CARTESIAN_POINT ( 'NONE',  ( 2.775557561562891351E-14, -2.775557561562891351E-14, 2.999999999999995559 ) ) ;
#20569=FACE_OUTER_BOUND ( 'NONE', #14856, .T. ) ;
#20574=DIRECTION ( 'NONE',  ( -1.000000000000000000, -1.208970125616044077E-17, 0.000000000000000000 ) ) ;
#20577=EDGE_CURVE ( 'NONE', #11397, #13545, #14846, .T. ) ;
#20578=ORIENTED_EDGE ( 'NONE', *, *, #17983, .F. ) ;
#20579=ORIENTED_EDGE ( 'NONE', *, *, #16549, .F. ) ;
#20581=DIRECTION ( 'NONE',  ( 6.505213034913038160E-19, 3.903127820947822896E-18, 1.000000000000000000 ) ) ;
#20582=CARTESIAN_POINT ( 'NONE',  ( 2.220446049250313081E-13, -2.498001805406602216E-13, -6.859353255829918616 ) ) ;
#20583=DIRECTION ( 'NONE',  ( -6.505213034913038160E-19, -3.903127820947822896E-18, -1.000000000000000000 ) ) ;
#20586=ORIENTED_EDGE ( 'NONE', *, *, #4093, .T. ) ;
#20591=EDGE_CURVE ( 'NONE', #8449, #5417, #14497, .T. ) ;
#20595=CARTESIAN_POINT ( 'NONE',  ( 5.551115123125782702E-14, -1.387778780781445676E-13, -5.749999999999949374 ) ) ;
#20597=DIRECTION ( 'NONE',  ( 6.505213034913038160E-19, 3.903127820947822896E-18, 1.000000000000000000 ) ) ;
#20600=CIRCLE ( 'NONE', #22447, 19.11328065563150957 ) ;
#20603=CARTESIAN_POINT ( 'NONE',  ( -14.76298474240507552, -28.95348479018572263, 3.000000000000023537 ) ) ;
#20605=EDGE_CURVE ( 'NONE', #13471, #8183, #20377, .T. ) ;
#20617=CIRCLE ( 'NONE', #13644, 19.11328065563152023 ) ;
#20619=CARTESIAN_POINT ( 'NONE',  ( 6.742883674876798850, 34.24928931925766307, 2.999999999999999112 ) ) ;
#20620=CIRCLE ( 'NONE', #14750, 1.000000000000001776 ) ;
#20622=DIRECTION ( 'NONE',  ( 1.000000000000000000, 0.000000000000000000, 0.000000000000000000 ) ) ;
#20628=CIRCLE ( 'NONE', #875, 19.11328065563150957 ) ;
#20631=ADVANCED_FACE ( 'NONE', ( #16879 ), #10214, .F. ) ;
#20634=CARTESIAN_POINT ( 'NONE',  ( 31.57187188083540619, 7.711478842616415363, -7.000000000000006217 ) ) ;
#20635=CARTESIAN_POINT ( 'NONE',  ( 36.75746821813321930, -0.6841746959067585010, -2.800654218530457484 ) ) ;
#20639=EDGE_LOOP ( 'NONE', ( #3250, #15290, #22617, #10224 ) ) ;
#20642=ORIENTED_EDGE ( 'NONE', *, *, #6978, .T. ) ;
#20644=CYLINDRICAL_SURFACE ( 'NONE', #19617, 19.11328065563150957 ) ;
#20648=DIRECTION ( 'NONE',  ( -1.000000000000000000, -1.208970125616060717E-17, 0.000000000000000000 ) ) ;
#20657=CARTESIAN_POINT ( 'NONE',  ( 1.128083539116558898, 34.88850421923955736, 3.000000000000002665 ) ) ;
#20661=ORIENTED_EDGE ( 'NONE', *, *, #6109, .F. ) ;
#20662=VERTEX_POINT ( 'NONE', #1407 ) ;
#20664=ORIENTED_EDGE ( 'NONE', *, *, #9439, .F. ) ;
#20669=ORIENTED_EDGE ( 'NONE', *, *, #19789, .T. ) ;
#20674=ORIENTED_EDGE ( 'NONE', *, *, #9181, .F. ) ;
#20680=ADVANCED_FACE ( 'NONE', ( #8281 ), #16339, .T. ) ;
#20681=DIRECTION ( 'NONE',  ( 1.000000000000000000, 0.000000000000000000, 0.000000000000000000 ) ) ;
#20685=VECTOR ( 'NONE', #8315, 1000.000000000000000 ) ;
#20688=DIRECTION ( 'NONE',  ( -6.505213034913038160E-19, -3.903127820947822896E-18, -1.000000000000000000 ) ) ;
#20689=EDGE_LOOP ( 'NONE', ( #16364, #12761, #11278, #12374 ) ) ;
#20693=AXIS2_PLACEMENT_3D ( 'NONE', #12601, #18339, #587 ) ;
#20694=ORIENTED_EDGE ( 'NONE', *, *, #16216, .T. ) ;
#20695=DIRECTION ( 'NONE',  ( 6.505213034913038160E-19, 3.903127820947822896E-18, 1.000000000000000000 ) ) ;
#20697=AXIS2_PLACEMENT_3D ( 'NONE', #5738, #9519, #2187 ) ;
#20699=AXIS2_PLACEMENT_3D ( 'NONE', #2328, #12621, #4168 ) ;
#20702=EDGE_CURVE ( 'NONE', #9840, #22614, #10100, .T. ) ;
#20704=DIRECTION ( 'NONE',  ( 6.505213034913038160E-19, 3.903127820947822896E-18, 1.000000000000000000 ) ) ;
#20706=DIRECTION ( 'NONE',  ( 6.505213034913038160E-19, 3.903127820947822896E-18, 1.000000000000000000 ) ) ;
#20709=VERTEX_POINT ( 'NONE', #1748 ) ;
#20710=CYLINDRICAL_SURFACE ( 'NONE', #7585, 1.000000000000000888 ) ;
#20713=AXIS2_PLACEMENT_3D ( 'NONE', #11372, #9546, #13072 ) ;
#20715=CARTESIAN_POINT ( 'NONE',  ( -24.03323817228460157, 20.36304159388333090, -2.999999999999988898 ) ) ;
#20716=AXIS2_PLACEMENT_3D ( 'NONE', #21850, #11058, #4544 ) ;
#20721=AXIS2_PLACEMENT_3D ( 'NONE', #20273, #18206, #11208 ) ;
#20722=B_SPLINE_CURVE_WITH_KNOTS ( 'NONE', 3,
 ( #12716, #11118, #21668, #19738 ),
 .UNSPECIFIED., .F., .F.,
 ( 4, 4 ),
 ( 0.001893031756885608539, 0.003808480026563944992 ),
 .UNSPECIFIED. ) ;
#20723=ORIENTED_EDGE ( 'NONE', *, *, #7070, .T. ) ;
#20730=ORIENTED_EDGE ( 'NONE', *, *, #6475, .F. ) ;
#20737=AXIS2_PLACEMENT_3D ( 'NONE', #6263, #13223, #11066 ) ;
#20742=CARTESIAN_POINT ( 'NONE',  ( 6.953913411055066440, 34.84300730320191519, 3.000000000000042188 ) ) ;
#20748=EDGE_CURVE ( 'NONE', #8849, #22077, #5404, .T. ) ;
#20749=ORIENTED_EDGE ( 'NONE', *, *, #15734, .T. ) ;
#20756=CARTESIAN_POINT ( 'NONE',  ( -22.26748298433250994, 22.28024240313478188, -6.999999999999957367 ) ) ;
#20758=EDGE_LOOP ( 'NONE', ( #12762, #17779, #3933, #3978, #1073, #3843 ) ) ;
#20759=CARTESIAN_POINT ( 'NONE',  ( -21.00948735876860596, -24.79619811426211839, 2.999999999999995559 ) ) ;
#20761=EDGE_LOOP ( 'NONE', ( #6056, #7899, #21902, #6624 ) ) ;
#20764=DIRECTION ( 'NONE',  ( -1.000000000000000000, 0.000000000000000000, 0.000000000000000000 ) ) ;
#20765=DIRECTION ( 'NONE',  ( 1.000000000000000000, 1.208970125616067188E-17, 0.000000000000000000 ) ) ;
#20768=EDGE_CURVE ( 'NONE', #8398, #573, #13392, .T. ) ;
#20772=ORIENTED_EDGE ( 'NONE', *, *, #13320, .F. ) ;
#20773=FACE_OUTER_BOUND ( 'NONE', #9512, .T. ) ;
#20774=VECTOR ( 'NONE', #14071, 1000.000000000000000 ) ;
#20776=FACE_OUTER_BOUND ( 'NONE', #19001, .T. ) ;
#20782=VERTEX_POINT ( 'NONE', #7014 ) ;
#20784=ORIENTED_EDGE ( 'NONE', *, *, #1051, .F. ) ;
#20785=ORIENTED_EDGE ( 'NONE', *, *, #5445, .F. ) ;
#20788=DIRECTION ( 'NONE',  ( -1.000000000000000000, -1.208970125616060101E-17, 6.505213034913038160E-19 ) ) ;
#20792=CARTESIAN_POINT ( 'NONE',  ( 29.74882400976413876, 20.54749497201894570, 2.932969818539052476 ) ) ;
#20803=DIRECTION ( 'NONE',  ( -6.505213034913038160E-19, -3.903127820947822896E-18, -1.000000000000000000 ) ) ;
#20804=AXIS2_PLACEMENT_3D ( 'NONE', #13915, #19332, #1800 ) ;
#20809=CARTESIAN_POINT ( 'NONE',  ( -0.6841746959067307454, -36.75746821813308429, 2.800654218530485018 ) ) ;
#20811=ORIENTED_EDGE ( 'NONE', *, *, #6400, .F. ) ;
#20814=ORIENTED_EDGE ( 'NONE', *, *, #218, .T. ) ;
#20815=EDGE_CURVE ( 'NONE', #14096, #5340, #6091, .T. ) ;
#20820=CARTESIAN_POINT ( 'NONE',  ( -11.85401191286884703, -32.83234229683740324, -2.999999999999971578 ) ) ;
#20824=EDGE_CURVE ( 'NONE', #1508, #17625, #7178, .T. ) ;
#20826=ORIENTED_EDGE ( 'NONE', *, *, #11189, .F. ) ;
#20827=DIRECTION ( 'NONE',  ( -6.505213034913038160E-19, -3.903127820947822896E-18, -1.000000000000000000 ) ) ;
#20829=TOROIDAL_SURFACE ( 'NONE', #9845, 34.90673715956759082, 8.750000000000000000 ) ;
#20830=DIRECTION ( 'NONE',  ( 6.505213034913038160E-19, 3.903127820947822896E-18, 1.000000000000000000 ) ) ;
#20838=CARTESIAN_POINT ( 'NONE',  ( -32.40961249803532240, 2.422192751863644133, -6.999999999999950262 ) ) ;
#20840=CARTESIAN_POINT ( 'NONE',  ( -30.07487443287959650, 12.31876324338271367, -2.999999999999999112 ) ) ;
#20841=DIRECTION ( 'NONE',  ( -1.000000000000000000, -1.788446540656407544E-15, 0.000000000000000000 ) ) ;
#20844=ADVANCED_FACE ( 'NONE', ( #3472 ), #10545, .F. ) ;
#20847=VERTEX_POINT ( 'NONE', #3918 ) ;
#20851=ORIENTED_EDGE ( 'NONE', *, *, #3649, .T. ) ;
#20853=CARTESIAN_POINT ( 'NONE',  ( 13.83143812983109200, -29.36548507648034700, 3.000000000000023537 ) ) ;
#20859=CARTESIAN_POINT ( 'NONE',  ( 1.128083539116392364, 34.88850421923958578, -2.999999999999981792 ) ) ;
#20861=ORIENTED_EDGE ( 'NONE', *, *, #17490, .T. ) ;
#20862=CARTESIAN_POINT ( 'NONE',  ( 27.57461708434214032, -4.862148974673824675, -2.999999999999971578 ) ) ;
#20867=CIRCLE ( 'NONE', #16829, 1.000000000000000888 ) ;
#20870=DIRECTION ( 'NONE',  ( 6.505213034913038160E-19, 3.903127820947822896E-18, 1.000000000000000000 ) ) ;
#20874=CARTESIAN_POINT ( 'NONE',  ( -28.07080038625074536, -14.29266125237910146, 2.999999999999995559 ) ) ;
#20878=ORIENTED_EDGE ( 'NONE', *, *, #8470, .F. ) ;
#20900=ORIENTED_EDGE ( 'NONE', *, *, #12534, .F. ) ;
#20902=DIRECTION ( 'NONE',  ( 6.505213034913038160E-19, 3.903127820947822896E-18, 1.000000000000000000 ) ) ;
#20906=ORIENTED_EDGE ( 'NONE', *, *, #519, .F. ) ;
#20907=CARTESIAN_POINT ( 'NONE',  ( 32.83234229683740324, -11.85401191286897316, 2.999999999999995559 ) ) ;
#20908=DIRECTION ( 'NONE',  ( -6.505213034913038160E-19, -3.903127820947822896E-18, -1.000000000000000000 ) ) ;
#20913=ORIENTED_EDGE ( 'NONE', *, *, #13426, .F. ) ;
#20914=CARTESIAN_POINT ( 'NONE',  ( 1.110223024625156540E-13, -5.551115123125782702E-14, -6.999999999999950262 ) ) ;
#20920=CARTESIAN_POINT ( 'NONE',  ( 2.775557561562891351E-14, -2.775557561562891351E-14, 2.999999999999999112 ) ) ;
#20921=DIRECTION ( 'NONE',  ( -6.505213034913038160E-19, -3.903127820947822896E-18, -1.000000000000000000 ) ) ;
#20922=CARTESIAN_POINT ( 'NONE',  ( 29.33526866242106124, -22.15900668633785742, 2.800654218530492123 ) ) ;
#20926=EDGE_CURVE ( 'NONE', #8398, #19833, #16503, .T. ) ;
#20927=ORIENTED_EDGE ( 'NONE', *, *, #12226, .T. ) ;
#20932=DIRECTION ( 'NONE',  ( 6.505213034913038160E-19, 3.903127820947822896E-18, 1.000000000000000000 ) ) ;
#20934=ADVANCED_FACE ( 'NONE', ( #16271 ), #6081, .T. ) ;
#20936=EDGE_LOOP ( 'NONE', ( #11160, #22121, #9324, #13143 ) ) ;
#20945=CARTESIAN_POINT ( 'NONE',  ( 2.775557561562891351E-14, -2.775557561562891351E-14, 2.999999999999999112 ) ) ;
#20948=ORIENTED_EDGE ( 'NONE', *, *, #163, .F. ) ;
#20949=VERTEX_POINT ( 'NONE', #9176 ) ;
#20951=ORIENTED_EDGE ( 'NONE', *, *, #10822, .T. ) ;
#20952=CARTESIAN_POINT ( 'NONE',  ( -14.29266125237879592, 28.07080038625078799, -7.000000000000006217 ) ) ;
#20956=ORIENTED_EDGE ( 'NONE', *, *, #16173, .F. ) ;
#20958=CARTESIAN_POINT ( 'NONE',  ( 2.775557561562891351E-14, 2.775557561562891351E-14, 5.750000000000001776 ) ) ;
#20959=CYLINDRICAL_SURFACE ( 'NONE', #19855, 0.9999999999999991118 ) ;
#20960=DIRECTION ( 'NONE',  ( -1.000000000000000000, 0.000000000000000000, 0.000000000000000000 ) ) ;
#20965=DIRECTION ( 'NONE',  ( 6.505213034913038160E-19, 3.903127820947822896E-18, 1.000000000000000000 ) ) ;
#20968=CARTESIAN_POINT ( 'NONE',  ( -35.16985127952374057, -10.70799354677395776, -2.800654218530457484 ) ) ;
#20969=CARTESIAN_POINT ( 'NONE',  ( 3.608224830031758756E-13, -2.775557561562891351E-14, -4.999999999999997335 ) ) ;
#20970=EDGE_LOOP ( 'NONE', ( #7891, #14360, #5997, #4391 ) ) ;
#20971=CARTESIAN_POINT ( 'NONE',  ( -26.79308242454895961, -16.56444186175090749, 2.999999999999995559 ) ) ;
#20979=LINE ( 'NONE', #21201, #20774 ) ;
#20980=LINE ( 'NONE', #20756, #18630 ) ;
#20983=AXIS2_PLACEMENT_3D ( 'NONE', #2459, #739, #7720 ) ;
#20988=EDGE_CURVE ( 'NONE', #3268, #15217, #22287, .T. ) ;
#20991=EDGE_CURVE ( 'NONE', #4363, #10740, #6108, .T. ) ;
#20992=DIRECTION ( 'NONE',  ( -1.000000000000000000, 0.000000000000000000, 0.000000000000000000 ) ) ;
#20997=ORIENTED_EDGE ( 'NONE', *, *, #14947, .T. ) ;
#20999=EDGE_CURVE ( 'NONE', #22470, #12493, #4041, .T. ) ;
#21000=DIRECTION ( 'NONE',  ( 6.505213034913038160E-19, 3.903127820947822896E-18, 1.000000000000000000 ) ) ;
#21003=AXIS2_PLACEMENT_3D ( 'NONE', #7736, #15978, #17701 ) ;
#21011=CYLINDRICAL_SURFACE ( 'NONE', #6319, 19.11328065563150957 ) ;
#21013=EDGE_CURVE ( 'NONE', #11834, #5053, #2300, .T. ) ;
#21014=CIRCLE ( 'NONE', #12219, 31.50000000000001421 ) ;
#21016=EDGE_LOOP ( 'NONE', ( #2799, #9215, #7557, #10241, #2110, #399 ) ) ;
#21019=VERTEX_POINT ( 'NONE', #7571 ) ;
#21020=FACE_OUTER_BOUND ( 'NONE', #10958, .T. ) ;
#21023=DIRECTION ( 'NONE',  ( 6.505213034913038160E-19, 3.903127820947822896E-18, 1.000000000000000000 ) ) ;
#21025=DIRECTION ( 'NONE',  ( -1.000000000000000000, -1.208970125616060101E-17, 6.505213034913038160E-19 ) ) ;
#21026=CARTESIAN_POINT ( 'NONE',  ( 4.718447854656915297E-13, -22.00000000000021316, -2.999999999999971578 ) ) ;
#21027=DIRECTION ( 'NONE',  ( -6.505213034913038160E-19, -3.903127820947822896E-18, -1.000000000000000000 ) ) ;
#21034=AXIS2_PLACEMENT_3D ( 'NONE', #20272, #8123, #18546 ) ;
#21035=ORIENTED_EDGE ( 'NONE', *, *, #1103, .F. ) ;
#21037=VERTEX_POINT ( 'NONE', #8030 ) ;
#21038=FACE_OUTER_BOUND ( 'NONE', #6834, .T. ) ;
#21039=EDGE_CURVE ( 'NONE', #16276, #3830, #16715, .T. ) ;
#21041=FACE_OUTER_BOUND ( 'NONE', #4459, .T. ) ;
#21043=VERTEX_POINT ( 'NONE', #6536 ) ;
#21045=CARTESIAN_POINT ( 'NONE',  ( 28.06260833510307151, -14.30873905802340573, -2.999999999999971578 ) ) ;
#21050=ADVANCED_FACE ( 'NONE', ( #4713 ), #9859, .F. ) ;
#21057=EDGE_CURVE ( 'NONE', #9968, #20345, #17812, .T. ) ;
#21060=EDGE_LOOP ( 'NONE', ( #5674, #1236, #7305, #20579 ) ) ;
#21061=EDGE_LOOP ( 'NONE', ( #20956, #21670, #7410, #21526 ) ) ;
#21064=DIRECTION ( 'NONE',  ( -6.505213034913038160E-19, -3.903127820947822896E-18, -1.000000000000000000 ) ) ;
#21069=VECTOR ( 'NONE', #17005, 1000.000000000000000 ) ;
#21076=LINE ( 'NONE', #209, #5356 ) ;
#21080=DIRECTION ( 'NONE',  ( 6.505213034913038160E-19, 3.903127820947822896E-18, 1.000000000000000000 ) ) ;
#21086=ORIENTED_EDGE ( 'NONE', *, *, #11406, .F. ) ;
#21090=VERTEX_POINT ( 'NONE', #20291 ) ;
#21092=EDGE_CURVE ( 'NONE', #5279, #2407, #9413, .T. ) ;
#21093=CARTESIAN_POINT ( 'NONE',  ( -13.06969024216335740, -19.15111107797470780, -2.999999999999995559 ) ) ;
#21098=DIRECTION ( 'NONE',  ( 6.505213034913038160E-19, 3.903127820947822896E-18, 1.000000000000000000 ) ) ;
#21099=EDGE_LOOP ( 'NONE', ( #2275, #15999, #17231, #9366 ) ) ;
#21102=CYLINDRICAL_SURFACE ( 'NONE', #18492, 22.00000000000000711 ) ;
#21105=DIRECTION ( 'NONE',  ( -1.000000000000000000, 0.000000000000000000, 0.000000000000000000 ) ) ;
#21107=VECTOR ( 'NONE', #583, 1000.000000000000000 ) ;
#21109=DIRECTION ( 'NONE',  ( -1.000000000000000000, -1.208970125616083212E-17, 0.000000000000000000 ) ) ;
#21112=EDGE_LOOP ( 'NONE', ( #19459, #16754, #15410, #4154 ) ) ;
#21113=EDGE_CURVE ( 'NONE', #13475, #19379, #1344, .T. ) ;
#21117=ORIENTED_EDGE ( 'NONE', *, *, #21966, .F. ) ;
#21122=CARTESIAN_POINT ( 'NONE',  ( 4.171001175319766219, 35.79662727779869869, 3.000000000000009770 ) ) ;
#21124=ADVANCED_FACE ( 'NONE', ( #17737 ), #17397, .T. ) ;
#21125=ORIENTED_EDGE ( 'NONE', *, *, #21309, .T. ) ;
#21128=ORIENTED_EDGE ( 'NONE', *, *, #10191, .F. ) ;
#21131=VERTEX_POINT ( 'NONE', #16014 ) ;
#21133=EDGE_LOOP ( 'NONE', ( #5211, #1087, #5131, #21490 ) ) ;
#21139=AXIS2_PLACEMENT_3D ( 'NONE', #7226, #14194, #21318 ) ;
#21147=ORIENTED_EDGE ( 'NONE', *, *, #18719, .F. ) ;
#21150=AXIS2_PLACEMENT_3D ( 'NONE', #15435, #11780, #20960 ) ;
#21156=ORIENTED_EDGE ( 'NONE', *, *, #13711, .T. ) ;
#21157=LINE ( 'NONE', #18387, #7903 ) ;
#21164=AXIS2_PLACEMENT_3D ( 'NONE', #2276, #9262, #9603 ) ;
#21165=DIRECTION ( 'NONE',  ( -6.505213034913038160E-19, -3.903127820947822896E-18, -1.000000000000000000 ) ) ;
#21167=ADVANCED_FACE ( 'NONE', ( #7199 ), #14168, .T. ) ;
#21168=DIRECTION ( 'NONE',  ( -6.505213034913038160E-19, -3.903127820947822896E-18, -1.000000000000000000 ) ) ;
#21169=CARTESIAN_POINT ( 'NONE',  ( -31.47514467962681550, 17.79500259159609499, 2.932460736555816627 ) ) ;
#21179=CARTESIAN_POINT ( 'NONE',  ( 1.110223024625156540E-13, -24.99999999999999289, 3.000000000000023537 ) ) ;
#21180=LINE ( 'NONE', #5481, #11192 ) ;
#21181=DIRECTION ( 'NONE',  ( -1.000000000000000000, 8.702939542935596068E-14, 0.000000000000000000 ) ) ;
#21190=ADVANCED_FACE ( 'NONE', ( #17280 ), #16351, .T. ) ;
#21192=DIRECTION ( 'NONE',  ( -1.000000000000000000, 1.234337511092497482E-14, 0.000000000000000000 ) ) ;
#21195=ORIENTED_EDGE ( 'NONE', *, *, #3394, .T. ) ;
#21200=DIRECTION ( 'NONE',  ( -6.505213034913038160E-19, -3.903127820947822896E-18, -1.000000000000000000 ) ) ;
#21201=CARTESIAN_POINT ( 'NONE',  ( -11.35354668330680639, -30.33632613426187774, -7.000000000000006217 ) ) ;
#21205=CARTESIAN_POINT ( 'NONE',  ( 2.220446049250313081E-13, -2.498001805406602216E-13, -6.859353255829918616 ) ) ;
#21208=EDGE_CURVE ( 'NONE', #6233, #7580, #5267, .T. ) ;
#21209=DIRECTION ( 'NONE',  ( -1.000000000000000000, -1.208970125616063644E-17, 0.000000000000000000 ) ) ;
#21226=ORIENTED_EDGE ( 'NONE', *, *, #19224, .F. ) ;
#21228=ORIENTED_EDGE ( 'NONE', *, *, #3453, .T. ) ;
#21230=CARTESIAN_POINT ( 'NONE',  ( -31.57187188083515750, -7.711478842616581453, -7.000000000000006217 ) ) ;
#21234=CARTESIAN_POINT ( 'NONE',  ( -31.41173278719228179, -17.66631876130928092, 2.999999999999999112 ) ) ;
#21235=ORIENTED_EDGE ( 'NONE', *, *, #6235, .F. ) ;
#21236=CARTESIAN_POINT ( 'NONE',  ( -35.33352588067108258, -7.094908322883481055, 2.999999999999999112 ) ) ;
#21237=DIRECTION ( 'NONE',  ( 1.000000000000000000, 0.000000000000000000, 0.000000000000000000 ) ) ;
#21239=EDGE_CURVE ( 'NONE', #20662, #17550, #19367, .T. ) ;
#21240=DIRECTION ( 'NONE',  ( 6.505213034913038160E-19, 3.903127820947822896E-18, 1.000000000000000000 ) ) ;
#21242=CARTESIAN_POINT ( 'NONE',  ( 34.65667543218833657, 4.170748987303380062, 2.999999999999999112 ) ) ;
#21244=PLANE ( 'NONE',  #1793 ) ;
#21251=DIRECTION ( 'NONE',  ( -6.505213034913038160E-19, -3.903127820947822896E-18, -1.000000000000000000 ) ) ;
#21254=CARTESIAN_POINT ( 'NONE',  ( 16.99647590252670426, 30.48934413892764894, -2.999999999999971578 ) ) ;
#21257=EDGE_CURVE ( 'NONE', #6602, #11475, #7961, .T. ) ;
#21258=ORIENTED_EDGE ( 'NONE', *, *, #21359, .T. ) ;
#21261=ORIENTED_EDGE ( 'NONE', *, *, #19323, .T. ) ;
#21262=DIRECTION ( 'NONE',  ( -6.505213034913038160E-19, -3.903127820947822896E-18, -1.000000000000000000 ) ) ;
#21264=CARTESIAN_POINT ( 'NONE',  ( -14.85562396683486952, 32.28023859650867422, -3.000000000000005773 ) ) ;
#21270=CARTESIAN_POINT ( 'NONE',  ( 31.67162468656012209, 14.67611967928900185, -2.999999999999971578 ) ) ;
#21273=DIRECTION ( 'NONE',  ( 6.505213034913038160E-19, 3.903127820947822896E-18, 1.000000000000000000 ) ) ;
#21278=AXIS2_PLACEMENT_3D ( 'NONE', #12149, #3458, #22370 ) ;
#21282=ORIENTED_EDGE ( 'NONE', *, *, #19432, .T. ) ;
#21285=ORIENTED_EDGE ( 'NONE', *, *, #1103, .T. ) ;
#21288=EDGE_CURVE ( 'NONE', #20345, #22114, #9150, .T. ) ;
#21291=CARTESIAN_POINT ( 'NONE',  ( 23.65408649739145375, 22.22891329980533470, 3.000000000000016431 ) ) ;
#21295=CARTESIAN_POINT ( 'NONE',  ( 31.92986134326236680, -18.22261011550291343, -2.800654218530485018 ) ) ;
#21298=DIRECTION ( 'NONE',  ( -6.505213034913038160E-19, -3.903127820947822896E-18, -1.000000000000000000 ) ) ;
#21302=ORIENTED_EDGE ( 'NONE', *, *, #6032, .T. ) ;
#21308=ORIENTED_EDGE ( 'NONE', *, *, #17441, .T. ) ;
#21309=EDGE_CURVE ( 'NONE', #4860, #9803, #19675, .T. ) ;
#21311=CARTESIAN_POINT ( 'NONE',  ( 2.220446049250313081E-13, -2.498001805406602216E-13, -6.859353255829918616 ) ) ;
#21312=DIRECTION ( 'NONE',  ( 6.505213034913038160E-19, 3.903127820947822896E-18, 1.000000000000000000 ) ) ;
#21313=ORIENTED_EDGE ( 'NONE', *, *, #21627, .F. ) ;
#21318=DIRECTION ( 'NONE',  ( -1.000000000000000000, 0.000000000000000000, 0.000000000000000000 ) ) ;
#21320=AXIS2_PLACEMENT_3D ( 'NONE', #2753, #4705, #11219 ) ;
#21322=ORIENTED_EDGE ( 'NONE', *, *, #17214, .F. ) ;
#21327=ORIENTED_EDGE ( 'NONE', *, *, #16160, .T. ) ;
#21329=CARTESIAN_POINT ( 'NONE',  ( -17.99805307122284859, -21.44924440733170101, -4.999999999999984013 ) ) ;
#21331=ADVANCED_FACE ( 'NONE', ( #5709 ), #10977, .T. ) ;
#21333=AXIS2_PLACEMENT_3D ( 'NONE', #15297, #18646, #2951 ) ;
#21334=EDGE_LOOP ( 'NONE', ( #4489, #8502, #9135, #21226 ) ) ;
#21338=EDGE_LOOP ( 'NONE', ( #9629, #9383, #1533, #6807 ) ) ;
#21342=ORIENTED_EDGE ( 'NONE', *, *, #9050, .F. ) ;
#21348=CARTESIAN_POINT ( 'NONE',  ( -14.93538271375398274, -34.13396246814581758, 3.000000000000023537 ) ) ;
#21349=ORIENTED_EDGE ( 'NONE', *, *, #2200, .F. ) ;
#21354=B_SPLINE_CURVE_WITH_KNOTS ( 'NONE', 3,
 ( #14851, #18197, #5711, #7765 ),
 .UNSPECIFIED., .F., .F.,
 ( 4, 4 ),
 ( 9.545285769333515678E-07, 0.001900595205834842375 ),
 .UNSPECIFIED. ) ;
#21355=LINE ( 'NONE', #19648, #18403 ) ;
#21358=AXIS2_PLACEMENT_3D ( 'NONE', #16997, #1304, #15151 ) ;
#21359=EDGE_CURVE ( 'NONE', #10824, #15170, #21501, .T. ) ;
#21361=CARTESIAN_POINT ( 'NONE',  ( 26.64693883069180913, 24.43377932785589479, -2.933296326616372074 ) ) ;
#21362=AXIS2_PLACEMENT_3D ( 'NONE', #12939, #14879, #6420 ) ;
#21366=ADVANCED_FACE ( 'NONE', ( #19107 ), #12516, .T. ) ;
#21368=EDGE_CURVE ( 'NONE', #14834, #13710, #7209, .T. ) ;
#21370=ORIENTED_EDGE ( 'NONE', *, *, #2501, .F. ) ;
#21371=VERTEX_POINT ( 'NONE', #15532 ) ;
#21375=AXIS2_PLACEMENT_3D ( 'NONE', #1019, #3201, #11561 ) ;
#21378=VERTEX_POINT ( 'NONE', #3954 ) ;
#21379=CARTESIAN_POINT ( 'NONE',  ( 31.41173278719261575, 17.66631876130911394, -6.999999999999950262 ) ) ;
#21382=ORIENTED_EDGE ( 'NONE', *, *, #12806, .T. ) ;
#21394=ADVANCED_FACE ( 'NONE', ( #22556 ), #20710, .F. ) ;
#21395=ORIENTED_EDGE ( 'NONE', *, *, #1493, .F. ) ;
#21396=DIRECTION ( 'NONE',  ( -1.000000000000000000, -1.208970125616063644E-17, 0.000000000000000000 ) ) ;
#21397=EDGE_CURVE ( 'NONE', #16345, #7411, #14290, .T. ) ;
#21399=CARTESIAN_POINT ( 'NONE',  ( 2.775557561562891351E-14, -2.775557561562891351E-14, 2.999999999999999112 ) ) ;
#21407=ORIENTED_EDGE ( 'NONE', *, *, #13116, .F. ) ;
#21410=DIRECTION ( 'NONE',  ( -1.000000000000000000, -1.208970125616081209E-17, 0.000000000000000000 ) ) ;
#21411=CARTESIAN_POINT ( 'NONE',  ( -22.97438720605751783, 22.98755168577401520, 3.000000000000023537 ) ) ;
#21412=ORIENTED_EDGE ( 'NONE', *, *, #9545, .T. ) ;
#21418=EDGE_LOOP ( 'NONE', ( #12948, #247, #21679, #3422, #8748, #13648 ) ) ;
#21422=ORIENTED_EDGE ( 'NONE', *, *, #9598, .T. ) ;
#21424=AXIS2_PLACEMENT_3D ( 'NONE', #10127, #20354, #22185 ) ;
#21426=CARTESIAN_POINT ( 'NONE',  ( 2.775557561562891351E-14, 2.775557561562891351E-14, 5.750000000000001776 ) ) ;
#21430=ORIENTED_EDGE ( 'NONE', *, *, #16805, .T. ) ;
#21432=AXIS2_PLACEMENT_3D ( 'NONE', #8729, #19050, #12163 ) ;
#21437=ORIENTED_EDGE ( 'NONE', *, *, #15894, .F. ) ;
#21441=EDGE_CURVE ( 'NONE', #15404, #13475, #8314, .T. ) ;
#21443=CARTESIAN_POINT ( 'NONE',  ( 24.65063509461090518, 12.50000000000006750, 2.999999999999995559 ) ) ;
#21450=AXIS2_PLACEMENT_3D ( 'NONE', #12116, #20597, #5027 ) ;
#21454=CARTESIAN_POINT ( 'NONE',  ( -25.34312177887347417, 20.17230487860832611, 3.000000000000006217 ) ) ;
#21458=ADVANCED_FACE ( 'NONE', ( #11446 ), #18433, .F. ) ;
#21459=ORIENTED_EDGE ( 'NONE', *, *, #5227, .F. ) ;
#21461=CARTESIAN_POINT ( 'NONE',  ( 20.00000000000004974, -2.506448799221099482E-14, 2.999999999999995559 ) ) ;
#21466=CARTESIAN_POINT ( 'NONE',  ( 13.83143812983136911, -29.36548507648045714, -2.999999999999971578 ) ) ;
#21473=DIRECTION ( 'NONE',  ( 6.505213034913038160E-19, 3.903127820947822896E-18, 1.000000000000000000 ) ) ;
#21481=AXIS2_PLACEMENT_3D ( 'NONE', #11576, #18788, #18564 ) ;
#21482=ORIENTED_EDGE ( 'NONE', *, *, #6945, .F. ) ;
#21485=EDGE_LOOP ( 'NONE', ( #22352, #2068, #21831, #20661 ) ) ;
#21488=CARTESIAN_POINT ( 'NONE',  ( 23.74488952252792728, -25.58633464742643326, 2.999999999999999112 ) ) ;
#21489=EDGE_CURVE ( 'NONE', #19293, #12403, #2834, .T. ) ;
#21490=ORIENTED_EDGE ( 'NONE', *, *, #8090, .T. ) ;
#21493=AXIS2_PLACEMENT_3D ( 'NONE', #13893, #20908, #4281 ) ;
#21496=VECTOR ( 'NONE', #4062, 1000.000000000000000 ) ;
#21498=EDGE_CURVE ( 'NONE', #2350, #4971, #15627, .T. ) ;
#21500=EDGE_CURVE ( 'NONE', #11128, #16827, #16490, .T. ) ;
#21501=CIRCLE ( 'NONE', #10131, 36.76383501243555685 ) ;
#21503=CARTESIAN_POINT ( 'NONE',  ( -28.06260833510301822, 14.30873905802315704, -6.999999999999950262 ) ) ;
#21506=CIRCLE ( 'NONE', #12699, 1.000000000000000888 ) ;
#21507=DIRECTION ( 'NONE',  ( 6.505213034913038160E-19, 3.903127820947822896E-18, 1.000000000000000000 ) ) ;
#21509=ORIENTED_EDGE ( 'NONE', *, *, #13711, .F. ) ;
#21510=AXIS2_PLACEMENT_3D ( 'NONE', #20506, #13038, #18220 ) ;
#21511=ORIENTED_EDGE ( 'NONE', *, *, #9181, .T. ) ;
#21514=ORIENTED_EDGE ( 'NONE', *, *, #3105, .F. ) ;
#21525=AXIS2_PLACEMENT_3D ( 'NONE', #10910, #2213, #9316 ) ;
#21526=ORIENTED_EDGE ( 'NONE', *, *, #13368, .T. ) ;
#21528=CARTESIAN_POINT ( 'NONE',  ( -22.15900668633764781, -29.33526866242125308, -1.999999999999980904 ) ) ;
#21533=EDGE_CURVE ( 'NONE', #66, #19404, #20408, .T. ) ;
#21534=VERTEX_POINT ( 'NONE', #8573 ) ;
#21535=DIRECTION ( 'NONE',  ( 6.505213034913038160E-19, 3.903127820947822896E-18, 1.000000000000000000 ) ) ;
#21536=DIRECTION ( 'NONE',  ( 1.000000000000000000, 2.269002777743560714E-17, 0.000000000000000000 ) ) ;
#21538=CIRCLE ( 'NONE', #1420, 1.000000000000000888 ) ;
#21539=EDGE_CURVE ( 'NONE', #11046, #9968, #1742, .T. ) ;
#21540=B_SPLINE_CURVE_WITH_KNOTS ( 'NONE', 3,
 ( #7222, #5733, #14542, #14191 ),
 .UNSPECIFIED., .F., .F.,
 ( 4, 4 ),
 ( 9.715086407228946956E-07, 0.001929643240672380446 ),
 .UNSPECIFIED. ) ;
#21547=ORIENTED_EDGE ( 'NONE', *, *, #12380, .F. ) ;
#21557=FACE_OUTER_BOUND ( 'NONE', #10866, .T. ) ;
#21558=DIRECTION ( 'NONE',  ( 6.505213034913038160E-19, 3.903127820947822896E-18, 1.000000000000000000 ) ) ;
#21564=EDGE_CURVE ( 'NONE', #13818, #18812, #6495, .T. ) ;
#21567=DIRECTION ( 'NONE',  ( -6.505213034913038160E-19, -3.903127820947822896E-18, -1.000000000000000000 ) ) ;
#21569=ADVANCED_FACE ( 'NONE', ( #18892 ), #10167, .T. ) ;
#21572=AXIS2_PLACEMENT_3D ( 'NONE', #17122, #8532, #22529 ) ;
#21574=EDGE_CURVE ( 'NONE', #43, #11353, #10500, .T. ) ;
#21577=DIRECTION ( 'NONE',  ( -6.505213034913038160E-19, -3.903127820947822896E-18, -1.000000000000000000 ) ) ;
#21579=DIRECTION ( 'NONE',  ( 6.505213034913038160E-19, 3.903127820947822896E-18, 1.000000000000000000 ) ) ;
#21596=AXIS2_PLACEMENT_3D ( 'NONE', #10567, #17566, #9313 ) ;
#21605=CYLINDRICAL_SURFACE ( 'NONE', #11442, 1.000000000000000888 ) ;
#21610=CARTESIAN_POINT ( 'NONE',  ( -35.99819890246949683, 7.463862311151203244, -2.800654218530485018 ) ) ;
#21612=EDGE_CURVE ( 'NONE', #15098, #13932, #11633, .T. ) ;
#21615=DIRECTION ( 'NONE',  ( -6.505213034913038160E-19, -3.903127820947822896E-18, -1.000000000000000000 ) ) ;
#21616=DIRECTION ( 'NONE',  ( -6.505213034913038160E-19, -3.903127820947822896E-18, -1.000000000000000000 ) ) ;
#21622=DIRECTION ( 'NONE',  ( 6.505213034913038160E-19, 3.903127820947822896E-18, 1.000000000000000000 ) ) ;
#21625=VECTOR ( 'NONE', #4535, 1000.000000000000000 ) ;
#21627=EDGE_CURVE ( 'NONE', #14890, #4617, #13807, .T. ) ;
#21636=CIRCLE ( 'NONE', #21278, 19.11328065563151668 ) ;
#21640=CARTESIAN_POINT ( 'NONE',  ( 3.330669073875469621E-13, -1.110223024625156540E-13, -2.999999999999971578 ) ) ;
#21641=CARTESIAN_POINT ( 'NONE',  ( 2.220446049250313081E-13, 2.775557561562891351E-14, -2.800654218530485018 ) ) ;
#21642=ORIENTED_EDGE ( 'NONE', *, *, #9506, .F. ) ;
#21647=DIRECTION ( 'NONE',  ( -1.000000000000000000, 0.000000000000000000, 0.000000000000000000 ) ) ;
#21649=EDGE_CURVE ( 'NONE', #16333, #11887, #15262, .T. ) ;
#21660=CYLINDRICAL_SURFACE ( 'NONE', #16563, 31.50000000000000711 ) ;
#21661=DIRECTION ( 'NONE',  ( 6.505213034913038160E-19, 3.903127820947822896E-18, 1.000000000000000000 ) ) ;
#21662=ORIENTED_EDGE ( 'NONE', *, *, #12062, .F. ) ;
#21665=LINE ( 'NONE', #2298, #3377 ) ;
#21668=CARTESIAN_POINT ( 'NONE',  ( -0.8615617109686474206, -36.14854559161353365, -2.932164912090525988 ) ) ;
#21670=ORIENTED_EDGE ( 'NONE', *, *, #21039, .T. ) ;
#21672=FACE_OUTER_BOUND ( 'NONE', #3785, .T. ) ;
#21679=ORIENTED_EDGE ( 'NONE', *, *, #1766, .T. ) ;
#21681=FACE_OUTER_BOUND ( 'NONE', #4185, .T. ) ;
#21683=CIRCLE ( 'NONE', #4486, 1.000000000000000888 ) ;
#21684=CARTESIAN_POINT ( 'NONE',  ( 2.775557561562891351E-14, -2.775557561562891351E-14, 2.999999999999999112 ) ) ;
#21685=EDGE_CURVE ( 'NONE', #18617, #19759, #9807, .T. ) ;
#21687=DIRECTION ( 'NONE',  ( 1.000000000000000000, 0.000000000000000000, 0.000000000000000000 ) ) ;
#21692=CARTESIAN_POINT ( 'NONE',  ( 7.711478842616664942, -31.57187188083537777, 2.999999999999995559 ) ) ;
#21694=CARTESIAN_POINT ( 'NONE',  ( -26.79308242454876776, -16.56444186175096078, -2.999999999999971578 ) ) ;
#21695=CARTESIAN_POINT ( 'NONE',  ( -36.14854559161338443, 0.8615617109687877528, -2.932164912090540199 ) ) ;
#21702=LINE ( 'NONE', #4405, #5654 ) ;
#21712=ORIENTED_EDGE ( 'NONE', *, *, #251, .T. ) ;
#21713=VERTEX_POINT ( 'NONE', #10726 ) ;
#21715=LINE ( 'NONE', #2697, #6687 ) ;
#21718=VERTEX_POINT ( 'NONE', #17845 ) ;
#21719=CARTESIAN_POINT ( 'NONE',  ( -16.56444186175071209, 26.79308242454869671, 3.000000000000009770 ) ) ;
#21723=LINE ( 'NONE', #15391, #3886 ) ;
#21727=DIRECTION ( 'NONE',  ( -6.505213034913038160E-19, -3.903127820947822896E-18, -1.000000000000000000 ) ) ;
#21730=ADVANCED_FACE ( 'NONE', ( #5477 ), #17729, .T. ) ;
#21734=ORIENTED_EDGE ( 'NONE', *, *, #17048, .F. ) ;
#21735=EDGE_CURVE ( 'NONE', #5940, #1508, #3929, .T. ) ;
#21736=EDGE_CURVE ( 'NONE', #2079, #8181, #16001, .T. ) ;
#21741=ORIENTED_EDGE ( 'NONE', *, *, #7897, .T. ) ;
#21747=DIRECTION ( 'NONE',  ( 6.505213034913038160E-19, 3.903127820947822896E-18, 1.000000000000000000 ) ) ;
#21751=CARTESIAN_POINT ( 'NONE',  ( 11.35354668330729133, 30.33632613426176405, -2.999999999999978240 ) ) ;
#21757=DIRECTION ( 'NONE',  ( -6.505213034913038160E-19, -3.903127820947822896E-18, -1.000000000000000000 ) ) ;
#21759=DIRECTION ( 'NONE',  ( -1.000000000000000000, -1.208970125616060717E-17, 0.000000000000000000 ) ) ;
#21764=DIRECTION ( 'NONE',  ( 1.000000000000000000, 1.208970125616063028E-17, 0.000000000000000000 ) ) ;
#21766=AXIS2_PLACEMENT_3D ( 'NONE', #6178, #6620, #6397 ) ;
#21769=CARTESIAN_POINT ( 'NONE',  ( 33.47097213929444592, -11.93830856187230971, 3.000000000000051514 ) ) ;
#21771=ORIENTED_EDGE ( 'NONE', *, *, #8351, .T. ) ;
#21777=CIRCLE ( 'NONE', #17018, 19.11328065563150957 ) ;
#21779=CYLINDRICAL_SURFACE ( 'NONE', #19584, 19.11328065563150957 ) ;
#21783=TOROIDAL_SURFACE ( 'NONE', #12560, 34.90673715956759082, 8.750000000000000000 ) ;
#21784=PLANE ( 'NONE',  #16244 ) ;
#21785=ADVANCED_FACE ( 'NONE', ( #14387 ), #17102, .T. ) ;
#21789=AXIS2_PLACEMENT_3D ( 'NONE', #17201, #17088, #13410 ) ;
#21794=CIRCLE ( 'NONE', #3133, 34.90673715956759082 ) ;
#21795=ORIENTED_EDGE ( 'NONE', *, *, #12837, .T. ) ;
#21797=ORIENTED_EDGE ( 'NONE', *, *, #21889, .F. ) ;
#21798=CIRCLE ( 'NONE', #15975, 1.000000000000000888 ) ;
#21807=FACE_OUTER_BOUND ( 'NONE', #4259, .T. ) ;
#21809=DIRECTION ( 'NONE',  ( 6.505213034913038160E-19, 3.903127820947822896E-18, 1.000000000000000000 ) ) ;
#21818=VECTOR ( 'NONE', #18755, 1000.000000000000000 ) ;
#21821=CIRCLE ( 'NONE', #17035, 36.76383501243555685 ) ;
#21822=ADVANCED_FACE ( 'NONE', ( #11419 ), #2499, .T. ) ;
#21824=EDGE_LOOP ( 'NONE', ( #10538, #11698, #11596, #21035 ) ) ;
#21825=CARTESIAN_POINT ( 'NONE',  ( 21.41958700883258970, 27.56232195404059837, 3.000000000000002665 ) ) ;
#21826=DIRECTION ( 'NONE',  ( 6.505213034913038160E-19, 3.903127820947822896E-18, 1.000000000000000000 ) ) ;
#21828=AXIS2_PLACEMENT_3D ( 'NONE', #17633, #335, #3779 ) ;
#21829=EDGE_CURVE ( 'NONE', #5003, #20565, #16746, .T. ) ;
#21831=ORIENTED_EDGE ( 'NONE', *, *, #688, .T. ) ;
#21832=ORIENTED_EDGE ( 'NONE', *, *, #11528, .F. ) ;
#21836=AXIS2_PLACEMENT_3D ( 'NONE', #18066, #4337, #18530 ) ;
#21837=CIRCLE ( 'NONE', #6466, 19.11328065563152379 ) ;
#21839=DIRECTION ( 'NONE',  ( -1.000000000000000000, -1.208970125616077665E-17, 0.000000000000000000 ) ) ;
#21841=AXIS2_PLACEMENT_3D ( 'NONE', #6989, #9037, #13945 ) ;
#21848=DIRECTION ( 'NONE',  ( -6.505213034913038160E-19, -3.903127820947822896E-18, -1.000000000000000000 ) ) ;
#21850=CARTESIAN_POINT ( 'NONE',  ( -12.31876324338268525, -30.07487443287973505, 2.999999999999995559 ) ) ;
#21864=AXIS2_PLACEMENT_3D ( 'NONE', #1584, #4915, #15088 ) ;
#21866=DIRECTION ( 'NONE',  ( 1.000000000000000000, 0.000000000000000000, 0.000000000000000000 ) ) ;
#21870=DIRECTION ( 'NONE',  ( -1.000000000000000000, -1.208970125616063182E-17, 0.000000000000000000 ) ) ;
#21873=AXIS2_PLACEMENT_3D ( 'NONE', #1846, #14187, #15798 ) ;
#21878=ORIENTED_EDGE ( 'NONE', *, *, #17742, .F. ) ;
#21880=CYLINDRICAL_SURFACE ( 'NONE', #21766, 1.000000000000000888 ) ;
#21881=CARTESIAN_POINT ( 'NONE',  ( 30.13956425491254265, 21.05198877411773495, 2.800654218530485018 ) ) ;
#21884=CIRCLE ( 'NONE', #10144, 1.000000000000000888 ) ;
#21885=ORIENTED_EDGE ( 'NONE', *, *, #10376, .T. ) ;
#21888=CARTESIAN_POINT ( 'NONE',  ( -32.14641817400170964, -18.83615802559815577, -2.999999999999971578 ) ) ;
#21889=EDGE_CURVE ( 'NONE', #12492, #17781, #21884, .T. ) ;
#21902=ORIENTED_EDGE ( 'NONE', *, *, #18741, .T. ) ;
#21904=FACE_OUTER_BOUND ( 'NONE', #15512, .T. ) ;
#21907=VECTOR ( 'NONE', #10072, 1000.000000000000000 ) ;
#21911=AXIS2_PLACEMENT_3D ( 'NONE', #20914, #21023, #1779 ) ;
#21912=ADVANCED_FACE ( 'NONE', ( #19691 ), #13128, .F. ) ;
#21924=DIRECTION ( 'NONE',  ( -6.505213034913038160E-19, -3.903127820947822896E-18, -1.000000000000000000 ) ) ;
#21927=CYLINDRICAL_SURFACE ( 'NONE', #4670, 36.76383501243555685 ) ;
#21929=ORIENTED_EDGE ( 'NONE', *, *, #12037, .T. ) ;
#21934=CARTESIAN_POINT ( 'NONE',  ( -2.422192751863727622, -32.40961249803553557, 3.000000000000023537 ) ) ;
#21944=CARTESIAN_POINT ( 'NONE',  ( -9.999999999999758415, -3.000000000000169198, -4.999999999999984013 ) ) ;
#21948=CIRCLE ( 'NONE', #4736, 1.000000000000001776 ) ;
#21953=ORIENTED_EDGE ( 'NONE', *, *, #15400, .T. ) ;
#21959=DIRECTION ( 'NONE',  ( 1.000000000000000000, 1.208970125616063182E-17, 0.000000000000000000 ) ) ;
#21961=DIRECTION ( 'NONE',  ( 1.000000000000000000, -7.981516076044952263E-15, 0.000000000000000000 ) ) ;
#21962=EDGE_CURVE ( 'NONE', #5560, #22077, #18973, .T. ) ;
#21963=AXIS2_PLACEMENT_3D ( 'NONE', #11325, #16479, #10979 ) ;
#21964=EDGE_LOOP ( 'NONE', ( #2865, #4171, #8409, #2608, #9169, #1267 ) ) ;
#21966=EDGE_CURVE ( 'NONE', #5340, #15747, #15661, .T. ) ;
#21973=DIRECTION ( 'NONE',  ( -6.505213034913038160E-19, -3.903127820947822896E-18, -1.000000000000000000 ) ) ;
#21979=CARTESIAN_POINT ( 'NONE',  ( 34.74700806321118307, -12.00937115242659026, -2.000000000000001776 ) ) ;
#21992=CARTESIAN_POINT ( 'NONE',  ( 3.330669073875469621E-13, -1.110223024625156540E-13, -2.999999999999971578 ) ) ;
#21996=CYLINDRICAL_SURFACE ( 'NONE', #20366, 19.11328065563152379 ) ;
#21998=DIRECTION ( 'NONE',  ( -1.000000000000000000, -1.208970125616044077E-17, 0.000000000000000000 ) ) ;
#21999=ADVANCED_FACE ( 'NONE', ( #13570 ), #4672, .T. ) ;
#22003=DIRECTION ( 'NONE',  ( 6.505213034913038160E-19, 3.903127820947822896E-18, 1.000000000000000000 ) ) ;
#22005=CARTESIAN_POINT ( 'NONE',  ( 2.775557561562891351E-14, -2.775557561562891351E-14, 2.999999999999999112 ) ) ;
#22008=EDGE_LOOP ( 'NONE', ( #10041, #10992, #11000, #509, #10796, #20642 ) ) ;
#22010=FACE_OUTER_BOUND ( 'NONE', #5550, .T. ) ;
#22013=ORIENTED_EDGE ( 'NONE', *, *, #11273, .T. ) ;
#22015=DIRECTION ( 'NONE',  ( -6.505213034913038160E-19, -3.903127820947822896E-18, -1.000000000000000000 ) ) ;
#22018=CIRCLE ( 'NONE', #15401, 34.90673715956759082 ) ;
#22019=PRODUCT_DEFINITION ( 'UNKNOWN', '', #15689, #12542 ) ;
#22021=ADVANCED_FACE ( 'NONE', ( #4893 ), #16810, .F. ) ;
#22023=ORIENTED_EDGE ( 'NONE', *, *, #1400, .F. ) ;
#22026=DIRECTION ( 'NONE',  ( 6.505213034913038160E-19, 3.903127820947822896E-18, 1.000000000000000000 ) ) ;
#22029=ORIENTED_EDGE ( 'NONE', *, *, #12441, .T. ) ;
#22035=CARTESIAN_POINT ( 'NONE',  ( 22.15900668633799597, 29.33526866242080899, -2.800654218530477912 ) ) ;
#22042=ORIENTED_EDGE ( 'NONE', *, *, #16066, .F. ) ;
#22045=ORIENTED_EDGE ( 'NONE', *, *, #20210, .F. ) ;
#22053=CIRCLE ( 'NONE', #16166, 1.000000000000000888 ) ;
#22056=VERTEX_POINT ( 'NONE', #6957 ) ;
#22058=DIRECTION ( 'NONE',  ( -1.000000000000000000, 0.000000000000000000, 0.000000000000000000 ) ) ;
#22060=DIRECTION ( 'NONE',  ( -1.000000000000000000, 1.775147869274631246E-14, 0.000000000000000000 ) ) ;
#22065=ADVANCED_FACE ( 'NONE', ( #3639 ), #5799, .T. ) ;
#22066=EDGE_LOOP ( 'NONE', ( #10563, #17387, #15646, #10812, #18337, #6757, #396, #7973, #7050, #489, #6960, #17329, #19468, #3290, #7016, #17590, #17417, #15179, #9875, #5086, #2925, #1577, #19060, #16282, #13486, #1189, #13093, #21514, #1477, #18835, #16897, #13960, #19950, #10733, #8211, #21662, #16832, #15036, #4441, #6778, #2164, #8954, #148, #17784, #21349, #80, #3172, #5001, #7586, #4417, #5081, #7852, #10121, #5548, #1172, #17218, #17817, #1944, #11254, #11358, #5363, #7697, #8590, #15273, #12973, #5382, #14489, #18397, #21322, #13441, #13931, #21313, #16852, #13295, #2589, #8148, #17971, #18694, #14835, #12406, #8161, #4600, #19515, #6230, #2510, #4194, #20664, #20785, #1156, #21509, #20900, #19849, #19852, #11144, #10658, #13236, #11590, #20457, #2256, #4902, #758, #7824, #13977, #4165, #1721, #8206, #1462, #13109, #18936, #3123, #9530, #18312, #14549, #7022, #8433, #3344, #3629, #20906, #11823, #19495, #17926, #7154, #2446, #19630, #18378, #20878, #21797, #16135, #2986, #18141, #17931 ) ) ;
#22068=CYLINDRICAL_SURFACE ( 'NONE', #14182, 36.76383501243555685 ) ;
#22070=CARTESIAN_POINT ( 'NONE',  ( 2.775557561562891351E-14, -2.775557561562891351E-14, 2.999999999999999112 ) ) ;
#22071=AXIS2_PLACEMENT_3D ( 'NONE', #2531, #9403, #1029 ) ;
#22072=AXIS2_PLACEMENT_3D ( 'NONE', #17333, #12179, #7024 ) ;
#22073=EDGE_CURVE ( 'NONE', #16550, #18180, #7243, .T. ) ;
#22076=CARTESIAN_POINT ( 'NONE',  ( -7.980461308159936706, 36.39375341857520141, -2.999999999999999112 ) ) ;
#22077=VERTEX_POINT ( 'NONE', #5231 ) ;
#22078=ORIENTED_EDGE ( 'NONE', *, *, #9735, .T. ) ;
#22087=CARTESIAN_POINT ( 'NONE',  ( 2.775557561562891351E-14, 2.775557561562891351E-14, 5.750000000000001776 ) ) ;
#22088=CIRCLE ( 'NONE', #12916, 1.000000000000000888 ) ;
#22097=CARTESIAN_POINT ( 'NONE',  ( -24.73600648735116536, 27.19760187735834123, -1.999999999999977573 ) ) ;
#22098=LINE ( 'NONE', #8225, #7868 ) ;
#22099=ORIENTED_EDGE ( 'NONE', *, *, #8746, .F. ) ;
#22103=DIRECTION ( 'NONE',  ( 6.505213034913038160E-19, 3.903127820947822896E-18, 1.000000000000000000 ) ) ;
#22104=DIRECTION ( 'NONE',  ( -1.000000000000000000, -1.208970125616063644E-17, 0.000000000000000000 ) ) ;
#22106=CIRCLE ( 'NONE', #12554, 31.50000000000001421 ) ;
#22110=VERTEX_POINT ( 'NONE', #19441 ) ;
#22112=ADVANCED_FACE ( 'NONE', ( #21041 ), #7054, .T. ) ;
#22113=DIRECTION ( 'NONE',  ( 6.505213034913038160E-19, 3.903127820947822896E-18, 1.000000000000000000 ) ) ;
#22114=VERTEX_POINT ( 'NONE', #12101 ) ;
#22115=DIRECTION ( 'NONE',  ( -1.000000000000000000, -1.208970125616063644E-17, 0.000000000000000000 ) ) ;
#22116=DIRECTION ( 'NONE',  ( 6.505213034913038160E-19, 3.903127820947822896E-18, 1.000000000000000000 ) ) ;
#22118=AXIS2_PLACEMENT_3D ( 'NONE', #2877, #2762, #22240 ) ;
#22119=LINE ( 'NONE', #18443, #5677 ) ;
#22120=DIRECTION ( 'NONE',  ( -6.505213034913038160E-19, -3.903127820947822896E-18, -1.000000000000000000 ) ) ;
#22121=ORIENTED_EDGE ( 'NONE', *, *, #2948, .T. ) ;
#22122=DIRECTION ( 'NONE',  ( 1.000000000000000000, 0.000000000000000000, 0.000000000000000000 ) ) ;
#22125=FACE_OUTER_BOUND ( 'NONE', #473, .T. ) ;
#22126=ORIENTED_EDGE ( 'NONE', *, *, #2163, .F. ) ;
#22133=EDGE_LOOP ( 'NONE', ( #5059, #19071, #7470, #8223 ) ) ;
#22134=VERTEX_POINT ( 'NONE', #1681 ) ;
#22136=ORIENTED_EDGE ( 'NONE', *, *, #7114, .T. ) ;
#22141=CIRCLE ( 'NONE', #13330, 19.11328065563152379 ) ;
#22142=DIRECTION ( 'NONE',  ( -1.000000000000000000, -1.208970125616060101E-17, 6.505213034913038160E-19 ) ) ;
#22145=CARTESIAN_POINT ( 'NONE',  ( 31.41173278719269746, 17.66631876130919565, 2.999999999999999112 ) ) ;
#22146=ORIENTED_EDGE ( 'NONE', *, *, #6306, .F. ) ;
#22148=EDGE_CURVE ( 'NONE', #2722, #20782, #6892, .T. ) ;
#22150=CARTESIAN_POINT ( 'NONE',  ( -10.00000000000000888, 2.999999999999836131, -4.999999999999948486 ) ) ;
#22151=CARTESIAN_POINT ( 'NONE',  ( 4.025500340002596822, -36.54278193890326065, -2.000000000000005329 ) ) ;
#22152=VERTEX_POINT ( 'NONE', #12212 ) ;
#22154=EDGE_LOOP ( 'NONE', ( #6851, #20784, #19350, #8046 ) ) ;
#22157=CARTESIAN_POINT ( 'NONE',  ( -24.75236754129142724, -27.84804035626034491, -6.999999999999999112 ) ) ;
#22159=PLANE ( 'NONE',  #6053 ) ;
#22160=DIRECTION ( 'NONE',  ( 1.000000000000000000, 0.000000000000000000, 0.000000000000000000 ) ) ;
#22161=AXIS2_PLACEMENT_3D ( 'NONE', #12195, #8011, #14966 ) ;
#22164=ORIENTED_EDGE ( 'NONE', *, *, #7070, .F. ) ;
#22165=AXIS2_PLACEMENT_3D ( 'NONE', #14514, #19390, #1959 ) ;
#22166=ORIENTED_EDGE ( 'NONE', *, *, #4221, .T. ) ;
#22172=CARTESIAN_POINT ( 'NONE',  ( -5.074925817841801745, 32.10132595304121850, -6.999999999999950262 ) ) ;
#22173=LINE ( 'NONE', #9798, #21625 ) ;
#22175=CIRCLE ( 'NONE', #13715, 2.999999999999999112 ) ;
#22181=ORIENTED_EDGE ( 'NONE', *, *, #19252, .T. ) ;
#22183=AXIS2_PLACEMENT_3D ( 'NONE', #14291, #15685, #21192 ) ;
#22185=DIRECTION ( 'NONE',  ( -1.000000000000000000, 1.243413522203471269E-14, 0.000000000000000000 ) ) ;
#22191=CIRCLE ( 'NONE', #19260, 34.90673715956759082 ) ;
#22203=EDGE_CURVE ( 'NONE', #12412, #10093, #294, .T. ) ;
#22204=FACE_OUTER_BOUND ( 'NONE', #12147, .T. ) ;
#22206=DIRECTION ( 'NONE',  ( -1.000000000000000000, -1.208970125616044077E-17, 0.000000000000000000 ) ) ;
#22208=DIRECTION ( 'NONE',  ( 1.000000000000000000, 0.000000000000000000, 0.000000000000000000 ) ) ;
#22209=AXIS2_PLACEMENT_3D ( 'NONE', #18226, #11226, #16616 ) ;
#22210=VERTEX_POINT ( 'NONE', #14134 ) ;
#22214=VECTOR ( 'NONE', #766, 1000.000000000000000 ) ;
#22215=ORIENTED_EDGE ( 'NONE', *, *, #14202, .T. ) ;
#22216=LINE ( 'NONE', #8452, #3609 ) ;
#22222=ADVANCED_FACE ( 'NONE', ( #17705 ), #15012, .F. ) ;
#22223=CIRCLE ( 'NONE', #22239, 19.11328065563151668 ) ;
#22228=ORIENTED_EDGE ( 'NONE', *, *, #2140, .T. ) ;
#22231=DIRECTION ( 'NONE',  ( -1.000000000000000000, 0.000000000000000000, 0.000000000000000000 ) ) ;
#22233=ADVANCED_FACE ( 'NONE', ( #21807 ), #11644, .T. ) ;
#22235=CIRCLE ( 'NONE', #10872, 31.50000000000001421 ) ;
#22237=VERTEX_POINT ( 'NONE', #9646 ) ;
#22239=AXIS2_PLACEMENT_3D ( 'NONE', #8389, #22608, #11930 ) ;
#22240=DIRECTION ( 'NONE',  ( 1.000000000000000000, 1.208970125616053321E-17, 0.000000000000000000 ) ) ;
#22242=CARTESIAN_POINT ( 'NONE',  ( 35.29097153256788744, 4.153395668489309855, -2.999999999999986677 ) ) ;
#22244=ORIENTED_EDGE ( 'NONE', *, *, #20258, .T. ) ;
#22245=DIRECTION ( 'NONE',  ( -1.000000000000000000, 0.000000000000000000, 0.000000000000000000 ) ) ;
#22260=ORIENTED_EDGE ( 'NONE', *, *, #8351, .F. ) ;
#22261=FACE_OUTER_BOUND ( 'NONE', #19887, .T. ) ;
#22267=CARTESIAN_POINT ( 'NONE',  ( -14.74639653023206165, 28.96193690644924246, -2.999999999999968026 ) ) ;
#22270=CARTESIAN_POINT ( 'NONE',  ( 35.52192638951989068, -1.010906942018348520, 3.000000000000051514 ) ) ;
#22271=AXIS2_PLACEMENT_3D ( 'NONE', #18914, #3223, #16543 ) ;
#22272=VERTEX_POINT ( 'NONE', #18700 ) ;
#22282=CARTESIAN_POINT ( 'NONE',  ( 2.220446049250313081E-13, 2.775557561562891351E-14, -2.800654218530485018 ) ) ;
#22287=B_SPLINE_CURVE_WITH_KNOTS ( 'NONE', 3,
 ( #461, #18334, #11349, #2650 ),
 .UNSPECIFIED., .F., .F.,
 ( 4, 4 ),
 ( 9.545285769853128040E-07, 0.001900595205834734389 ),
 .UNSPECIFIED. ) ;
#22289=AXIS2_PLACEMENT_3D ( 'NONE', #2244, #14490, #3857 ) ;
#22293=ORIENTED_EDGE ( 'NONE', *, *, #8400, .F. ) ;
#22296=LINE ( 'NONE', #11513, #1230 ) ;
#22302=ORIENTED_EDGE ( 'NONE', *, *, #20251, .T. ) ;
#22304=DIRECTION ( 'NONE',  ( 6.505213034913038160E-19, 3.903127820947822896E-18, 1.000000000000000000 ) ) ;
#22321=EDGE_CURVE ( 'NONE', #15970, #11834, #12010, .T. ) ;
#22322=FACE_OUTER_BOUND ( 'NONE', #20048, .T. ) ;
#22323=DIRECTION ( 'NONE',  ( -1.000000000000000000, -1.208970125616044077E-17, 0.000000000000000000 ) ) ;
#22330=DIRECTION ( 'NONE',  ( 6.505213034913038160E-19, 3.903127820947822896E-18, 1.000000000000000000 ) ) ;
#22332=ORIENTED_EDGE ( 'NONE', *, *, #2612, .F. ) ;
#22343=DIRECTION ( 'NONE',  ( -1.000000000000000000, -1.208970125616063644E-17, 0.000000000000000000 ) ) ;
#22345=FACE_OUTER_BOUND ( 'NONE', #16238, .T. ) ;
#22346=DIRECTION ( 'NONE',  ( 1.000000000000000000, 0.000000000000000000, 0.000000000000000000 ) ) ;
#22347=CARTESIAN_POINT ( 'NONE',  ( 10.34893680499437707, -34.64233806479136035, 2.932969818539088003 ) ) ;
#22349=CARTESIAN_POINT ( 'NONE',  ( -4.080045426412826082, 32.20238537491812281, -6.999999999999999112 ) ) ;
#22352=ORIENTED_EDGE ( 'NONE', *, *, #12378, .T. ) ;
#22357=EDGE_LOOP ( 'NONE', ( #9825, #19489, #4607, #8432 ) ) ;
#22359=DIRECTION ( 'NONE',  ( 6.505213034913038160E-19, 3.903127820947822896E-18, 1.000000000000000000 ) ) ;
#22365=VERTEX_POINT ( 'NONE', #3113 ) ;
#22366=EDGE_CURVE ( 'NONE', #11842, #1931, #15294, .T. ) ;
#22370=DIRECTION ( 'NONE',  ( -1.000000000000000000, 0.000000000000000000, 0.000000000000000000 ) ) ;
#22376=CARTESIAN_POINT ( 'NONE',  ( -23.74488952252773544, 25.58633464742632313, 3.000000000000023537 ) ) ;
#22382=DIRECTION ( 'NONE',  ( 6.505213034913038160E-19, 3.903127820947822896E-18, 1.000000000000000000 ) ) ;
#22386=CARTESIAN_POINT ( 'NONE',  ( -32.83234229683721850, 11.85401191286866762, -2.999999999999971578 ) ) ;
#22389=DIRECTION ( 'NONE',  ( 1.000000000000000000, 0.000000000000000000, 0.000000000000000000 ) ) ;
#22391=DIRECTION ( 'NONE',  ( -6.505213034913038160E-19, -3.903127820947822896E-18, -1.000000000000000000 ) ) ;
#22400=CARTESIAN_POINT ( 'NONE',  ( 11.35354668330712613, 30.33632613426179248, -6.999999999999985789 ) ) ;
#22407=EDGE_LOOP ( 'NONE', ( #7345, #14385, #18919, #10568 ) ) ;
#22409=DIRECTION ( 'NONE',  ( 6.505213034913038160E-19, 3.903127820947822896E-18, 1.000000000000000000 ) ) ;
#22410=CARTESIAN_POINT ( 'NONE',  ( 34.11307262910447236, -11.98990878915382119, -2.932164912090505560 ) ) ;
#22419=VERTEX_POINT ( 'NONE', #13740 ) ;
#22421=DIRECTION ( 'NONE',  ( -1.000000000000000000, -1.208970125616077665E-17, 0.000000000000000000 ) ) ;
#22433=EDGE_CURVE ( 'NONE', #15811, #5732, #20980, .T. ) ;
#22435=DIRECTION ( 'NONE',  ( -1.000000000000000000, -1.208970125616077665E-17, 0.000000000000000000 ) ) ;
#22437=EDGE_CURVE ( 'NONE', #12610, #8443, #6918, .T. ) ;
#22439=CARTESIAN_POINT ( 'NONE',  ( -4.080045426412826082, 32.20238537491803754, -2.999999999999971578 ) ) ;
#22440=EDGE_CURVE ( 'NONE', #4768, #13346, #1619, .T. ) ;
#22441=DIRECTION ( 'NONE',  ( -1.000000000000000000, -1.208970125616081209E-17, 0.000000000000000000 ) ) ;
#22443=DIRECTION ( 'NONE',  ( 6.505213034913038160E-19, 3.903127820947822896E-18, 1.000000000000000000 ) ) ;
#22444=ORIENTED_EDGE ( 'NONE', *, *, #19406, .F. ) ;
#22446=VECTOR ( 'NONE', #8782, 1000.000000000000000 ) ;
#22447=AXIS2_PLACEMENT_3D ( 'NONE', #3925, #21567, #9416 ) ;
#22448=ORIENTED_EDGE ( 'NONE', *, *, #15228, .F. ) ;
#22456=CARTESIAN_POINT ( 'NONE',  ( -22.26748298433256679, 22.28024240313483517, 2.999999999999995559 ) ) ;
#22465=B_SPLINE_CURVE_WITH_KNOTS ( 'NONE', 3,
 ( #12697, #7780, #14752, #16132 ),
 .UNSPECIFIED., .F., .F.,
 ( 4, 4 ),
 ( 0.001875451646902692423, 0.003761979286331381712 ),
 .UNSPECIFIED. ) ;
#22466=DIRECTION ( 'NONE',  ( 1.000000000000000000, 2.269002777743560714E-17, 0.000000000000000000 ) ) ;
#22469=EDGE_CURVE ( 'NONE', #12370, #19815, #14183, .T. ) ;
#22470=VERTEX_POINT ( 'NONE', #10201 ) ;
#22479=ORIENTED_EDGE ( 'NONE', *, *, #11783, .T. ) ;
#22480=CARTESIAN_POINT ( 'NONE',  ( 26.50842683089768670, -24.41514043009201984, 2.999999999999995559 ) ) ;
#22481=DIRECTION ( 'NONE',  ( -6.505213034913038160E-19, -3.903127820947822896E-18, -1.000000000000000000 ) ) ;
#22483=CYLINDRICAL_SURFACE ( 'NONE', #7968, 22.00000000000000000 ) ;
#22486=DIRECTION ( 'NONE',  ( 6.505213034913038160E-19, 3.903127820947822896E-18, 1.000000000000000000 ) ) ;
#22487=CARTESIAN_POINT ( 'NONE',  ( 9.708269511265326557, -33.52953626616050542, 3.000000000000002665 ) ) ;
#22491=FACE_OUTER_BOUND ( 'NONE', #19726, .T. ) ;
#22496=DIRECTION ( 'NONE',  ( -6.505213034913038160E-19, -3.903127820947822896E-18, -1.000000000000000000 ) ) ;
#22498=VERTEX_POINT ( 'NONE', #20874 ) ;
#22499=CYLINDRICAL_SURFACE ( 'NONE', #8692, 1.000000000000000888 ) ;
#22500=CARTESIAN_POINT ( 'NONE',  ( -12.00937115242646591, -34.74700806321101254, 2.800654218530512551 ) ) ;
#22513=CARTESIAN_POINT ( 'NONE',  ( -27.56232195404058416, 21.41958700883256483, -2.999999999999971578 ) ) ;
#22528=CARTESIAN_POINT ( 'NONE',  ( 29.32895111104242503, 20.05817253550603851, -2.999999999999993339 ) ) ;
#22529=DIRECTION ( 'NONE',  ( 1.000000000000000000, 0.000000000000000000, 0.000000000000000000 ) ) ;
#22530=ADVANCED_FACE ( 'NONE', ( #10874 ), #5607, .F. ) ;
#22532=DIRECTION ( 'NONE',  ( -6.505213034913038160E-19, -3.903127820947822896E-18, -1.000000000000000000 ) ) ;
#22533=CIRCLE ( 'NONE', #9356, 0.9999999999999974465 ) ;
#22535=EDGE_CURVE ( 'NONE', #16319, #22498, #16261, .T. ) ;
#22537=VERTEX_POINT ( 'NONE', #10752 ) ;
#22540=ORIENTED_EDGE ( 'NONE', *, *, #19694, .T. ) ;
#22541=DIRECTION ( 'NONE',  ( 6.505213034913038160E-19, 3.903127820947822896E-18, 1.000000000000000000 ) ) ;
#22542=DIRECTION ( 'NONE',  ( -1.000000000000000000, -1.208970125616046080E-17, 6.505213034913038160E-19 ) ) ;
#22543=CIRCLE ( 'NONE', #6430, 31.50000000000000711 ) ;
#22551=CARTESIAN_POINT ( 'NONE',  ( -34.90673715956756240, -1.391773526489529182E-13, 2.999999999999999112 ) ) ;
#22555=ORIENTED_EDGE ( 'NONE', *, *, #11553, .F. ) ;
#22556=FACE_OUTER_BOUND ( 'NONE', #12242, .T. ) ;
#22558=VECTOR ( 'NONE', #8495, 1000.000000000000000 ) ;
#22560=EDGE_LOOP ( 'NONE', ( #18155, #16076, #13003, #20312 ) ) ;
#22561=DIRECTION ( 'NONE',  ( 1.000000000000000000, 0.000000000000000000, 0.000000000000000000 ) ) ;
#22566=EDGE_LOOP ( 'NONE', ( #15455, #741, #12834, #7517 ) ) ;
#22567=CIRCLE ( 'NONE', #17780, 34.90673715956759082 ) ;
#22576=ADVANCED_FACE ( 'NONE', ( #450 ), #2288, .F. ) ;
#22582=AXIS2_PLACEMENT_3D ( 'NONE', #19792, #7643, #649 ) ;
#22588=ORIENTED_EDGE ( 'NONE', *, *, #3879, .T. ) ;
#22590=DIRECTION ( 'NONE',  ( 1.000000000000000000, 0.000000000000000000, 0.000000000000000000 ) ) ;
#22591=VECTOR ( 'NONE', #11009, 1000.000000000000000 ) ;
#22592=EDGE_CURVE ( 'NONE', #17930, #11125, #9365, .T. ) ;
#22594=AXIS2_PLACEMENT_3D ( 'NONE', #13073, #16761, #9772 ) ;
#22596=ORIENTED_EDGE ( 'NONE', *, *, #13250, .F. ) ;
#22597=LINE ( 'NONE', #6894, #14296 ) ;
#22598=EDGE_CURVE ( 'NONE', #9329, #4860, #17132, .T. ) ;
#22600=DIRECTION ( 'NONE',  ( -6.505213034913038160E-19, -3.903127820947822896E-18, -1.000000000000000000 ) ) ;
#22605=DIRECTION ( 'NONE',  ( -1.000000000000000000, -1.208970125616060101E-17, 6.505213034913038160E-19 ) ) ;
#22606=LINE ( 'NONE', #5181, #7216 ) ;
#22607=ORIENTED_EDGE ( 'NONE', *, *, #19940, .T. ) ;
#22608=DIRECTION ( 'NONE',  ( -6.505213034913038160E-19, -3.903127820947822896E-18, -1.000000000000000000 ) ) ;
#22614=VERTEX_POINT ( 'NONE', #16137 ) ;
#22615=DIRECTION ( 'NONE',  ( -1.000000000000000000, -1.208970125616081209E-17, 0.000000000000000000 ) ) ;
#22617=ORIENTED_EDGE ( 'NONE', *, *, #8898, .T. ) ;
#22623=CARTESIAN_POINT ( 'NONE',  ( 24.10368028608819913, -26.10969099697642193, -2.999999999999983125 ) ) ;
#22626=VECTOR ( 'NONE', #14986, 1000.000000000000000 ) ;
#22628=ADVANCED_FACE ( 'NONE', ( #17538 ), #2526, .T. ) ;
#22633=ORIENTED_EDGE ( 'NONE', *, *, #6883, .F. ) ;
#22635=DIRECTION ( 'NONE',  ( -6.505213034913038160E-19, -3.903127820947822896E-18, -1.000000000000000000 ) ) ;
#22638=AXIS2_PLACEMENT_3D ( 'NONE', #18290, #7746, #20016 ) ;
#22640=CARTESIAN_POINT ( 'NONE',  ( -20.05817253550612023, 29.32895111104205199, -3.000000000000006661 ) ) ;
#22643=AXIS2_PLACEMENT_3D ( 'NONE', #2321, #9431, #14221 ) ;
#22646=CYLINDRICAL_SURFACE ( 'NONE', #21911, 31.50000000000001421 ) ;
#22650=ADVANCED_FACE ( 'NONE', ( #12815 ), #7677, .F. ) ;
#22656=DIRECTION ( 'NONE',  ( -1.000000000000000000, 1.764267138144086878E-15, 0.000000000000000000 ) ) ;
#22664=AXIS2_PLACEMENT_3D ( 'NONE', #6898, #17078, #13619 ) ;
#22670=DIRECTION ( 'NONE',  ( 6.505213034913038160E-19, 3.903127820947822896E-18, 1.000000000000000000 ) ) ;
#22676=CARTESIAN_POINT ( 'NONE',  ( 2.775557561562891351E-14, -2.775557561562891351E-14, 2.999999999999999112 ) ) ;
#22679=ORIENTED_EDGE ( 'NONE', *, *, #9439, .T. ) ;
#22680=DIRECTION ( 'NONE',  ( 1.000000000000000000, 0.000000000000000000, 0.000000000000000000 ) ) ;
#22682=CYLINDRICAL_SURFACE ( 'NONE', #17847, 1.000000000000000888 ) ;
#22683=CARTESIAN_POINT ( 'NONE',  ( -20.17230487860793886, -25.34312177887360207, 2.999999999999995559 ) ) ;
#22685=DIRECTION ( 'NONE',  ( 6.505213034913038160E-19, 3.903127820947822896E-18, 1.000000000000000000 ) ) ;
#22688=EDGE_CURVE ( 'NONE', #4478, #1089, #8374, .T. ) ;
#22690=FACE_OUTER_BOUND ( 'NONE', #6036, .T. ) ;
#22694=FACE_OUTER_BOUND ( 'NONE', #9815, .T. ) ;
#22695=EDGE_LOOP ( 'NONE', ( #9768, #7752, #22588, #21086 ) ) ;
#22742=COLOUR_RGB('Off White',0.89,0.88,0.83);
#22743=FILL_AREA_STYLE_COLOUR('',#22742);
#22744=FILL_AREA_STYLE('',(#22743));
#22745=SURFACE_STYLE_FILL_AREA(#22744);
#22746=SURFACE_SIDE_STYLE('',(#22745));
#22747=SURFACE_STYLE_USAGE(.BOTH.,#22746);
#22748=PRESENTATION_STYLE_ASSIGNMENT((#22747));
ENDSEC;
END-ISO-10303-21;
